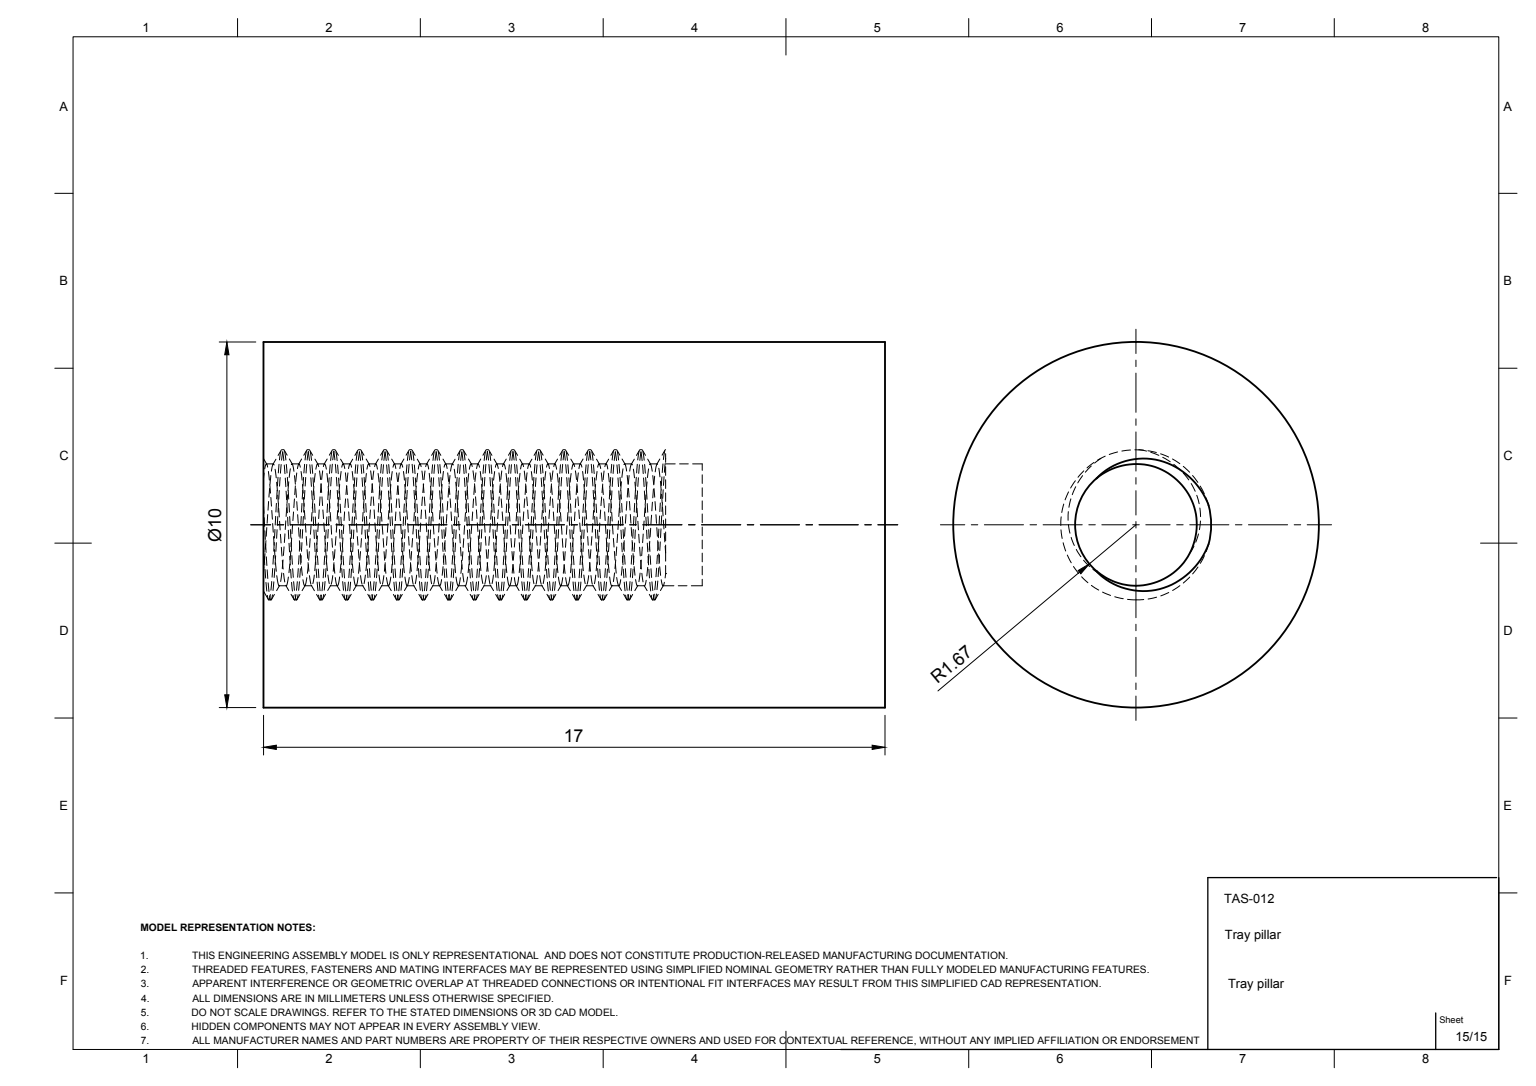
ISO-10303-21;
HEADER;
/* Generated by software containing ST-Developer
 * from STEP Tools, Inc. (www.steptools.com) 
 */

FILE_DESCRIPTION(
/* description */ (
'Independent welded steel electronics enclosure with removable sealed 
lid, internal mounting tray and two threaded cable entries. 300 x 220 
mm body. No ingress or electrical safety rating assigned.'),
/* implementation_level */ '2;1');

FILE_NAME(
/* name */ 'Tray pillar.step',
/* time_stamp */ '2026-11-14T09:13:27-08:00',
/* author */ (''),
/* organization */ (''),
/* preprocessor_version */ 'ST-DEVELOPER v20.2',
/* originating_system */ 'Autodesk Translation Framework v15.17.0.0',
/* authorisation */ '');

FILE_SCHEMA (('AUTOMOTIVE_DESIGN { 1 0 10303 214 3 1 1 }'));
ENDSEC;

DATA;
#10=MECHANICAL_DESIGN_GEOMETRIC_PRESENTATION_REPRESENTATION('',(#972),#94412);
#160=B_SPLINE_SURFACE_WITH_KNOTS('',3,3,((#58672,#58673,#58674,#58675,#58676,
#58677,#58678,#58679,#58680,#58681,#58682,#58683,#58684,#58685,#58686,#58687,
#58688,#58689,#58690,#58691,#58692,#58693,#58694,#58695,#58696,#58697,#58698,
#58699,#58700,#58701,#58702,#58703,#58704,#58705,#58706,#58707,#58708,#58709,
#58710,#58711,#58712,#58713,#58714,#58715,#58716,#58717,#58718,#58719,#58720,
#58721,#58722,#58723,#58724,#58725,#58726,#58727,#58728,#58729,#58730,#58731,
#58732,#58733,#58734,#58735,#58736,#58737,#58738,#58739,#58740,#58741,#58742,
#58743,#58744,#58745,#58746,#58747,#58748,#58749,#58750,#58751,#58752,#58753,
#58754,#58755,#58756,#58757,#58758,#58759,#58760,#58761,#58762,#58763,#58764,
#58765,#58766,#58767,#58768,#58769,#58770,#58771,#58772,#58773,#58774,#58775),
(#58776,#58777,#58778,#58779,#58780,#58781,#58782,#58783,#58784,#58785,
#58786,#58787,#58788,#58789,#58790,#58791,#58792,#58793,#58794,#58795,#58796,
#58797,#58798,#58799,#58800,#58801,#58802,#58803,#58804,#58805,#58806,#58807,
#58808,#58809,#58810,#58811,#58812,#58813,#58814,#58815,#58816,#58817,#58818,
#58819,#58820,#58821,#58822,#58823,#58824,#58825,#58826,#58827,#58828,#58829,
#58830,#58831,#58832,#58833,#58834,#58835,#58836,#58837,#58838,#58839,#58840,
#58841,#58842,#58843,#58844,#58845,#58846,#58847,#58848,#58849,#58850,#58851,
#58852,#58853,#58854,#58855,#58856,#58857,#58858,#58859,#58860,#58861,#58862,
#58863,#58864,#58865,#58866,#58867,#58868,#58869,#58870,#58871,#58872,#58873,
#58874,#58875,#58876,#58877,#58878,#58879),(#58880,#58881,#58882,#58883,
#58884,#58885,#58886,#58887,#58888,#58889,#58890,#58891,#58892,#58893,#58894,
#58895,#58896,#58897,#58898,#58899,#58900,#58901,#58902,#58903,#58904,#58905,
#58906,#58907,#58908,#58909,#58910,#58911,#58912,#58913,#58914,#58915,#58916,
#58917,#58918,#58919,#58920,#58921,#58922,#58923,#58924,#58925,#58926,#58927,
#58928,#58929,#58930,#58931,#58932,#58933,#58934,#58935,#58936,#58937,#58938,
#58939,#58940,#58941,#58942,#58943,#58944,#58945,#58946,#58947,#58948,#58949,
#58950,#58951,#58952,#58953,#58954,#58955,#58956,#58957,#58958,#58959,#58960,
#58961,#58962,#58963,#58964,#58965,#58966,#58967,#58968,#58969,#58970,#58971,
#58972,#58973,#58974,#58975,#58976,#58977,#58978,#58979,#58980,#58981,#58982,
#58983),(#58984,#58985,#58986,#58987,#58988,#58989,#58990,#58991,#58992,
#58993,#58994,#58995,#58996,#58997,#58998,#58999,#59000,#59001,#59002,#59003,
#59004,#59005,#59006,#59007,#59008,#59009,#59010,#59011,#59012,#59013,#59014,
#59015,#59016,#59017,#59018,#59019,#59020,#59021,#59022,#59023,#59024,#59025,
#59026,#59027,#59028,#59029,#59030,#59031,#59032,#59033,#59034,#59035,#59036,
#59037,#59038,#59039,#59040,#59041,#59042,#59043,#59044,#59045,#59046,#59047,
#59048,#59049,#59050,#59051,#59052,#59053,#59054,#59055,#59056,#59057,#59058,
#59059,#59060,#59061,#59062,#59063,#59064,#59065,#59066,#59067,#59068,#59069,
#59070,#59071,#59072,#59073,#59074,#59075,#59076,#59077,#59078,#59079,#59080,
#59081,#59082,#59083,#59084,#59085,#59086,#59087)),.UNSPECIFIED.,.F.,.F.,
 .F.,(4,4),(4,1,1,1,1,1,1,1,1,1,1,1,1,1,1,1,1,1,1,1,1,1,1,1,1,1,1,1,1,1,
1,1,1,1,1,1,1,1,1,1,1,1,1,1,1,1,1,1,1,1,1,1,1,1,1,1,1,1,1,1,1,1,1,1,1,1,
1,1,1,1,1,1,1,1,1,1,1,1,1,1,1,1,1,1,1,1,1,1,1,1,1,1,1,1,1,1,1,1,1,1,1,4),
(-0.000342905668100493,0.0451832374712266),(11.8612370985886,12.8591085386933,
13.8566370731299,14.8541656075665,15.8516941420031,16.8492226764397,17.8467512108763,
18.8442797453129,19.8418082797495,20.8393368141861,21.8368653486227,22.8343938830593,
23.8319224174959,24.8294509519325,25.8269794863691,26.8245080208057,27.8220365552423,
28.8195650896789,29.8170936241155,30.8146221585521,31.8121506929887,32.8096792274253,
33.8072077618619,34.8047362962985,35.8022648307351,36.7997933651717,37.7973218996083,
38.7948504340449,39.7923789684815,40.7899075029181,41.7874360373547,42.7849645717913,
43.7824931062279,44.7800216406645,45.7775501751011,46.7750787095377,47.7726072439743,
48.7701357784109,49.7676643128475,50.7651928472841,51.7627213817207,52.7602499161573,
53.7577784505939,54.7553069850305,55.7528355194671,56.7503640539037,57.7478925883403,
58.7454211227769,59.7429496572135,60.7404781916501,61.7380067260867,62.7355352605233,
63.7330637949599,64.7305923293965,65.7281208638331,66.7256493982697,67.7231779327063,
68.7207064671429,69.7182350015795,70.7157635360161,71.7132920704527,72.7108206048892,
73.7083491393258,74.7058776737625,75.7034062081991,76.7009347426357,77.6984632770722,
78.6959918115088,79.6935203459455,80.6910488803821,81.6885774148187,82.6861059492552,
83.6836344836918,84.6811630181284,85.678691552565,86.6762200870017,87.6737486214382,
88.6712771558748,89.6688056903114,90.666334224748,91.6638627591846,92.6613912936212,
93.6589198280578,94.6564483624944,95.653976896931,96.6515054313676,97.6490339658042,
98.6465625002408,99.6440910346774,100.641619569114,101.639148103551,102.636676637987,
103.634205172424,104.63173370686,105.629262241297,106.626790775734,107.62431931017,
108.621847844607,109.619376379043,110.61690491348,111.614433447917,112.611961982353),
 .UNSPECIFIED.);
#161=B_SPLINE_SURFACE_WITH_KNOTS('',3,3,((#59170,#59171,#59172,#59173,#59174,
#59175,#59176,#59177,#59178,#59179,#59180,#59181,#59182,#59183,#59184,#59185,
#59186,#59187,#59188,#59189,#59190,#59191,#59192,#59193,#59194,#59195,#59196,
#59197,#59198,#59199,#59200,#59201,#59202,#59203,#59204,#59205,#59206,#59207,
#59208,#59209,#59210,#59211,#59212,#59213,#59214,#59215,#59216,#59217,#59218,
#59219,#59220,#59221,#59222,#59223,#59224,#59225,#59226,#59227,#59228,#59229,
#59230,#59231,#59232,#59233,#59234,#59235,#59236,#59237,#59238,#59239,#59240,
#59241,#59242,#59243,#59244,#59245,#59246,#59247,#59248,#59249,#59250,#59251,
#59252,#59253,#59254,#59255,#59256,#59257,#59258,#59259,#59260,#59261,#59262,
#59263,#59264,#59265,#59266,#59267,#59268,#59269,#59270,#59271,#59272,#59273),
(#59274,#59275,#59276,#59277,#59278,#59279,#59280,#59281,#59282,#59283,
#59284,#59285,#59286,#59287,#59288,#59289,#59290,#59291,#59292,#59293,#59294,
#59295,#59296,#59297,#59298,#59299,#59300,#59301,#59302,#59303,#59304,#59305,
#59306,#59307,#59308,#59309,#59310,#59311,#59312,#59313,#59314,#59315,#59316,
#59317,#59318,#59319,#59320,#59321,#59322,#59323,#59324,#59325,#59326,#59327,
#59328,#59329,#59330,#59331,#59332,#59333,#59334,#59335,#59336,#59337,#59338,
#59339,#59340,#59341,#59342,#59343,#59344,#59345,#59346,#59347,#59348,#59349,
#59350,#59351,#59352,#59353,#59354,#59355,#59356,#59357,#59358,#59359,#59360,
#59361,#59362,#59363,#59364,#59365,#59366,#59367,#59368,#59369,#59370,#59371,
#59372,#59373,#59374,#59375,#59376,#59377),(#59378,#59379,#59380,#59381,
#59382,#59383,#59384,#59385,#59386,#59387,#59388,#59389,#59390,#59391,#59392,
#59393,#59394,#59395,#59396,#59397,#59398,#59399,#59400,#59401,#59402,#59403,
#59404,#59405,#59406,#59407,#59408,#59409,#59410,#59411,#59412,#59413,#59414,
#59415,#59416,#59417,#59418,#59419,#59420,#59421,#59422,#59423,#59424,#59425,
#59426,#59427,#59428,#59429,#59430,#59431,#59432,#59433,#59434,#59435,#59436,
#59437,#59438,#59439,#59440,#59441,#59442,#59443,#59444,#59445,#59446,#59447,
#59448,#59449,#59450,#59451,#59452,#59453,#59454,#59455,#59456,#59457,#59458,
#59459,#59460,#59461,#59462,#59463,#59464,#59465,#59466,#59467,#59468,#59469,
#59470,#59471,#59472,#59473,#59474,#59475,#59476,#59477,#59478,#59479,#59480,
#59481),(#59482,#59483,#59484,#59485,#59486,#59487,#59488,#59489,#59490,
#59491,#59492,#59493,#59494,#59495,#59496,#59497,#59498,#59499,#59500,#59501,
#59502,#59503,#59504,#59505,#59506,#59507,#59508,#59509,#59510,#59511,#59512,
#59513,#59514,#59515,#59516,#59517,#59518,#59519,#59520,#59521,#59522,#59523,
#59524,#59525,#59526,#59527,#59528,#59529,#59530,#59531,#59532,#59533,#59534,
#59535,#59536,#59537,#59538,#59539,#59540,#59541,#59542,#59543,#59544,#59545,
#59546,#59547,#59548,#59549,#59550,#59551,#59552,#59553,#59554,#59555,#59556,
#59557,#59558,#59559,#59560,#59561,#59562,#59563,#59564,#59565,#59566,#59567,
#59568,#59569,#59570,#59571,#59572,#59573,#59574,#59575,#59576,#59577,#59578,
#59579,#59580,#59581,#59582,#59583,#59584,#59585)),.UNSPECIFIED.,.F.,.F.,
 .F.,(4,4),(4,1,1,1,1,1,1,1,1,1,1,1,1,1,1,1,1,1,1,1,1,1,1,1,1,1,1,1,1,1,
1,1,1,1,1,1,1,1,1,1,1,1,1,1,1,1,1,1,1,1,1,1,1,1,1,1,1,1,1,1,1,1,1,1,1,1,
1,1,1,1,1,1,1,1,1,1,1,1,1,1,1,1,1,1,1,1,1,1,1,1,1,1,1,1,1,1,1,1,1,1,1,4),
(-0.000291827121531397,0.0452318691957662),(14.3981410127769,15.3956695472135,
16.3931980816501,17.3907266160867,18.3882551505233,19.3857836849599,20.3833122193965,
21.3808407538331,22.3783692882697,23.3758978227063,24.3734263571429,25.3709548915795,
26.3684834260161,27.3660119604527,28.3635404948893,29.3610690293259,30.3585975637625,
31.3561260981991,32.3536546326357,33.3511831670723,34.3487117015089,35.3462402359455,
36.3437687703821,37.3412973048187,38.3388258392553,39.3363543736919,40.3338829081285,
41.3314114425651,42.3289399770017,43.3264685114383,44.3239970458749,45.3215255803115,
46.3190541147481,47.3165826491847,48.3141111836213,49.3116397180579,50.3091682524945,
51.3066967869311,52.3042253213677,53.3017538558043,54.2992823902409,55.2968109246775,
56.2943394591141,57.2918679935507,58.2893965279873,59.2869250624239,60.2844535968605,
61.2819821312971,62.2795106657337,63.2770392001703,64.2745677346069,65.2720962690435,
66.2696248034801,67.2671533379167,68.2646818723533,69.2622104067899,70.2597389412265,
71.2572674756631,72.2547960100997,73.2523245445363,74.2498530789729,75.2473816134095,
76.2449101478461,77.2424386822827,78.2399672167193,79.2374957511559,80.2350242855925,
81.2325528200291,82.2300813544657,83.2276098889023,84.2251384233389,85.2226669577755,
86.2201954922121,87.2177240266487,88.2152525610853,89.2127810955219,90.2103096299585,
91.2078381643951,92.2053666988317,93.2028952332683,94.2004237677049,95.1979523021415,
96.1954808365781,97.1930093710147,98.1905379054513,99.1880664398879,100.185594974324,
101.183123508761,102.180652043198,103.178180577634,104.175709112071,105.173237646507,
106.170766180944,107.168294715381,108.165823249817,109.163351784254,110.16088031869,
111.158408853127,112.155937387564,113.153465922,114.150994456437,115.148865876639),
 .UNSPECIFIED.);
#538=B_SPLINE_CURVE_WITH_KNOTS('',3,(#48404,#48405,#48406,#48407),
 .UNSPECIFIED.,.F.,.F.,(4,4),(112.182457130247,112.611961982353),
 .UNSPECIFIED.);
#539=B_SPLINE_CURVE_WITH_KNOTS('',3,(#48410,#48411,#48412,#48413,#48414,
#48415,#48416,#48417,#48418,#48419,#48420,#48421,#48422,#48423,#48424,#48425,
#48426,#48427,#48428,#48429,#48430,#48431,#48432,#48433,#48434,#48435,#48436,
#48437,#48438,#48439,#48440),.UNSPECIFIED.,.F.,.F.,(4,3,3,3,3,3,3,3,3,3,
4),(112.181990371131,112.285911257127,112.391911114027,112.495583234741,
112.599202596607,112.702804270412,112.81058073089,112.914317775615,113.018127482769,
113.122103490096,113.133910112327),.UNSPECIFIED.);
#540=B_SPLINE_CURVE_WITH_KNOTS('',3,(#48446,#48447,#48448,#48449,#48450,
#48451,#48452,#48453,#48454,#48455,#48456,#48457,#48458,#48459,#48460,#48461,
#48462,#48463,#48464,#48465,#48466,#48467,#48468,#48469,#48470,#48471,#48472,
#48473,#48474,#48475,#48476,#48477,#48478,#48479,#48480,#48481,#48482,#48483,
#48484,#48485,#48486,#48487,#48488,#48489,#48490,#48491,#48492,#48493,#48494,
#48495,#48496,#48497,#48498,#48499,#48500,#48501,#48502,#48503,#48504,#48505,
#48506,#48507,#48508,#48509,#48510,#48511,#48512,#48513,#48514,#48515,#48516,
#48517,#48518,#48519,#48520,#48521,#48522,#48523,#48524,#48525,#48526,#48527,
#48528,#48529,#48530,#48531,#48532,#48533,#48534,#48535,#48536,#48537,#48538,
#48539,#48540,#48541,#48542,#48543,#48544,#48545,#48546,#48547,#48548,#48549,
#48550,#48551,#48552,#48553,#48554,#48555,#48556,#48557,#48558,#48559,#48560,
#48561,#48562,#48563,#48564,#48565,#48566),.UNSPECIFIED.,.F.,.F.,(4,3,3,
3,3,3,3,3,3,3,3,3,3,3,3,3,3,3,3,3,3,3,3,3,3,3,3,3,3,3,3,3,3,3,3,3,3,3,3,
3,4),(105.899155442176,106.00304508501,106.1068896956,106.210723989893,
106.314740686353,106.41871988312,106.522893881941,106.626790775734,106.731006157979,
106.835066684879,106.939005596441,107.042879290909,107.146722500751,107.250569915224,
107.354526007897,107.45854099524,107.562737655316,107.62431931017,107.728358547242,
107.832242196635,107.936003986749,108.03970049976,108.143366723004,108.247037600669,
108.350819047469,108.454660186161,108.558686145832,108.621847844607,108.726235019868,
108.830466334637,108.934573735116,109.038614403188,109.14262283246,109.246633471616,
109.350748646957,109.45492061008,109.559269251373,109.619376379043,109.74022388422,
109.860008885434,109.955742675385),.UNSPECIFIED.);
#541=B_SPLINE_CURVE_WITH_KNOTS('',3,(#48567,#48568,#48569,#48570,#48571,
#48572),.UNSPECIFIED.,.F.,.F.,(4,1,1,4),(109.955742875643,110.61690491348,
111.614433447917,112.182457130247),.UNSPECIFIED.);
#542=B_SPLINE_CURVE_WITH_KNOTS('',3,(#48574,#48575,#48576,#48577,#48578,
#48579,#48580,#48581,#48582,#48583,#48584,#48585,#48586,#48587,#48588,#48589,
#48590,#48591,#48592,#48593,#48594,#48595,#48596,#48597,#48598,#48599,#48600,
#48601,#48602,#48603,#48604,#48605,#48606,#48607,#48608,#48609,#48610,#48611,
#48612,#48613,#48614,#48615,#48616,#48617,#48618,#48619,#48620,#48621,#48622,
#48623,#48624,#48625,#48626,#48627,#48628,#48629,#48630,#48631,#48632,#48633,
#48634,#48635,#48636,#48637,#48638,#48639,#48640,#48641,#48642,#48643),
 .UNSPECIFIED.,.F.,.F.,(4,3,3,3,3,3,3,3,3,3,3,3,3,3,3,3,3,3,3,3,3,3,3,4),
(109.955742875643,110.103561930893,110.16088031869,110.264919435449,110.368802964289,
110.472564634045,110.576261026872,110.679927130268,110.783597888585,110.887379217594,
110.991220239184,111.095246084109,111.158408853127,111.262796080625,111.367027447102,
111.471134898278,111.575175616393,111.679184094987,111.783194782677,111.887310005039,
111.991482014394,112.0958307002,112.155937387564,112.181990371131),
 .UNSPECIFIED.);
#543=B_SPLINE_CURVE_WITH_KNOTS('',3,(#48644,#48645,#48646,#48647,#48648,
#48649,#48650,#48651),.UNSPECIFIED.,.F.,.F.,(4,1,1,1,1,4),(105.897706904075,
106.170766180944,107.168294715381,108.165823249817,109.163351784254,109.955739920457),
 .UNSPECIFIED.);
#544=B_SPLINE_CURVE_WITH_KNOTS('',3,(#48657,#48658,#48659,#48660,#48661,
#48662,#48663,#48664,#48665,#48666,#48667,#48668,#48669,#48670,#48671,#48672,
#48673,#48674,#48675,#48676,#48677,#48678,#48679,#48680,#48681,#48682,#48683,
#48684,#48685,#48686,#48687,#48688,#48689,#48690,#48691,#48692,#48693,#48694,
#48695,#48696,#48697,#48698,#48699,#48700,#48701,#48702,#48703,#48704,#48705,
#48706,#48707,#48708,#48709,#48710,#48711,#48712,#48713,#48714,#48715,#48716,
#48717,#48718,#48719,#48720,#48721,#48722,#48723,#48724,#48725,#48726,#48727,
#48728,#48729,#48730,#48731,#48732,#48733,#48734,#48735,#48736,#48737,#48738,
#48739,#48740,#48741,#48742,#48743,#48744,#48745,#48746,#48747,#48748,#48749,
#48750,#48751,#48752,#48753,#48754,#48755,#48756,#48757,#48758,#48759,#48760,
#48761,#48762,#48763,#48764,#48765,#48766,#48767,#48768,#48769,#48770,#48771,
#48772,#48773,#48774,#48775,#48776,#48777,#48778,#48779,#48780,#48781,#48782,
#48783),.UNSPECIFIED.,.F.,.F.,(4,3,3,3,3,3,3,3,3,3,3,3,3,3,3,3,3,3,3,3,
3,3,3,3,3,3,3,3,3,3,3,3,3,3,3,3,3,3,3,3,3,3,4),(99.6152477845043,99.6440910346774,
99.7482777229514,99.8523091754732,99.9562185935285,100.060062552649,100.163875831174,
100.267693164011,100.371619156583,100.475603988335,100.57977073543,100.641619569114,
100.745806998585,100.849839202802,100.95374938437,101.057594113864,101.161408168437,
101.265226281812,101.369153056302,101.473138671925,101.577306197386,101.639148103551,
101.743331447498,101.847359555346,101.951265644064,102.055106285069,102.158916261446,
102.262730312857,102.366653077886,102.470634707604,102.574798327491,102.636676637987,
102.740865744067,102.844899598207,102.94881138278,103.052657685547,103.156473281631,
103.260292902696,103.364221123497,103.468208153012,103.572377026272,103.634205172424,
103.672557568463),.UNSPECIFIED.);
#545=B_SPLINE_CURVE_WITH_KNOTS('',3,(#48784,#48785,#48786,#48787,#48788,
#48789,#48790,#48791,#48792,#48793,#48794,#48795,#48796,#48797,#48798,#48799,
#48800,#48801,#48802,#48803,#48804,#48805,#48806,#48807,#48808,#48809,#48810,
#48811,#48812,#48813,#48814,#48815,#48816,#48817,#48818,#48819,#48820,#48821,
#48822,#48823,#48824,#48825,#48826,#48827,#48828,#48829,#48830,#48831,#48832,
#48833,#48834,#48835,#48836,#48837,#48838,#48839,#48840,#48841,#48842,#48843,
#48844,#48845,#48846,#48847,#48848,#48849,#48850,#48851,#48852,#48853),
 .UNSPECIFIED.,.F.,.F.,(4,3,3,3,3,3,3,3,3,3,3,3,3,3,3,3,3,3,3,3,3,3,3,4),
(103.672557568731,103.776102954499,103.883056798544,103.98633119127,104.089546016561,
104.192736914806,104.295939489046,104.399253774652,104.502635390832,104.606186629628,
104.63173370686,104.735898602296,104.839908226138,104.943795866233,105.047618090183,
105.151409707593,105.255205484688,105.359110229006,105.463073953701,105.567220044936,
105.629262241297,105.733467137487,105.837506123452,105.899155442176),
 .UNSPECIFIED.);
#546=B_SPLINE_CURVE_WITH_KNOTS('',3,(#48855,#48856,#48857,#48858,#48859,
#48860),.UNSPECIFIED.,.F.,.F.,(4,1,1,4),(103.672557568463,104.175709112071,
105.173237646507,105.897706904075),.UNSPECIFIED.);
#547=B_SPLINE_CURVE_WITH_KNOTS('',3,(#48861,#48862,#48863,#48864,#48865,
#48866,#48867,#48868),.UNSPECIFIED.,.F.,.F.,(4,1,1,1,1,4),(99.6157845049343,
100.185594974324,101.183123508761,102.180652043198,103.178180577634,103.672557568463),
 .UNSPECIFIED.);
#548=B_SPLINE_CURVE_WITH_KNOTS('',3,(#48874,#48875,#48876,#48877,#48878,
#48879,#48880,#48881,#48882,#48883,#48884,#48885,#48886,#48887,#48888,#48889,
#48890,#48891,#48892,#48893,#48894,#48895,#48896,#48897,#48898,#48899,#48900,
#48901,#48902,#48903,#48904,#48905,#48906,#48907,#48908,#48909,#48910,#48911,
#48912,#48913,#48914,#48915,#48916,#48917,#48918,#48919,#48920,#48921,#48922,
#48923,#48924,#48925,#48926,#48927,#48928,#48929,#48930,#48931,#48932,#48933,
#48934,#48935,#48936,#48937,#48938,#48939,#48940,#48941,#48942,#48943,#48944,
#48945,#48946,#48947,#48948,#48949,#48950,#48951,#48952,#48953,#48954,#48955,
#48956,#48957,#48958,#48959,#48960,#48961,#48962,#48963,#48964,#48965,#48966,
#48967,#48968,#48969,#48970,#48971,#48972,#48973,#48974,#48975,#48976,#48977,
#48978,#48979,#48980,#48981,#48982,#48983,#48984,#48985,#48986,#48987,#48988,
#48989,#48990,#48991,#48992,#48993,#48994,#48995,#48996,#48997,#48998,#48999,
#49000),.UNSPECIFIED.,.F.,.F.,(4,3,3,3,3,3,3,3,3,3,3,3,3,3,3,3,3,3,3,3,
3,3,3,3,3,3,3,3,3,3,3,3,3,3,3,3,3,3,3,3,3,3,4),(93.3317577724807,93.4357061372678,
93.5397274007927,93.6439169172147,93.6589198280578,93.7631062477657,93.8671374348272,
93.9710465932312,94.0748902964138,94.178703323056,94.2825204084065,94.3864461618292,
94.4904307587697,94.5945972803976,94.6564483624944,94.7606348092475,94.8646660235604,
94.9685752093887,95.0724189400873,95.1762319942962,95.2800491072232,95.3839748880465,
95.4879595123299,95.5921260609117,95.653976896931,95.7581632576346,95.862194385787,
95.9661034856999,96.0699471306798,96.1737600994903,96.2775771274626,96.3815028245876,
96.4854873657548,96.5896538330368,96.6515054313676,96.7545601552911,96.8574737962598,
96.9602827783287,97.0675551490674,97.1702895580433,97.2730250439425,97.3758312784415,
97.3893722612836),.UNSPECIFIED.);
#549=B_SPLINE_CURVE_WITH_KNOTS('',3,(#49001,#49002,#49003,#49004,#49005,
#49006,#49007,#49008,#49009,#49010,#49011,#49012,#49013,#49014,#49015,#49016,
#49017,#49018,#49019,#49020,#49021,#49022,#49023,#49024,#49025,#49026,#49027,
#49028,#49029,#49030,#49031,#49032,#49033,#49034,#49035,#49036,#49037,#49038,
#49039,#49040,#49041,#49042,#49043,#49044,#49045,#49046,#49047,#49048,#49049,
#49050,#49051,#49052,#49053,#49054,#49055,#49056,#49057,#49058,#49059,#49060,
#49061,#49062,#49063,#49064,#49065,#49066,#49067),.UNSPECIFIED.,.F.,.F.,
(4,3,3,3,3,3,3,3,3,3,3,3,3,3,3,3,3,3,3,3,3,3,4),(97.3893722615972,97.522113023048,
97.6490339658042,97.753220555222,97.8572519130545,97.9611612429749,98.0650051180403,
98.1688183166771,98.2726355738801,98.3765614977545,98.4805462646138,98.5847129534722,
98.6465625002408,98.7507505133837,98.8588126722738,98.9627174078728,99.0665572074508,
99.1703668484503,99.274181065115,99.3780952818548,99.482069213541,99.5862024944616,
99.6152477845043),.UNSPECIFIED.);
#550=B_SPLINE_CURVE_WITH_KNOTS('',3,(#49069,#49070,#49071,#49072,#49073,
#49074),.UNSPECIFIED.,.F.,.F.,(4,1,1,4),(97.3893756995033,98.1905379054513,
99.1880664398879,99.6157845049343),.UNSPECIFIED.);
#551=B_SPLINE_CURVE_WITH_KNOTS('',3,(#49075,#49076,#49077,#49078,#49079,
#49080,#49081,#49082,#49083,#49084,#49085,#49086,#49087,#49088,#49089,#49090,
#49091,#49092,#49093,#49094,#49095,#49096,#49097,#49098,#49099,#49100,#49101,
#49102,#49103,#49104,#49105,#49106,#49107,#49108,#49109,#49110,#49111,#49112,
#49113,#49114,#49115,#49116,#49117,#49118,#49119,#49120,#49121,#49122,#49123,
#49124,#49125,#49126,#49127,#49128,#49129,#49130,#49131,#49132,#49133,#49134,
#49135,#49136,#49137,#49138,#49139,#49140,#49141,#49142,#49143,#49144,#49145,
#49146,#49147,#49148,#49149,#49150,#49151,#49152,#49153,#49154,#49155,#49156,
#49157,#49158,#49159,#49160,#49161,#49162,#49163,#49164,#49165,#49166,#49167,
#49168,#49169,#49170,#49171,#49172,#49173,#49174,#49175,#49176,#49177,#49178,
#49179,#49180,#49181,#49182,#49183,#49184,#49185,#49186,#49187,#49188,#49189,
#49190,#49191,#49192,#49193,#49194,#49195,#49196,#49197,#49198),
 .UNSPECIFIED.,.F.,.F.,(4,3,3,3,3,3,3,3,3,3,3,3,3,3,3,3,3,3,3,3,3,3,3,3,
3,3,3,3,3,3,3,3,3,3,3,3,3,3,3,3,3,4),(93.3327430891432,93.4412031739634,
93.5450898018628,93.6489210495062,93.7527316794015,93.856556420739,93.9604959875624,
94.0645034316264,94.1686838441858,94.2004237677049,94.304610191284,94.4086413823106,
94.5125505447987,94.6163942521362,94.7202072829974,94.8240243726246,94.9279501303813,
95.0319347316947,95.1361012577082,95.1979523021415,95.3021387136097,95.4061698925181,
95.5100790429346,95.6139227382356,95.7177357571129,95.8215528348257,95.9254785808556,
96.02946317053,96.1336296851692,96.1954808365781,96.2996672562813,96.403698443338,
96.507607601737,96.6114513049142,96.7152643315507,96.8190814168954,96.9230071703122,
97.0269917672468,97.1311582888685,97.1930093710147,97.3433995313053,97.3893722612836),
 .UNSPECIFIED.);
#552=B_SPLINE_CURVE_WITH_KNOTS('',3,(#49204,#49205,#49206,#49207,#49208,
#49209,#49210,#49211),.UNSPECIFIED.,.F.,.F.,(4,1,1,1,1,4),(87.0496595016183,
87.6737486214382,88.6712771558748,89.6688056903114,90.666334224748,91.1061824133145),
 .UNSPECIFIED.);
#553=B_SPLINE_CURVE_WITH_KNOTS('',3,(#49212,#49213,#49214,#49215,#49216,
#49217,#49218,#49219,#49220,#49221,#49222,#49223,#49224,#49225,#49226,#49227,
#49228,#49229,#49230,#49231,#49232,#49233,#49234,#49235,#49236,#49237,#49238,
#49239,#49240,#49241,#49242,#49243,#49244,#49245,#49246,#49247,#49248,#49249,
#49250,#49251,#49252,#49253,#49254,#49255,#49256,#49257,#49258,#49259,#49260,
#49261,#49262,#49263,#49264,#49265,#49266,#49267,#49268,#49269,#49270,#49271,
#49272,#49273,#49274,#49275,#49276,#49277,#49278,#49279,#49280,#49281),
 .UNSPECIFIED.,.F.,.F.,(4,3,3,3,3,3,3,3,3,3,3,3,3,3,3,3,3,3,3,3,3,3,3,4),
(91.106186954104,91.2126211244869,91.3191385189971,91.4258526613343,91.5326811144277,
91.6397297919096,91.6638627591846,91.7680491827495,91.872080373762,91.9759895362358,
92.0798332435591,92.1836462744062,92.2874633640191,92.3913891217618,92.4953737230612,
92.5995402490611,92.6613912936212,92.7655571697299,92.8695782280914,92.9734894823971,
93.0773351303294,93.1811423577143,93.2849756902826,93.3317577724807),
 .UNSPECIFIED.);
#554=B_SPLINE_CURVE_WITH_KNOTS('',3,(#49283,#49284,#49285,#49286,#49287,
#49288,#49289,#49290,#49291,#49292,#49293,#49294,#49295,#49296,#49297,#49298,
#49299,#49300,#49301,#49302,#49303,#49304,#49305,#49306,#49307,#49308,#49309,
#49310,#49311,#49312,#49313,#49314,#49315,#49316,#49317,#49318,#49319,#49320,
#49321,#49322,#49323,#49324,#49325,#49326,#49327,#49328,#49329,#49330,#49331,
#49332,#49333,#49334,#49335,#49336,#49337,#49338,#49339,#49340,#49341,#49342,
#49343,#49344,#49345,#49346,#49347,#49348,#49349,#49350,#49351,#49352),
 .UNSPECIFIED.,.F.,.F.,(4,3,3,3,3,3,3,3,3,3,3,3,3,3,3,3,3,3,3,3,3,3,3,4),
(91.106186954104,91.2078381643951,91.3120245843195,91.4160557716771,91.5199649304926,
91.6238086341573,91.7276216613509,91.8314387473207,91.9353645014613,92.0393490991763,
92.1435156216584,92.2053666988317,92.3095531170952,92.4135843027923,92.5174934599552,
92.6213371619734,92.7251501875286,92.8289672718709,92.9328930244111,93.0368776205386,
93.1410441414708,93.2028952332683,93.3070788384004,93.3327430891432),
 .UNSPECIFIED.);
#555=B_SPLINE_CURVE_WITH_KNOTS('',3,(#49353,#49354,#49355,#49356,#49357,
#49358,#49359,#49360,#49361,#49362,#49363,#49364,#49365,#49366,#49367,#49368,
#49369,#49370,#49371,#49372,#49373,#49374,#49375,#49376,#49377,#49378,#49379,
#49380,#49381,#49382,#49383,#49384,#49385,#49386,#49387,#49388,#49389,#49390,
#49391,#49392,#49393,#49394,#49395,#49396,#49397,#49398,#49399,#49400,#49401,
#49402,#49403,#49404,#49405,#49406,#49407,#49408,#49409,#49410,#49411,#49412,
#49413,#49414,#49415,#49416,#49417,#49418,#49419,#49420,#49421,#49422,#49423,
#49424,#49425,#49426,#49427,#49428,#49429,#49430,#49431,#49432,#49433,#49434,
#49435,#49436,#49437,#49438,#49439,#49440,#49441,#49442,#49443,#49444,#49445,
#49446,#49447,#49448,#49449,#49450,#49451,#49452,#49453,#49454,#49455,#49456,
#49457,#49458,#49459,#49460,#49461,#49462,#49463,#49464,#49465,#49466,#49467,
#49468,#49469,#49470,#49471,#49472,#49473,#49474,#49475,#49476),
 .UNSPECIFIED.,.F.,.F.,(4,3,3,3,3,3,3,3,3,3,3,3,3,3,3,3,3,3,3,3,3,3,3,3,
3,3,3,3,3,3,3,3,3,3,3,3,3,3,3,3,3,4),(87.0484659949012,87.1526312129392,
87.2177240266487,87.3219104458962,87.4259416325748,87.5298507907112,87.6336944936971,
87.7375075202133,87.8413246055082,87.9452503589819,88.0492349560335,88.1534014778652,
88.2152525610853,88.3194389804513,88.4234701672489,88.5273793255043,88.6312230286093,
88.7350360552444,88.8388531406578,88.9427788942487,89.0467634914171,89.1509300133632,
89.2127810955219,89.3169675146659,89.4209987012417,89.5249078592767,89.6287515621622,
89.7325645885791,89.8363816737758,89.940307427154,90.0442920241114,90.1484585458519,
90.2103096299585,90.3131827202774,90.4158805806228,90.5184806859093,90.6210195308692,
90.7235335246182,90.8261208446082,90.9287446851267,91.0315305432363,91.1061869536522),
 .UNSPECIFIED.);
#556=B_SPLINE_CURVE_WITH_KNOTS('',3,(#49482,#49483,#49484,#49485,#49486,
#49487,#49488,#49489,#49490,#49491,#49492,#49493,#49494,#49495,#49496,#49497,
#49498,#49499,#49500,#49501,#49502,#49503,#49504,#49505,#49506,#49507,#49508,
#49509,#49510,#49511,#49512,#49513,#49514,#49515,#49516,#49517,#49518,#49519,
#49520,#49521,#49522,#49523,#49524,#49525,#49526,#49527,#49528,#49529,#49530,
#49531,#49532,#49533,#49534,#49535,#49536,#49537,#49538,#49539,#49540,#49541,
#49542,#49543,#49544,#49545,#49546,#49547,#49548,#49549,#49550,#49551,#49552,
#49553,#49554,#49555,#49556,#49557,#49558,#49559,#49560,#49561,#49562,#49563,
#49564,#49565,#49566,#49567,#49568,#49569,#49570,#49571,#49572,#49573,#49574,
#49575,#49576,#49577,#49578,#49579,#49580,#49581,#49582,#49583,#49584,#49585,
#49586,#49587,#49588,#49589,#49590,#49591,#49592,#49593,#49594,#49595,#49596,
#49597,#49598,#49599,#49600,#49601,#49602),.UNSPECIFIED.,.F.,.F.,(4,3,3,
3,3,3,3,3,3,3,3,3,3,3,3,3,3,3,3,3,3,3,3,3,3,3,3,3,3,3,3,3,3,3,3,3,3,3,3,
3,4),(80.7662207640143,80.8702913123123,80.9742249190925,81.0780833656369,
81.1819014489876,81.2857139129852,81.3896288357873,81.4935939089057,81.5977500997127,
81.6885774148187,81.7927638340834,81.8967950207793,82.0007041789332,82.1045478819369,
82.2083609084708,82.3121779937836,82.4161037472752,82.5200883443447,82.6242548661941,
82.6861059492552,82.7902923685379,82.8943235552519,82.9982327134239,83.1020764164457,
83.2058894429977,83.3097065283284,83.4136322818377,83.517616878925,83.6217834007917,
83.6836344836918,83.7878209029459,83.8918520896312,83.9957612477749,84.0996049507683,
84.2034179772922,84.3072350625951,84.4111608160771,84.5151454131373,84.6193119349777,
84.6811630181284,84.8230016469244),.UNSPECIFIED.);
#557=B_SPLINE_CURVE_WITH_KNOTS('',3,(#49603,#49604,#49605,#49606,#49607,
#49608),.UNSPECIFIED.,.F.,.F.,(4,1,1,4),(84.8230094328245,85.678691552565,
86.6762200870017,87.0496595016183),.UNSPECIFIED.);
#558=B_SPLINE_CURVE_WITH_KNOTS('',3,(#49610,#49611,#49612,#49613,#49614,
#49615,#49616,#49617,#49618,#49619,#49620,#49621,#49622,#49623,#49624,#49625,
#49626,#49627,#49628,#49629,#49630,#49631,#49632,#49633,#49634,#49635,#49636,
#49637,#49638,#49639,#49640,#49641,#49642,#49643,#49644,#49645,#49646,#49647,
#49648,#49649,#49650,#49651,#49652,#49653,#49654,#49655,#49656,#49657,#49658,
#49659,#49660,#49661,#49662,#49663,#49664,#49665,#49666,#49667,#49668,#49669,
#49670,#49671,#49672,#49673,#49674,#49675,#49676),.UNSPECIFIED.,.F.,.F.,
(4,3,3,3,3,3,3,3,3,3,3,3,3,3,3,3,3,3,3,3,3,3,4),(84.8230020854923,84.9377584637952,
85.0529305011137,85.1686597771981,85.2226669577755,85.3268533770583,85.4308845637724,
85.5347937219446,85.6386374249663,85.7424504515183,85.8462675368491,85.9501932903585,
86.0541778874458,86.1583444093125,86.2201954922121,86.3243482544069,86.4283607931299,
86.5322681004129,86.6361050454483,86.7399459750719,86.843781441697,86.947723926167,
87.0484659949012),.UNSPECIFIED.);
#559=B_SPLINE_CURVE_WITH_KNOTS('',3,(#49677,#49678,#49679,#49680,#49681,
#49682,#49683,#49684),.UNSPECIFIED.,.F.,.F.,(4,1,1,1,1,4),(80.7656839778309,
81.2325528200291,82.2300813544657,83.2276098889023,84.2251384233389,84.8230016469244),
 .UNSPECIFIED.);
#560=B_SPLINE_CURVE_WITH_KNOTS('',3,(#49690,#49691,#49692,#49693,#49694,
#49695,#49696,#49697,#49698,#49699,#49700,#49701,#49702,#49703,#49704,#49705,
#49706,#49707,#49708,#49709,#49710,#49711,#49712,#49713,#49714,#49715,#49716,
#49717,#49718,#49719,#49720,#49721,#49722,#49723,#49724,#49725,#49726,#49727,
#49728,#49729,#49730,#49731,#49732,#49733,#49734,#49735,#49736,#49737,#49738,
#49739,#49740,#49741,#49742,#49743,#49744,#49745,#49746,#49747,#49748,#49749,
#49750,#49751,#49752,#49753,#49754,#49755,#49756,#49757,#49758,#49759,#49760,
#49761,#49762,#49763,#49764,#49765,#49766,#49767,#49768,#49769,#49770,#49771,
#49772,#49773,#49774,#49775,#49776,#49777,#49778,#49779,#49780,#49781,#49782,
#49783,#49784,#49785,#49786,#49787,#49788,#49789,#49790,#49791,#49792,#49793,
#49794,#49795,#49796,#49797,#49798,#49799,#49800,#49801,#49802,#49803,#49804,
#49805,#49806,#49807,#49808,#49809,#49810,#49811,#49812,#49813,#49814,#49815,
#49816),.UNSPECIFIED.,.F.,.F.,(4,3,3,3,3,3,3,3,3,3,3,3,3,3,3,3,3,3,3,3,
3,3,3,3,3,3,3,3,3,3,3,3,3,3,3,3,3,3,3,3,3,3,4),(74.4820777272201,74.5860984994285,
74.6902876866266,74.7058776737625,74.8100640930311,74.9140952797311,75.0180044378891,
75.1218481408968,75.2256611674348,75.3294782527517,75.4334040062473,75.5373886033209,
75.6415551251743,75.7034062081991,75.8075926274676,75.9116238141675,76.0155329723254,
76.1193766753329,76.2231897018708,76.3270067871875,76.430932540683,76.5349171377565,
76.6390836596097,76.7009347426357,76.8051211619046,76.9091523486048,77.0130615067631,
77.1169052097711,77.2207182363094,77.3245353216266,77.4284610751225,77.5324456721964,
77.63661219405,77.6984632770722,77.8036324098624,77.9060965907556,78.0084634414074,
78.1107696824831,78.2180313467107,78.3203753326952,78.4227592903825,78.5252692707006,
78.5398163393936),.UNSPECIFIED.);
#561=B_SPLINE_CURVE_WITH_KNOTS('',3,(#49817,#49818,#49819,#49820,#49821,
#49822,#49823,#49824,#49825,#49826,#49827,#49828,#49829,#49830,#49831,#49832,
#49833,#49834,#49835,#49836,#49837,#49838,#49839,#49840,#49841,#49842,#49843,
#49844,#49845,#49846,#49847,#49848,#49849,#49850,#49851,#49852,#49853,#49854,
#49855,#49856,#49857,#49858,#49859,#49860,#49861,#49862,#49863,#49864,#49865,
#49866,#49867,#49868,#49869,#49870,#49871,#49872,#49873,#49874,#49875,#49876,
#49877,#49878,#49879,#49880,#49881,#49882,#49883),.UNSPECIFIED.,.F.,.F.,
(4,3,3,3,3,3,3,3,3,3,3,3,3,3,3,3,3,3,3,3,3,3,4),(78.5398163397448,78.6959918115088,
78.8001782307767,78.904209417476,79.0081185756333,79.1119622786403,79.2157753051776,
79.3195923904937,79.4235181439887,79.5275027410616,79.6316692629143,79.6935203459455,
79.7977067652162,79.9017379519181,80.0056471100781,80.1094908130878,80.2133038396278,
80.3171209249467,80.4210466784442,80.5250312755198,80.629197797375,80.6910488803821,
80.7662207640143),.UNSPECIFIED.);
#562=B_SPLINE_CURVE_WITH_KNOTS('',3,(#49885,#49886,#49887,#49888,#49889,
#49890),.UNSPECIFIED.,.F.,.F.,(4,1,1,4),(78.5398163397448,79.2374957511559,
80.2350242855925,80.7656839778309),.UNSPECIFIED.);
#563=B_SPLINE_CURVE_WITH_KNOTS('',3,(#49891,#49892,#49893,#49894,#49895,
#49896,#49897,#49898,#49899,#49900,#49901,#49902,#49903,#49904,#49905,#49906,
#49907,#49908,#49909,#49910,#49911,#49912,#49913,#49914,#49915,#49916,#49917,
#49918,#49919,#49920,#49921,#49922,#49923,#49924,#49925,#49926,#49927,#49928,
#49929,#49930,#49931,#49932,#49933,#49934,#49935,#49936,#49937,#49938,#49939,
#49940,#49941,#49942,#49943,#49944,#49945,#49946,#49947,#49948,#49949,#49950,
#49951,#49952,#49953,#49954,#49955,#49956,#49957,#49958,#49959,#49960,#49961,
#49962,#49963,#49964,#49965,#49966,#49967,#49968,#49969,#49970,#49971,#49972,
#49973,#49974,#49975,#49976,#49977,#49978,#49979,#49980,#49981,#49982,#49983,
#49984,#49985,#49986,#49987,#49988,#49989,#49990,#49991,#49992,#49993,#49994,
#49995,#49996,#49997,#49998,#49999,#50000,#50001,#50002,#50003,#50004,#50005,
#50006,#50007,#50008,#50009,#50010,#50011,#50012,#50013,#50014),
 .UNSPECIFIED.,.F.,.F.,(4,3,3,3,3,3,3,3,3,3,3,3,3,3,3,3,3,3,3,3,3,3,3,3,
3,3,3,3,3,3,3,3,3,3,3,3,3,3,3,3,3,4),(74.483258856194,74.58714895619,74.6909820348205,
74.7947928570274,74.8986161527883,75.0025532911364,75.1065568345892,75.2107347646363,
75.2473816134095,75.3515680326781,75.4555992193779,75.5595083775358,75.6633520805436,
75.7671651070816,75.8709821923984,75.974907945894,76.0788925429675,76.1830590648209,
76.2449101478461,76.3490965671147,76.4531277538146,76.5570369119727,76.6608806149803,
76.7646936415184,76.8685107268353,76.9724364803309,77.0764210774048,77.1805875992581,
77.2424386822827,77.3466251015512,77.4506562882509,77.5545654464089,77.6584091494165,
77.7622221759546,77.8660392612716,77.9699650147671,78.0739496118409,78.1781161336942,
78.2399672167193,78.3667743019381,78.4918646593798,78.5398161595682),
 .UNSPECIFIED.);
#564=B_SPLINE_CURVE_WITH_KNOTS('',3,(#50020,#50021,#50022,#50023,#50024,
#50025,#50026,#50027),.UNSPECIFIED.,.F.,.F.,(4,1,1,1,1,4),(68.1996051490179,
68.7207064671429,69.7182350015795,70.7157635360161,71.7132920704527,72.2566310325652),
 .UNSPECIFIED.);
#565=B_SPLINE_CURVE_WITH_KNOTS('',3,(#50028,#50029,#50030,#50031,#50032,
#50033,#50034,#50035,#50036,#50037,#50038,#50039,#50040,#50041,#50042,#50043,
#50044,#50045,#50046,#50047,#50048,#50049,#50050,#50051,#50052,#50053,#50054,
#50055,#50056,#50057,#50058,#50059,#50060,#50061,#50062,#50063,#50064,#50065,
#50066,#50067,#50068,#50069,#50070,#50071,#50072,#50073,#50074,#50075,#50076,
#50077,#50078,#50079,#50080,#50081,#50082,#50083,#50084,#50085,#50086,#50087,
#50088,#50089,#50090,#50091,#50092,#50093,#50094),.UNSPECIFIED.,.F.,.F.,
(4,3,3,3,3,3,3,3,3,3,3,3,3,3,3,3,3,3,3,3,3,3,4),(72.2566312677228,72.3701786020144,
72.4815875706104,72.5962040877498,72.7108206048892,72.8150070241578,72.9190382108577,
73.0229473690157,73.1267910720234,73.2306040985615,73.3344211838783,73.438346937374,
73.5423315344476,73.646498056301,73.7083491393258,73.8125058078903,73.9165206668431,
74.0204287152825,74.1242648270253,74.228091613986,74.3319123109939,74.4358068237418,
74.4820777272201),.UNSPECIFIED.);
#566=B_SPLINE_CURVE_WITH_KNOTS('',3,(#50096,#50097,#50098,#50099,#50100,
#50101,#50102,#50103,#50104,#50105,#50106,#50107,#50108,#50109,#50110,#50111,
#50112,#50113,#50114,#50115,#50116,#50117,#50118,#50119,#50120,#50121,#50122,
#50123,#50124,#50125,#50126,#50127,#50128,#50129,#50130,#50131,#50132,#50133,
#50134,#50135,#50136,#50137,#50138,#50139,#50140,#50141,#50142,#50143,#50144,
#50145,#50146,#50147,#50148,#50149,#50150,#50151,#50152,#50153,#50154,#50155,
#50156,#50157,#50158,#50159,#50160,#50161,#50162,#50163,#50164,#50165),
 .UNSPECIFIED.,.F.,.F.,(4,3,3,3,3,3,3,3,3,3,3,3,3,3,3,3,3,3,3,3,3,3,3,4),
(72.2566310325652,72.3607828828408,72.4647795326403,72.5686542861374,72.6724637223968,
72.7762426721719,72.8800259229371,72.983917905017,73.0878690474533,73.1920015684938,
73.2523245445363,73.356510963805,73.4605421505049,73.564451308663,73.6682950116707,
73.7721080382088,73.8759251235256,73.9798508770212,74.0838354740948,74.1880019959481,
74.2498530789729,74.3540440432939,74.4580688811934,74.483258856194),
 .UNSPECIFIED.);
#567=B_SPLINE_CURVE_WITH_KNOTS('',3,(#50166,#50167,#50168,#50169,#50170,
#50171,#50172,#50173,#50174,#50175,#50176,#50177,#50178,#50179,#50180,#50181,
#50182,#50183,#50184,#50185,#50186,#50187,#50188,#50189,#50190,#50191,#50192,
#50193,#50194,#50195,#50196,#50197,#50198,#50199,#50200,#50201,#50202,#50203,
#50204,#50205,#50206,#50207,#50208,#50209,#50210,#50211,#50212,#50213,#50214,
#50215,#50216,#50217,#50218,#50219,#50220,#50221,#50222,#50223,#50224,#50225,
#50226,#50227,#50228,#50229,#50230,#50231,#50232,#50233,#50234,#50235,#50236,
#50237,#50238,#50239,#50240,#50241,#50242,#50243,#50244,#50245,#50246,#50247,
#50248,#50249,#50250,#50251,#50252,#50253,#50254,#50255,#50256,#50257,#50258,
#50259,#50260,#50261,#50262,#50263,#50264,#50265,#50266,#50267,#50268,#50269,
#50270,#50271,#50272,#50273,#50274,#50275,#50276,#50277,#50278,#50279,#50280,
#50281,#50282,#50283,#50284,#50285,#50286,#50287,#50288,#50289,#50290,#50291,
#50292),.UNSPECIFIED.,.F.,.F.,(4,3,3,3,3,3,3,3,3,3,3,3,3,3,3,3,3,3,3,3,
3,3,3,3,3,3,3,3,3,3,3,3,3,3,3,3,3,3,3,3,3,3,4),(68.1991556033306,68.2646818723533,
68.3688682916219,68.4728994783219,68.5768086364799,68.6806523394876,68.7844653660256,
68.8882824513425,68.9922082048381,69.0961928019117,69.2003593237651,69.2622104067899,
69.3663968260585,69.4704280127585,69.5743371709165,69.6781808739242,69.7819939004622,
69.885810985779,69.9897367392747,70.0937213363483,70.1978878582017,70.2597389412265,
70.3639253604952,70.4679565471951,70.5718657053531,70.6757094083608,70.7795224348989,
70.8833395202158,70.9872652737114,71.091249870785,71.1954163926384,71.2572674756631,
71.3614538949318,71.4654850816318,71.5693942397898,71.6732379427974,71.7770509693354,
71.8808680546522,71.9847938081478,72.0887784052214,72.1929449270748,72.2547960100997,
72.2566310321323),.UNSPECIFIED.);
#568=B_SPLINE_CURVE_WITH_KNOTS('',3,(#50298,#50299,#50300,#50301,#50302,
#50303,#50304,#50305,#50306,#50307,#50308,#50309,#50310,#50311,#50312,#50313,
#50314,#50315,#50316,#50317,#50318,#50319,#50320,#50321,#50322,#50323,#50324,
#50325,#50326,#50327,#50328,#50329,#50330,#50331,#50332,#50333,#50334,#50335,
#50336,#50337,#50338,#50339,#50340,#50341,#50342,#50343,#50344,#50345,#50346,
#50347,#50348,#50349,#50350,#50351,#50352,#50353,#50354,#50355,#50356,#50357,
#50358,#50359,#50360,#50361,#50362,#50363,#50364,#50365,#50366,#50367,#50368,
#50369,#50370,#50371,#50372,#50373,#50374,#50375,#50376,#50377,#50378,#50379,
#50380,#50381,#50382,#50383,#50384,#50385,#50386,#50387,#50388,#50389,#50390,
#50391,#50392,#50393,#50394,#50395,#50396,#50397,#50398,#50399,#50400,#50401,
#50402,#50403,#50404,#50405,#50406,#50407,#50408,#50409,#50410,#50411,#50412,
#50413,#50414,#50415,#50416,#50417,#50418),.UNSPECIFIED.,.F.,.F.,(4,3,3,
3,3,3,3,3,3,3,3,3,3,3,3,3,3,3,3,3,3,3,3,3,3,3,3,3,3,3,3,3,3,3,3,3,3,3,3,
3,4),(61.9168822289229,62.0208161626315,62.1246748131786,62.2284929778564,
62.3323054006316,62.4362202018145,62.5401850432597,62.6443411223858,62.7355352605233,
62.8397216797919,62.9437528664919,63.0476620246499,63.1515057276576,63.2553187541956,
63.3591358395125,63.4630615930081,63.5670461900817,63.6712127119351,63.7330637949599,
63.8372502142285,63.9412814009285,64.0451905590865,64.1490342620942,64.2528472886323,
64.356664373949,64.4605901274447,64.5645747245183,64.6687412463717,64.7305923293965,
64.8347787486652,64.9388099353651,65.0427190935231,65.1465627965308,65.2503758230688,
65.3541929083857,65.4581186618813,65.5621032589549,65.6662697808083,65.7281208638331,
65.8639211032556,65.9734456460794),.UNSPECIFIED.);
#569=B_SPLINE_CURVE_WITH_KNOTS('',3,(#50419,#50420,#50421,#50422,#50423,
#50424),.UNSPECIFIED.,.F.,.F.,(4,1,1,4),(65.9734457253856,66.7256493982697,
67.7231779327063,68.1996051490179),.UNSPECIFIED.);
#570=B_SPLINE_CURVE_WITH_KNOTS('',3,(#50426,#50427,#50428,#50429,#50430,
#50431,#50432,#50433,#50434,#50435,#50436,#50437,#50438,#50439,#50440,#50441,
#50442,#50443,#50444,#50445,#50446,#50447,#50448,#50449,#50450,#50451,#50452,
#50453,#50454,#50455,#50456,#50457,#50458,#50459,#50460,#50461,#50462,#50463,
#50464,#50465,#50466,#50467,#50468,#50469,#50470,#50471,#50472,#50473,#50474,
#50475,#50476,#50477,#50478,#50479,#50480,#50481,#50482,#50483,#50484,#50485,
#50486,#50487,#50488,#50489,#50490,#50491,#50492),.UNSPECIFIED.,.F.,.F.,
(4,3,3,3,3,3,3,3,3,3,3,3,3,3,3,3,3,3,3,3,3,3,4),(65.973445898234,66.098877789982,
66.2261301221736,66.2696248034801,66.3738112227488,66.4778424094487,66.5817515676067,
66.6855952706144,66.7894082971524,66.8932253824693,66.9971511359649,67.1011357330385,
67.2053022548919,67.2671533379167,67.371344420459,67.4753543177416,67.5792620003784,
67.6831023298771,67.7869100863057,67.8907809338262,67.9946786755476,68.0987368797689,
68.1991556033306),.UNSPECIFIED.);
#571=B_SPLINE_CURVE_WITH_KNOTS('',3,(#50493,#50494,#50495,#50496,#50497,
#50498,#50499,#50500),.UNSPECIFIED.,.F.,.F.,(4,1,1,1,1,4),(61.91564316731,
62.2795106657337,63.2770392001703,64.2745677346069,65.2720962690435,65.9734457253856),
 .UNSPECIFIED.);
#572=B_SPLINE_CURVE_WITH_KNOTS('',3,(#50506,#50507,#50508,#50509,#50510,
#50511,#50512,#50513,#50514,#50515,#50516,#50517,#50518,#50519,#50520,#50521,
#50522,#50523,#50524,#50525,#50526,#50527,#50528,#50529,#50530,#50531,#50532,
#50533,#50534,#50535,#50536,#50537,#50538,#50539,#50540,#50541,#50542,#50543,
#50544,#50545,#50546,#50547,#50548,#50549,#50550,#50551,#50552,#50553,#50554,
#50555,#50556,#50557,#50558,#50559,#50560,#50561,#50562,#50563,#50564,#50565,
#50566,#50567,#50568,#50569,#50570,#50571,#50572,#50573,#50574,#50575,#50576,
#50577,#50578,#50579,#50580,#50581,#50582,#50583,#50584,#50585,#50586,#50587,
#50588,#50589,#50590,#50591,#50592,#50593,#50594,#50595,#50596,#50597,#50598,
#50599,#50600,#50601,#50602,#50603,#50604,#50605,#50606,#50607,#50608,#50609,
#50610,#50611,#50612,#50613,#50614,#50615,#50616,#50617,#50618,#50619,#50620,
#50621,#50622,#50623,#50624,#50625,#50626,#50627,#50628,#50629,#50630,#50631,
#50632),.UNSPECIFIED.,.F.,.F.,(4,3,3,3,3,3,3,3,3,3,3,3,3,3,3,3,3,3,3,3,
3,3,3,3,3,3,3,3,3,3,3,3,3,3,3,3,3,3,3,3,3,3,4),(55.6326174533268,55.73680638972,
55.7528355194671,55.8570219387357,55.9610531254357,56.0649622835937,56.1688059866014,
56.2726190131394,56.3764360984563,56.4803618519519,56.5843464490255,56.6885129708789,
56.7503640539037,56.8545504731723,56.9585816598723,57.0624908180303,57.166334521038,
57.270147547576,57.3739646328929,57.4778903863885,57.5818749834621,57.6860415053155,
57.7478925883403,57.8520790076089,57.9561101943089,58.0600193524669,58.1638630554746,
58.2676760820126,58.3714931673294,58.475418920825,58.5794035178986,58.683570039752,
58.7454211227769,58.8487780338705,58.9539633318708,59.0570447634811,59.1600643665938,
59.2630580262842,59.3698586241814,59.4729706208906,59.5761501528133,59.6794897442538,
59.690260417873),.UNSPECIFIED.);
#573=B_SPLINE_CURVE_WITH_KNOTS('',3,(#50633,#50634,#50635,#50636,#50637,
#50638,#50639,#50640,#50641,#50642,#50643,#50644,#50645,#50646,#50647,#50648,
#50649,#50650,#50651,#50652,#50653,#50654,#50655,#50656,#50657,#50658,#50659,
#50660,#50661,#50662,#50663,#50664,#50665,#50666,#50667,#50668,#50669,#50670,
#50671,#50672,#50673,#50674,#50675,#50676,#50677,#50678,#50679,#50680,#50681,
#50682,#50683,#50684,#50685,#50686,#50687,#50688,#50689,#50690,#50691,#50692,
#50693,#50694,#50695,#50696,#50697,#50698,#50699,#50700,#50701,#50702),
 .UNSPECIFIED.,.F.,.F.,(4,3,3,3,3,3,3,3,3,3,3,3,3,3,3,3,3,3,3,3,3,3,3,4),
(59.690260418206,59.7429496572135,59.8471360764821,59.9511672631822,60.0550764213402,
60.1589201243479,60.2627331508859,60.3665502362027,60.4704759896983,60.574460586772,
60.6786271086253,60.7404781916501,60.8446646109187,60.9486957976187,61.0526049557767,
61.1564486587844,61.2602616853224,61.3640787706392,61.4680045241349,61.5719891212085,
61.6761556430618,61.7380067260867,61.842168294112,61.9168822289229),
 .UNSPECIFIED.);
#574=B_SPLINE_CURVE_WITH_KNOTS('',3,(#50704,#50705,#50706,#50707,#50708,
#50709),.UNSPECIFIED.,.F.,.F.,(4,1,1,4),(59.690260418206,60.2844535968605,
61.2819821312971,61.91564316731),.UNSPECIFIED.);
#575=B_SPLINE_CURVE_WITH_KNOTS('',3,(#50710,#50711,#50712,#50713,#50714,
#50715,#50716,#50717,#50718,#50719,#50720,#50721,#50722,#50723,#50724,#50725,
#50726,#50727,#50728,#50729,#50730,#50731,#50732,#50733,#50734,#50735,#50736,
#50737,#50738,#50739,#50740,#50741,#50742,#50743,#50744,#50745,#50746,#50747,
#50748,#50749,#50750,#50751,#50752,#50753,#50754,#50755,#50756,#50757,#50758,
#50759,#50760,#50761,#50762,#50763,#50764,#50765,#50766,#50767,#50768,#50769,
#50770,#50771,#50772,#50773,#50774,#50775,#50776,#50777,#50778,#50779,#50780,
#50781,#50782,#50783,#50784,#50785,#50786,#50787,#50788,#50789,#50790,#50791,
#50792,#50793,#50794,#50795,#50796,#50797,#50798,#50799,#50800,#50801,#50802,
#50803,#50804,#50805,#50806,#50807,#50808,#50809,#50810,#50811,#50812,#50813,
#50814,#50815,#50816,#50817,#50818,#50819,#50820,#50821,#50822,#50823,#50824,
#50825,#50826,#50827,#50828,#50829,#50830,#50831,#50832,#50833),
 .UNSPECIFIED.,.F.,.F.,(4,3,3,3,3,3,3,3,3,3,3,3,3,3,3,3,3,3,3,3,3,3,3,3,
3,3,3,3,3,3,3,3,3,3,3,3,3,3,3,3,3,4),(55.6335626494765,55.7373959362262,
55.8412067845232,55.9450299244374,56.0489667972699,56.1529699116885,56.2571475712116,
56.2943394591141,56.3985258783827,56.5025570650826,56.6064662232406,56.7103099262482,
56.8141229527862,56.9179400381028,57.0218657915985,57.1258503886722,57.2300169105256,
57.2918679935507,57.3960544128194,57.5000855995192,57.6039947576773,57.7078384606848,
57.8116514872228,57.9154685725394,58.019394326035,58.1233789231088,58.2275454449622,
58.2893965279873,58.3935829472557,58.4976141339561,58.6015232921141,58.7053669951219,
58.8091800216598,58.9129971069768,59.0169228604724,59.120907457546,59.2250739793994,
59.2869250624239,59.4023023751458,59.5173142795046,59.631721429585,59.6902599887701),
 .UNSPECIFIED.);
#576=B_SPLINE_CURVE_WITH_KNOTS('',3,(#50839,#50840,#50841,#50842,#50843,
#50844,#50845,#50846),.UNSPECIFIED.,.F.,.F.,(4,1,1,1,1,4),(49.3495089121257,
49.7676643128475,50.7651928472841,51.7627213817207,52.7602499161573,53.4070751110264),
 .UNSPECIFIED.);
#577=B_SPLINE_CURVE_WITH_KNOTS('',3,(#50847,#50848,#50849,#50850,#50851,
#50852,#50853,#50854,#50855,#50856,#50857,#50858,#50859,#50860,#50861,#50862,
#50863,#50864,#50865,#50866,#50867,#50868,#50869,#50870,#50871,#50872,#50873,
#50874,#50875,#50876,#50877,#50878,#50879,#50880,#50881,#50882,#50883,#50884,
#50885,#50886,#50887,#50888,#50889,#50890,#50891,#50892,#50893,#50894,#50895,
#50896,#50897,#50898,#50899,#50900,#50901,#50902,#50903,#50904,#50905,#50906,
#50907,#50908,#50909,#50910,#50911,#50912,#50913),.UNSPECIFIED.,.F.,.F.,
(4,3,3,3,3,3,3,3,3,3,3,3,3,3,3,3,3,3,3,3,3,3,4),(53.4070753517635,53.5260748736241,
53.6461598280863,53.7577784505939,53.8619648698625,53.9659960565623,54.0699052147203,
54.173748917728,54.277561944266,54.3813790295829,54.4853047830786,54.5892893801522,
54.6934559020056,54.7553069850305,54.8649707935675,54.9689754329642,55.0728781103241,
55.1767136856929,55.2805169373318,55.3843685433793,55.4882480448386,55.5922481426596,
55.6326174533268),.UNSPECIFIED.);
#578=B_SPLINE_CURVE_WITH_KNOTS('',3,(#50915,#50916,#50917,#50918,#50919,
#50920,#50921,#50922,#50923,#50924,#50925,#50926,#50927,#50928,#50929,#50930,
#50931,#50932,#50933,#50934,#50935,#50936,#50937,#50938,#50939,#50940,#50941,
#50942,#50943,#50944,#50945,#50946,#50947,#50948,#50949,#50950,#50951,#50952,
#50953,#50954,#50955,#50956,#50957,#50958,#50959,#50960,#50961,#50962,#50963,
#50964,#50965,#50966,#50967,#50968,#50969,#50970,#50971,#50972,#50973,#50974,
#50975,#50976,#50977,#50978,#50979,#50980,#50981,#50982,#50983,#50984),
 .UNSPECIFIED.,.F.,.F.,(4,3,3,3,3,3,3,3,3,3,3,3,3,3,3,3,3,3,3,3,3,3,3,4),
(53.4070751114733,53.5098558320602,53.612486311178,53.7150344153122,53.8175366234368,
53.920029348614,54.0226180274639,54.1252565130453,54.2280753277646,54.2992823902409,
54.4034688095096,54.5074999962095,54.6114091543675,54.7152528573752,54.8190658839133,
54.9228829692301,55.0268087227257,55.1307933197992,55.2349598416526,55.2968109246775,
55.4009764939796,55.505005930678,55.6089152639628,55.6335626494765),
 .UNSPECIFIED.);
#579=B_SPLINE_CURVE_WITH_KNOTS('',3,(#50985,#50986,#50987,#50988,#50989,
#50990,#50991,#50992,#50993,#50994,#50995,#50996,#50997,#50998,#50999,#51000,
#51001,#51002,#51003,#51004,#51005,#51006,#51007,#51008,#51009,#51010,#51011,
#51012,#51013,#51014,#51015,#51016,#51017,#51018,#51019,#51020,#51021,#51022,
#51023,#51024,#51025,#51026,#51027,#51028,#51029,#51030,#51031,#51032,#51033,
#51034,#51035,#51036,#51037,#51038,#51039,#51040,#51041,#51042,#51043,#51044,
#51045,#51046,#51047,#51048,#51049,#51050,#51051,#51052,#51053,#51054,#51055,
#51056,#51057,#51058,#51059,#51060,#51061,#51062,#51063,#51064,#51065,#51066,
#51067,#51068,#51069,#51070,#51071,#51072,#51073,#51074,#51075,#51076,#51077,
#51078,#51079,#51080,#51081,#51082,#51083,#51084,#51085,#51086,#51087,#51088,
#51089,#51090,#51091,#51092,#51093,#51094,#51095,#51096,#51097,#51098,#51099,
#51100,#51101,#51102,#51103,#51104,#51105,#51106,#51107,#51108),
 .UNSPECIFIED.,.F.,.F.,(4,3,3,3,3,3,3,3,3,3,3,3,3,3,3,3,3,3,3,3,3,3,3,3,
3,3,3,3,3,3,3,3,3,3,3,3,3,3,3,3,3,4),(49.3501402663156,49.4542648365893,
49.5611277635774,49.6650067633435,49.7688341253606,49.8726446068756,49.9817755182803,
50.0857237633826,50.1897448377912,50.2939342287898,50.3091682524945,50.413354671763,
50.5173858584629,50.6212950166208,50.7251387196283,50.8289517461662,50.932768831483,
51.0366945849785,51.140679182052,51.2448457039053,51.3066967869311,51.4108832061997,
51.5149143928997,51.6188235510577,51.7226672540654,51.8264802806034,51.9302973659203,
52.0342231194159,52.1382077164896,52.2423742383429,52.3042253213677,52.4084117406364,
52.5124429273364,52.6163520854945,52.7201957885022,52.8240088150403,52.9278259003571,
53.0317516538528,53.1357362509265,53.2399027727799,53.3017538558043,53.4070751110264),
 .UNSPECIFIED.);
#580=B_SPLINE_CURVE_WITH_KNOTS('',3,(#51114,#51115,#51116,#51117,#51118,
#51119,#51120,#51121,#51122,#51123,#51124,#51125,#51126,#51127,#51128,#51129,
#51130,#51131,#51132,#51133,#51134,#51135,#51136,#51137,#51138,#51139,#51140,
#51141,#51142,#51143,#51144,#51145,#51146,#51147,#51148,#51149,#51150,#51151,
#51152,#51153,#51154,#51155,#51156,#51157,#51158,#51159,#51160,#51161,#51162,
#51163,#51164,#51165,#51166,#51167,#51168,#51169,#51170,#51171,#51172,#51173,
#51174,#51175,#51176,#51177,#51178,#51179,#51180,#51181,#51182,#51183,#51184,
#51185,#51186,#51187,#51188,#51189,#51190,#51191,#51192,#51193,#51194,#51195,
#51196,#51197,#51198,#51199,#51200,#51201,#51202,#51203,#51204,#51205,#51206,
#51207,#51208,#51209,#51210,#51211,#51212,#51213,#51214,#51215,#51216,#51217,
#51218,#51219,#51220,#51221,#51222,#51223,#51224,#51225,#51226,#51227,#51228,
#51229,#51230,#51231,#51232,#51233,#51234),.UNSPECIFIED.,.F.,.F.,(4,3,3,
3,3,3,3,3,3,3,3,3,3,3,3,3,3,3,3,3,3,3,3,3,3,3,3,3,3,3,3,3,3,3,3,3,3,3,3,
3,4),(43.0672872443465,43.1711461664278,43.274964439754,43.3787768084601,
43.4826914487572,43.5866559831908,43.690811914766,43.7824931062279,43.8866795254984,
43.9907107122005,44.0946198703604,44.1984635733701,44.3022765999102,44.4060936852289,
44.5100194387266,44.6140040358023,44.7181705576576,44.7800216406645,44.8842080599324,
44.9882392466315,45.0921484047887,45.1959921077957,45.2998051343331,45.4036222196496,
45.5075479731445,45.6115325702172,45.7156990920699,45.7775501751011,45.8817365943696,
45.9857677810689,46.0896769392268,46.1935206422343,46.2973336687722,46.4011507540888,
46.5050765075843,46.6090611046576,46.7132276265108,46.7750787095377,46.8955468169138,
47.0149579018511,47.1238895638475),.UNSPECIFIED.);
#581=B_SPLINE_CURVE_WITH_KNOTS('',3,(#51235,#51236,#51237,#51238,#51239,
#51240),.UNSPECIFIED.,.F.,.F.,(4,1,1,4),(47.1238898038468,47.7726072439743,
48.7701357784109,49.3495089121257),.UNSPECIFIED.);
#582=B_SPLINE_CURVE_WITH_KNOTS('',3,(#51242,#51243,#51244,#51245,#51246,
#51247,#51248,#51249,#51250,#51251,#51252,#51253,#51254,#51255,#51256,#51257,
#51258,#51259,#51260,#51261,#51262,#51263,#51264,#51265,#51266,#51267,#51268,
#51269,#51270,#51271,#51272,#51273,#51274,#51275,#51276,#51277,#51278,#51279,
#51280,#51281,#51282,#51283,#51284,#51285,#51286,#51287,#51288,#51289,#51290,
#51291,#51292,#51293,#51294,#51295,#51296,#51297,#51298,#51299,#51300,#51301,
#51302,#51303,#51304,#51305,#51306,#51307,#51308,#51309,#51310,#51311),
 .UNSPECIFIED.,.F.,.F.,(4,3,3,3,3,3,3,3,3,3,3,3,3,3,3,3,3,3,3,3,3,3,3,4),
(47.1238898038468,47.2757519674286,47.3165826491847,47.4207690684526,47.524800255152,
47.6287094133093,47.7325531163163,47.8363661428537,47.9401832281699,48.0441089816649,
48.1480935787378,48.2522601005905,48.3141111836213,48.4182976028898,48.5223287895896,
48.6262379477475,48.7300816507551,48.8338946772929,48.9377117626097,49.0416375161052,
49.1456221131786,49.2497886350318,49.3116397180579,49.3501402663156),
 .UNSPECIFIED.);
#583=B_SPLINE_CURVE_WITH_KNOTS('',3,(#51312,#51313,#51314,#51315,#51316,
#51317,#51318,#51319),.UNSPECIFIED.,.F.,.F.,(4,1,1,1,1,4),(43.0658398005562,
43.3264685114383,44.3239970458749,45.3215255803115,46.3190541147481,47.1238860295235),
 .UNSPECIFIED.);
#584=B_SPLINE_CURVE_WITH_KNOTS('',3,(#51325,#51326,#51327,#51328,#51329,
#51330,#51331,#51332,#51333,#51334,#51335,#51336,#51337,#51338,#51339,#51340,
#51341,#51342,#51343,#51344,#51345,#51346,#51347,#51348,#51349,#51350,#51351,
#51352,#51353,#51354,#51355,#51356,#51357,#51358,#51359,#51360,#51361,#51362,
#51363,#51364,#51365,#51366,#51367,#51368,#51369,#51370,#51371,#51372,#51373,
#51374,#51375,#51376,#51377,#51378,#51379,#51380,#51381,#51382,#51383,#51384,
#51385,#51386,#51387,#51388,#51389,#51390,#51391,#51392,#51393,#51394,#51395,
#51396,#51397,#51398,#51399,#51400,#51401,#51402,#51403,#51404,#51405,#51406,
#51407,#51408,#51409,#51410,#51411,#51412,#51413,#51414,#51415,#51416,#51417,
#51418,#51419,#51420,#51421,#51422,#51423,#51424,#51425,#51426,#51427,#51428,
#51429,#51430,#51431,#51432,#51433,#51434,#51435,#51436,#51437,#51438,#51439,
#51440,#51441,#51442,#51443,#51444,#51445,#51446,#51447,#51448,#51449,#51450,
#51451),.UNSPECIFIED.,.F.,.F.,(4,3,3,3,3,3,3,3,3,3,3,3,3,3,3,3,3,3,3,3,
3,3,3,3,3,3,3,3,3,3,3,3,3,3,3,3,3,3,3,3,3,3,4),(36.7834620528982,36.7997933651717,
36.9039797843287,37.0080109709146,37.1119201289555,37.2157638318444,37.3195768582619,
37.4233939434569,37.5273196968292,37.6313042937785,37.7354708155074,37.7973218996083,
37.9015083189688,38.0055395057619,38.1094486640147,38.2132923671181,38.3171053937527,
38.4209224791667,38.5248482327598,38.6288328299312,38.7329993518819,38.7948504340449,
38.899036853292,39.0030680399703,39.1069771981065,39.2108209010924,39.3146339276087,
39.4184510129037,39.5223767663778,39.6263613634299,39.7305278852622,39.7923789684815,
39.8965653877372,40.0005965744239,40.1045057325683,40.2083494355621,40.3121624620861,
40.4159795473886,40.5199053008698,40.6238898979288,40.7280564197675,40.7899075029181,
40.8407044966672),.UNSPECIFIED.);
#585=B_SPLINE_CURVE_WITH_KNOTS('',3,(#51452,#51453,#51454,#51455,#51456,
#51457,#51458,#51459,#51460,#51461,#51462,#51463,#51464,#51465,#51466,#51467,
#51468,#51469,#51470,#51471,#51472,#51473,#51474,#51475,#51476,#51477,#51478,
#51479,#51480,#51481,#51482,#51483,#51484,#51485,#51486,#51487,#51488,#51489,
#51490,#51491,#51492,#51493,#51494,#51495,#51496,#51497,#51498,#51499,#51500,
#51501,#51502,#51503,#51504,#51505,#51506,#51507,#51508,#51509,#51510,#51511,
#51512,#51513,#51514,#51515,#51516,#51517,#51518,#51519,#51520,#51521),
 .UNSPECIFIED.,.F.,.F.,(4,3,3,3,3,3,3,3,3,3,3,3,3,3,3,3,3,3,3,3,3,3,3,4),
(40.8407044969988,40.9440672893101,41.0494883828156,41.1525861150597,41.2556259852456,
41.3586438439961,41.4658418923358,41.5689883265775,41.6722057013573,41.7755885097806,
41.7874360373547,41.8916224566194,41.9956536433155,42.0995628014695,42.2034065044732,
42.3072195310072,42.4110366163199,42.5149623698115,42.6189469668809,42.7231134887303,
42.7849645717913,42.8891423345831,42.9931552794839,43.0672872443465),
 .UNSPECIFIED.);
#586=B_SPLINE_CURVE_WITH_KNOTS('',3,(#51523,#51524,#51525,#51526,#51527,
#51528),.UNSPECIFIED.,.F.,.F.,(4,1,1,4),(40.8407051184979,41.3314114425651,
42.3289399770017,43.0658398005562),.UNSPECIFIED.);
#587=B_SPLINE_CURVE_WITH_KNOTS('',3,(#51529,#51530,#51531,#51532,#51533,
#51534,#51535,#51536,#51537,#51538,#51539,#51540,#51541,#51542,#51543,#51544,
#51545,#51546,#51547,#51548,#51549,#51550,#51551,#51552,#51553,#51554,#51555,
#51556,#51557,#51558,#51559,#51560,#51561,#51562,#51563,#51564,#51565,#51566,
#51567,#51568,#51569,#51570,#51571,#51572,#51573,#51574,#51575,#51576,#51577,
#51578,#51579,#51580,#51581,#51582,#51583,#51584,#51585,#51586,#51587,#51588,
#51589,#51590,#51591,#51592,#51593,#51594,#51595,#51596,#51597,#51598,#51599,
#51600,#51601,#51602,#51603,#51604,#51605,#51606,#51607,#51608,#51609,#51610,
#51611,#51612,#51613,#51614,#51615,#51616,#51617,#51618,#51619,#51620,#51621,
#51622,#51623,#51624,#51625,#51626,#51627,#51628,#51629,#51630,#51631,#51632,
#51633,#51634,#51635,#51636,#51637,#51638,#51639,#51640,#51641,#51642,#51643,
#51644,#51645,#51646,#51647,#51648,#51649,#51650,#51651,#51652),
 .UNSPECIFIED.,.F.,.F.,(4,3,3,3,3,3,3,3,3,3,3,3,3,3,3,3,3,3,3,3,3,3,3,3,
3,3,3,3,3,3,3,3,3,3,3,3,3,3,3,3,3,4),(36.7837376627694,36.887548540786,
36.9913715043335,37.0953080764532,37.1993107049402,37.303488058312,37.3412973048187,
37.4454837247122,37.5495149120458,37.6534240708478,37.7572677745056,37.8610808016985,
37.9648978876741,38.0688236418301,38.172808239566,38.2769747620775,38.3388258392553,
38.4430122584196,38.547043445015,38.6509526030691,38.7547963059732,38.8586093324081,
38.9624264176225,39.0663521710174,39.1703367679912,39.2745032897469,39.3363543736919,
39.4405407928485,39.544571979434,39.6484811374745,39.7523248403629,39.85613786678,
39.9599549519746,40.0638807053465,40.1678653022953,40.2720318240237,40.3338829081285,
40.4430298278223,40.5518710897036,40.6605292202185,40.7689635853024,40.8407044966672),
 .UNSPECIFIED.);
#588=B_SPLINE_CURVE_WITH_KNOTS('',3,(#51658,#51659,#51660,#51661,#51662,
#51663,#51664,#51665),.UNSPECIFIED.,.F.,.F.,(4,1,1,1,1,4),(30.4995607225879,
30.8146221585521,31.8121506929887,32.8096792274253,33.8072077618619,34.5575191894876),
 .UNSPECIFIED.);
#589=B_SPLINE_CURVE_WITH_KNOTS('',3,(#51666,#51667,#51668,#51669,#51670,
#51671,#51672,#51673,#51674,#51675,#51676,#51677,#51678,#51679,#51680,#51681,
#51682,#51683,#51684,#51685,#51686,#51687,#51688,#51689,#51690,#51691,#51692,
#51693,#51694,#51695,#51696,#51697,#51698,#51699,#51700,#51701,#51702,#51703,
#51704,#51705,#51706,#51707,#51708,#51709,#51710,#51711,#51712,#51713,#51714,
#51715,#51716,#51717,#51718,#51719,#51720,#51721,#51722,#51723,#51724,#51725,
#51726,#51727,#51728,#51729,#51730,#51731,#51732),.UNSPECIFIED.,.F.,.F.,
(4,3,3,3,3,3,3,3,3,3,3,3,3,3,3,3,3,3,3,3,3,3,4),(34.5575192801504,34.6928923433788,
34.8047362962985,34.9089227161898,35.0129539035213,35.116863062321,35.2207067659762,
35.3245197931666,35.4283368791399,35.5322626332934,35.6362472310269,35.7404137535359,
35.8022648307351,35.9064523898748,36.0104843838919,36.1143930799466,36.2182358499137,
36.3220474727609,36.4258626833867,36.5297810949895,36.6337581570599,36.7379046758095,
36.7834620528982),.UNSPECIFIED.);
#590=B_SPLINE_CURVE_WITH_KNOTS('',3,(#51734,#51735,#51736,#51737,#51738,
#51739,#51740,#51741,#51742,#51743,#51744,#51745,#51746,#51747,#51748,#51749,
#51750,#51751,#51752,#51753,#51754,#51755,#51756,#51757,#51758,#51759,#51760,
#51761,#51762,#51763,#51764,#51765,#51766,#51767,#51768,#51769,#51770,#51771,
#51772,#51773,#51774,#51775,#51776,#51777,#51778,#51779,#51780,#51781,#51782,
#51783,#51784,#51785,#51786,#51787,#51788,#51789,#51790,#51791,#51792,#51793,
#51794,#51795,#51796,#51797,#51798,#51799,#51800,#51801,#51802,#51803),
 .UNSPECIFIED.,.F.,.F.,(4,3,3,3,3,3,3,3,3,3,3,3,3,3,3,3,3,3,3,3,3,3,3,4),
(34.5575191899647,34.6600276259523,34.7624524502431,34.8648302680991,34.9671976162021,
35.0696598730461,35.1721712758146,35.2748625475711,35.3462402359455,35.4504266548286,
35.5544578411485,35.658366998936,35.7622107015796,35.8660237277603,35.9698408127272,
36.0737665658867,36.1777511626315,36.2819176841713,36.3437687703821,36.4479637269223,
36.5519784416308,36.6558896246249,36.75972644537,36.7837376627694),
 .UNSPECIFIED.);
#591=B_SPLINE_CURVE_WITH_KNOTS('',3,(#51804,#51805,#51806,#51807,#51808,
#51809,#51810,#51811,#51812,#51813,#51814,#51815,#51816,#51817,#51818,#51819,
#51820,#51821,#51822,#51823,#51824,#51825,#51826,#51827,#51828,#51829,#51830,
#51831,#51832,#51833,#51834,#51835,#51836,#51837,#51838,#51839,#51840,#51841,
#51842,#51843,#51844,#51845,#51846,#51847,#51848,#51849,#51850,#51851,#51852,
#51853,#51854,#51855,#51856,#51857,#51858,#51859,#51860,#51861,#51862,#51863,
#51864,#51865,#51866,#51867,#51868,#51869,#51870,#51871,#51872,#51873,#51874,
#51875,#51876,#51877,#51878,#51879,#51880,#51881,#51882,#51883,#51884,#51885,
#51886,#51887,#51888,#51889,#51890,#51891,#51892,#51893,#51894,#51895,#51896,
#51897,#51898,#51899,#51900,#51901,#51902,#51903,#51904,#51905,#51906,#51907,
#51908,#51909,#51910,#51911,#51912,#51913,#51914,#51915,#51916,#51917,#51918,
#51919,#51920,#51921,#51922,#51923,#51924,#51925,#51926,#51927),
 .UNSPECIFIED.,.F.,.F.,(4,3,3,3,3,3,3,3,3,3,3,3,3,3,3,3,3,3,3,3,3,3,3,3,
3,3,3,3,3,3,3,3,3,3,3,3,3,3,3,3,3,4),(30.5009126726331,30.6078143508288,
30.7116934740814,30.815520868173,30.9193312905574,31.0285299924679,31.1324780670269,
31.2364989095826,31.3406881250854,31.3561260981991,31.4603125441236,31.5643437578127,
31.6682529433233,31.7720966738931,31.8759097281617,31.9797268413366,32.0836526226934,
32.1876372476719,32.2918037971965,32.3536546326357,32.4578410516562,32.5618722381836,
32.6657813962831,32.769625099303,32.8734381259239,32.9772552113946,33.0811809651525,
33.1851655625499,33.2893320848217,33.3511831670723,33.4553695791772,33.5594007585792,
33.6633099092749,33.7671536047227,33.8709666236145,33.9747837012098,34.0787094469216,
34.1826940361645,34.2868605501974,34.3487117015089,34.4945927786811,34.5575191894876),
 .UNSPECIFIED.);
#592=B_SPLINE_CURVE_WITH_KNOTS('',3,(#51933,#51934,#51935,#51936,#51937,
#51938,#51939,#51940),.UNSPECIFIED.,.F.,.F.,(4,1,1,1,1,4),(24.2177548267501,
24.8294509519325,25.8269794863691,26.8245080208057,27.8220365552423,28.274333882308),
 .UNSPECIFIED.);
#593=B_SPLINE_CURVE_WITH_KNOTS('',3,(#51941,#51942,#51943,#51944,#51945,
#51946),.UNSPECIFIED.,.F.,.F.,(4,1,1,4),(28.274333882308,28.8195650896789,
29.8170936241155,30.4995607225879),.UNSPECIFIED.);
#594=B_SPLINE_CURVE_WITH_KNOTS('',3,(#51948,#51949,#51950,#51951,#51952,
#51953,#51954,#51955,#51956,#51957,#51958,#51959,#51960,#51961,#51962,#51963,
#51964,#51965,#51966,#51967,#51968,#51969,#51970,#51971,#51972,#51973,#51974,
#51975,#51976,#51977,#51978,#51979,#51980,#51981,#51982,#51983,#51984,#51985,
#51986,#51987,#51988,#51989,#51990,#51991,#51992,#51993,#51994,#51995,#51996,
#51997,#51998,#51999,#52000,#52001,#52002,#52003,#52004,#52005,#52006,#52007,
#52008,#52009,#52010,#52011,#52012,#52013,#52014,#52015,#52016,#52017),
 .UNSPECIFIED.,.F.,.F.,(4,3,3,3,3,3,3,3,3,3,3,3,3,3,3,3,3,3,3,3,3,3,3,4),
(28.2743338823081,28.3635404948893,28.4677270806907,28.5717584358195,28.6756677644013,
28.779511638971,28.883324837953,28.9871420963408,29.0910680226713,29.1950527927073,
29.2992194858461,29.3610690293259,29.4652554639064,29.569286666705,29.6731958420586,
29.777039562931,29.8808526079774,29.984669712422,30.0885954858662,30.1925801033819,
30.2967466462425,30.3585975637625,30.4627747018241,30.5009126726331),
 .UNSPECIFIED.);
#595=B_SPLINE_CURVE_WITH_KNOTS('',3,(#52018,#52019,#52020,#52021,#52022,
#52023,#52024,#52025),.UNSPECIFIED.,.F.,.F.,(4,1,1,1,1,4),(24.2163931842857,
24.3734263571429,25.3709548915795,26.3684834260161,27.3660119604527,28.2743252313376),
 .UNSPECIFIED.);
#596=B_SPLINE_CURVE_WITH_KNOTS('',3,(#52031,#52032,#52033,#52034,#52035,
#52036),.UNSPECIFIED.,.F.,.F.,(4,1,1,4),(15.7079632679489,16.3931980816501,
17.3907266160867,17.9337012577548),.UNSPECIFIED.);
#597=B_SPLINE_CURVE_WITH_KNOTS('',3,(#52038,#52039,#52040,#52041,#52042),
 .UNSPECIFIED.,.F.,.F.,(4,1,4),(14.3981410127769,15.3956695472135,15.7079632679489),
 .UNSPECIFIED.);
#598=B_SPLINE_CURVE_WITH_KNOTS('',3,(#52046,#52047,#52048,#52049,#52050,
#52051,#52052,#52053,#52054,#52055,#52056,#52057,#52058,#52059,#52060,#52061,
#52062,#52063,#52064,#52065,#52066,#52067,#52068,#52069,#52070,#52071,#52072,
#52073,#52074,#52075,#52076,#52077,#52078,#52079,#52080,#52081,#52082,#52083,
#52084,#52085,#52086,#52087,#52088,#52089,#52090,#52091,#52092,#52093,#52094,
#52095,#52096,#52097,#52098,#52099,#52100,#52101,#52102,#52103),
 .UNSPECIFIED.,.F.,.F.,(4,3,3,3,3,3,3,3,3,3,3,3,3,3,3,3,3,3,3,4),(13.8761928828999,
13.9801649720632,14.0894150515011,14.1931072386484,14.296736927948,14.4003392051333,
14.5039491154842,14.6076671378982,14.7114479052023,14.8153999666522,14.8541656075665,
14.9608903151143,15.0635176111712,15.1660512775799,15.2685278719585,15.3709838699761,
15.4735074808561,15.5760720021476,15.6787728795733,15.7079632679489),
 .UNSPECIFIED.);
#599=B_SPLINE_CURVE_WITH_KNOTS('',3,(#52104,#52105,#52106,#52107,#52108,
#52109,#52110),.UNSPECIFIED.,.F.,.F.,(4,1,1,1,4),(15.7079632679489,15.8516941420031,
16.8492226764397,17.8467512108763,17.9345079337947),.UNSPECIFIED.);
#600=B_SPLINE_CURVE_WITH_KNOTS('',3,(#52116,#52117,#52118,#52119,#52120,
#52121,#52122,#52123,#52124,#52125,#52126,#52127,#52128,#52129,#52130,#52131,
#52132,#52133,#52134,#52135,#52136,#52137,#52138,#52139,#52140,#52141,#52142,
#52143,#52144,#52145,#52146,#52147,#52148,#52149,#52150,#52151,#52152,#52153,
#52154,#52155,#52156,#52157,#52158,#52159,#52160,#52161,#52162,#52163,#52164,
#52165,#52166,#52167,#52168,#52169,#52170,#52171,#52172,#52173,#52174,#52175,
#52176,#52177,#52178,#52179,#52180,#52181,#52182,#52183,#52184,#52185,#52186,
#52187,#52188,#52189,#52190,#52191,#52192,#52193,#52194,#52195,#52196,#52197,
#52198,#52199,#52200,#52201,#52202,#52203,#52204,#52205,#52206,#52207,#52208,
#52209,#52210,#52211,#52212,#52213,#52214,#52215,#52216,#52217,#52218,#52219,
#52220,#52221,#52222,#52223,#52224,#52225,#52226,#52227,#52228,#52229,#52230,
#52231,#52232,#52233,#52234,#52235,#52236,#52237,#52238,#52239,#52240,#52241,
#52242,#52243,#52244,#52245,#52246,#52247,#52248,#52249,#52250,#52251),
 .UNSPECIFIED.,.F.,.F.,(4,3,3,3,3,3,3,3,3,3,3,3,3,3,3,3,3,3,3,3,3,3,3,3,
3,3,3,3,3,3,3,3,3,3,3,3,3,3,3,3,3,3,3,3,3,4),(95.9108836822778,96.0202873100601,
96.1295970836597,96.2388539961436,96.3480989644021,96.4574524049631,96.5668605200234,
96.6764760888946,96.7602678403501,96.870274343827,96.981214597697,97.0909160403511,
97.2005489408146,97.3101536583972,97.4220643374946,97.5318017309419,97.6447990528643,
97.7577963747867,97.8677427759327,97.978690542594,98.088340801476,98.1979259593122,
98.3074864207066,98.4194460428358,98.529148157587,98.6422365334051,98.7553249092233,
98.863931659696,98.9750468826915,99.0833537633358,99.1915974508863,99.2998202680834,
99.4130785619775,99.5214671674737,99.6299441469002,99.7386243094718,99.7528534436599,
99.8657192639262,99.9783447484258,100.090828298591,100.203203130945,100.315502311895,
100.42779296924,100.54006917202,100.652430269464,100.750381978097),
 .UNSPECIFIED.);
#601=B_SPLINE_CURVE_WITH_KNOTS('',3,(#52255,#52256,#52257,#52258,#52259,
#52260,#52261,#52262,#52263,#52264),.UNSPECIFIED.,.F.,.F.,(4,3,3,4),(-98.7357640758916,
-98.6263458761001,-98.5171144442792,-98.4464074264151),.UNSPECIFIED.);
#602=B_SPLINE_CURVE_WITH_KNOTS('',3,(#52269,#52270,#52271,#52272,#52273,
#52274,#52275,#52276,#52277,#52278,#52279,#52280,#52281),.UNSPECIFIED.,
 .F.,.F.,(4,3,3,3,4),(-98.4464074264151,-98.3373449196508,-98.228335758133,
-98.1193172715618,-98.094162871386),.UNSPECIFIED.);
#603=B_SPLINE_CURVE_WITH_KNOTS('',3,(#52282,#52283,#52284,#52285,#52286,
#52287,#52288,#52289,#52290,#52291,#52292,#52293,#52294,#52295,#52296,#52297,
#52298,#52299,#52300,#52301,#52302,#52303,#52304,#52305,#52306,#52307,#52308,
#52309,#52310,#52311,#52312,#52313,#52314,#52315,#52316,#52317,#52318,#52319,
#52320,#52321,#52322,#52323,#52324,#52325,#52326,#52327,#52328,#52329,#52330,
#52331,#52332,#52333,#52334,#52335,#52336,#52337,#52338,#52339,#52340,#52341,
#52342,#52343,#52344,#52345,#52346,#52347,#52348,#52349,#52350,#52351,#52352,
#52353,#52354,#52355,#52356,#52357,#52358,#52359,#52360,#52361,#52362,#52363,
#52364,#52365,#52366,#52367,#52368,#52369,#52370,#52371,#52372,#52373,#52374,
#52375,#52376,#52377,#52378,#52379,#52380,#52381,#52382,#52383,#52384,#52385,
#52386,#52387,#52388,#52389,#52390,#52391,#52392,#52393,#52394,#52395,#52396,
#52397,#52398,#52399,#52400,#52401,#52402,#52403,#52404,#52405,#52406,#52407,
#52408,#52409,#52410,#52411,#52412,#52413,#52414,#52415,#52416,#52417,#52418,
#52419,#52420,#52421,#52422,#52423,#52424,#52425,#52426,#52427,#52428,#52429,
#52430,#52431,#52432,#52433,#52434,#52435,#52436,#52437,#52438,#52439,#52440,
#52441,#52442,#52443,#52444),.UNSPECIFIED.,.F.,.F.,(4,3,3,3,3,3,3,3,3,3,
3,3,3,3,3,3,3,3,3,3,3,3,3,3,3,3,3,3,3,3,3,3,3,3,3,3,3,3,3,3,3,3,3,3,3,3,
3,3,3,3,3,3,3,3,4),(-98.0941628710682,-97.96814081787,-97.8409325597495,
-97.7577963747867,-97.6478110000828,-97.5368681051162,-97.4271754338014,
-97.3175466708406,-97.2079414641239,-97.0960230581805,-96.9862737960981,
-96.8732708182241,-96.7602678403501,-96.6506201762776,-96.5396350674821,
-96.4302948044108,-96.3210229586511,-96.2117785902267,-96.0995187691484,
-95.9901358924464,-95.8764375991799,-95.7627393059135,-95.6529127814426,
-95.5419500301969,-95.4324257238689,-95.3229684069732,-95.2135374400353,
-95.1014557728957,-94.991885638747,-94.8785482051119,-94.7652107714769,
-94.6553934240873,-94.5444295257064,-94.4349133954284,-94.3254638552065,
-94.2160402511401,-94.1039507476152,-93.9943868569596,-93.881034547,-93.7676822370403,
-93.6579087468788,-93.5469393663444,-93.4374690990798,-93.3280660442032,
-93.2186894719818,-93.1065555296373,-92.9970394857318,-92.8835965941678,
-92.7701537026037,-92.6610396721199,-92.5520859975439,-92.4432521481903,
-92.3344888111749,-92.2257252315868,-92.1641970933112),.UNSPECIFIED.);
#604=B_SPLINE_CURVE_WITH_KNOTS('',3,(#52450,#52451,#52452,#52453,#52454,
#52455,#52456,#52457,#52458,#52459,#52460,#52461,#52462,#52463,#52464,#52465,
#52466,#52467,#52468,#52469,#52470,#52471,#52472,#52473,#52474,#52475,#52476,
#52477,#52478,#52479,#52480,#52481,#52482,#52483,#52484,#52485,#52486,#52487,
#52488,#52489,#52490,#52491,#52492,#52493,#52494,#52495,#52496,#52497,#52498,
#52499,#52500,#52501,#52502,#52503,#52504,#52505,#52506,#52507,#52508,#52509,
#52510,#52511,#52512,#52513,#52514,#52515,#52516,#52517,#52518,#52519,#52520,
#52521,#52522,#52523,#52524,#52525,#52526,#52527,#52528,#52529,#52530,#52531,
#52532,#52533,#52534,#52535,#52536,#52537,#52538,#52539,#52540,#52541,#52542,
#52543,#52544,#52545,#52546,#52547,#52548,#52549,#52550,#52551,#52552,#52553,
#52554,#52555,#52556,#52557,#52558,#52559,#52560,#52561,#52562,#52563,#52564,
#52565,#52566,#52567,#52568,#52569,#52570,#52571,#52572,#52573,#52574,#52575,
#52576,#52577,#52578,#52579,#52580,#52581,#52582,#52583,#52584,#52585,#52586,
#52587,#52588,#52589,#52590,#52591,#52592,#52593,#52594,#52595,#52596,#52597,
#52598,#52599,#52600,#52601,#52602,#52603,#52604,#52605,#52606,#52607,#52608,
#52609,#52610,#52611,#52612,#52613,#52614,#52615),.UNSPECIFIED.,.F.,.F.,
(4,3,3,3,3,3,3,3,3,3,3,3,3,3,3,3,3,3,3,3,3,3,3,3,3,3,3,3,3,3,3,3,3,3,3,
3,3,3,3,3,3,3,3,3,3,3,3,3,3,3,3,3,3,3,3,4),(89.6265168405702,89.7416999786078,
89.7775680992939,89.8873597387442,89.9983268506175,90.1078160365984,90.2172382449346,
90.326634173892,90.4387497888516,90.5482854700897,90.6616910519101,90.7750966337305,
90.8848943530555,90.9958607049444,91.1053559024537,91.2147840805338,91.3241859281211,
91.4362957381326,91.5458371451358,91.6592311566515,91.7726251681671,91.8824260289159,
91.9933919881269,92.1028905104742,92.2123220720462,92.3217273557269,92.4338339424461,
92.5433788739247,92.6567662882642,92.7701537026037,92.8799258782005,92.9908954230555,
93.1003651299235,93.2097679068537,93.3191444831736,93.4312789216403,93.5407956652934,
93.6542389511669,93.7676822370403,93.8775024156856,93.9884659601595,94.0979832706209,
94.2074333726056,94.3168569209728,94.4289453835988,94.538507696895,94.651859234186,
94.7652107714769,94.8734085310505,94.9814556744687,95.089395275171,95.1972702333879,
95.305166435024,95.4130758431646,95.5210990899593,95.5576018624958),
 .UNSPECIFIED.);
#605=B_SPLINE_CURVE_WITH_KNOTS('',3,(#52616,#52617,#52618,#52619,#52620,
#52621,#52622,#52623,#52624,#52625,#52626,#52627,#52628),.UNSPECIFIED.,
 .F.,.F.,(4,3,3,3,4),(95.5576018628657,95.7133781757262,95.7627393059135,
95.8723662565049,95.9108836822778),.UNSPECIFIED.);
#606=B_SPLINE_CURVE_WITH_KNOTS('',3,(#52630,#52631,#52632,#52633,#52634,
#52635,#52636,#52637,#52638,#52639,#52640,#52641,#52642),.UNSPECIFIED.,
 .F.,.F.,(4,3,3,3,4),(-92.1641970933112,-92.0553357947036,-91.9464069945238,
-91.8372961626777,-91.8109778956704),.UNSPECIFIED.);
#607=B_SPLINE_CURVE_WITH_KNOTS('',3,(#52643,#52644,#52645,#52646,#52647,
#52648,#52649,#52650,#52651,#52652),.UNSPECIFIED.,.F.,.F.,(4,1,1,1,1,1,
1,4),(-91.8109775642065,-91.7726251681671,-90.7750966337305,-89.7775680992939,
-88.7800395648573,-87.7825110304207,-86.7849824959841,-85.8810642303289),
 .UNSPECIFIED.);
#608=B_SPLINE_CURVE_WITH_KNOTS('',3,(#52658,#52659,#52660,#52661,#52662,
#52663,#52664,#52665,#52666,#52667,#52668,#52669,#52670,#52671,#52672,#52673,
#52674,#52675,#52676,#52677,#52678,#52679,#52680,#52681,#52682,#52683,#52684,
#52685,#52686,#52687,#52688,#52689,#52690,#52691,#52692,#52693,#52694,#52695,
#52696,#52697,#52698,#52699,#52700,#52701,#52702,#52703,#52704,#52705,#52706,
#52707,#52708,#52709,#52710,#52711,#52712,#52713,#52714,#52715,#52716,#52717,
#52718,#52719,#52720,#52721,#52722,#52723,#52724,#52725,#52726,#52727,#52728,
#52729,#52730,#52731,#52732,#52733,#52734,#52735,#52736,#52737,#52738,#52739,
#52740,#52741,#52742,#52743,#52744,#52745,#52746,#52747,#52748,#52749,#52750,
#52751,#52752,#52753,#52754,#52755,#52756,#52757,#52758,#52759,#52760,#52761,
#52762,#52763,#52764,#52765,#52766,#52767,#52768,#52769,#52770,#52771,#52772,
#52773,#52774,#52775,#52776,#52777,#52778,#52779,#52780,#52781,#52782,#52783,
#52784,#52785,#52786,#52787,#52788,#52789,#52790,#52791,#52792,#52793,#52794,
#52795,#52796,#52797,#52798,#52799,#52800,#52801,#52802,#52803,#52804,#52805,
#52806,#52807,#52808,#52809,#52810,#52811,#52812,#52813,#52814,#52815,#52816,
#52817,#52818,#52819,#52820,#52821,#52822,#52823,#52824,#52825,#52826,#52827,
#52828,#52829,#52830,#52831,#52832,#52833,#52834,#52835,#52836,#52837,#52838,
#52839,#52840,#52841,#52842,#52843,#52844,#52845,#52846,#52847,#52848,#52849,
#52850,#52851,#52852,#52853),.UNSPECIFIED.,.F.,.F.,(4,2,2,2,2,2,2,2,2,2,
2,2,2,2,2,2,2,2,2,2,2,2,2,2,2,2,2,2,2,2,2,2,2,2,2,2,2,2,2,2,2,2,2,2,2,2,
2,2,2,2,2,2,2,2,2,2,2,2,2,2,2,2,2,2,2,2,2,2,2,2,2,2,2,2,2,2,2,2,2,2,2,2,
2,2,2,2,2,2,2,2,2,2,2,2,2,2,2,4),(-0.991236153398999,-0.990017865976998,
-0.964607879434727,-0.943939536477733,-0.922340595067815,-0.91885741669439,
-0.916924820957,-0.915292113581256,-0.913130929280484,-0.908382445715242,
-0.886866887530864,-0.847302037237583,-0.838963004043493,-0.835172705929818,
-0.83222782939185,-0.829008582358732,-0.823744300259359,-0.802366888533965,
-0.781707146913141,-0.775200231778021,-0.755609484870657,-0.752164588709421,
-0.750240610566901,-0.748606734880102,-0.746432954453861,-0.741614150301461,
-0.734848095536509,-0.714847540287023,-0.678606366608066,-0.672285034585661,
-0.668505018026553,-0.665561651923485,-0.662337497142246,-0.657050020559074,
-0.635291539871278,-0.604902387260126,-0.588774647522847,-0.585428344628336,
-0.583526493905173,-0.582038967196741,-0.579918876560076,-0.575393286400109,
-0.556033025010661,-0.522722974749949,-0.508051222584194,-0.503202641130385,
-0.500072158908907,-0.497092601997238,-0.493012007878406,-0.483182245670826,
-0.468851008500812,-0.448369897731706,-0.442067401786093,-0.42232462769962,
-0.418875902185947,-0.41695111693077,-0.41531747189453,-0.413145182831603,
-0.408334228069118,-0.401582738643682,-0.381657016717515,-0.345307233686974,
-0.338992396615969,-0.335214346322189,-0.332271413861628,-0.329046622193269,
-0.323755526239595,-0.301932589169151,-0.271249539362225,-0.255458224900243,
-0.252129948707979,-0.25023224562982,-0.248744110519532,-0.246618113211251,
-0.242060270886421,-0.222397340509815,-0.188245937030999,-0.174547669159655,
-0.169803535366404,-0.166695138592338,-0.163918924956194,-0.160999925688576,
-0.153812070139955,-0.144424563473928,-0.119742431598706,-0.0909134879582886,
-0.0862462850030538,-0.0841228543318537,-0.0824756176659709,-0.0805358393016943,
-0.0769189482045256,-0.0722721498534541,-0.0613630431171712,-0.0268129717864068,
-0.00882475856751817,-0.00411511755648563,-0.00192617516552268,-0.000492596523146994),
 .UNSPECIFIED.);
#609=B_SPLINE_CURVE_WITH_KNOTS('',3,(#52854,#52855,#52856,#52857,#52858,
#52859,#52860,#52861,#52862,#52863),.UNSPECIFIED.,.F.,.F.,(4,3,3,4),(89.2744165556861,
89.3888571977691,89.5076870191697,89.6265168405702),.UNSPECIFIED.);
#610=B_SPLINE_CURVE_WITH_KNOTS('',3,(#52865,#52866,#52867,#52868,#52869),
 .UNSPECIFIED.,.F.,.F.,(4,1,4),(-85.8810642303289,-85.7874539615475,-85.5277947543664),
 .UNSPECIFIED.);
#611=B_SPLINE_CURVE_WITH_KNOTS('',3,(#52870,#52871,#52872,#52873,#52874,
#52875,#52876,#52877,#52878,#52879,#52880,#52881,#52882,#52883,#52884,#52885,
#52886,#52887,#52888,#52889,#52890,#52891,#52892,#52893,#52894,#52895,#52896,
#52897,#52898,#52899,#52900,#52901,#52902,#52903,#52904,#52905,#52906,#52907,
#52908,#52909,#52910,#52911,#52912,#52913,#52914,#52915,#52916,#52917,#52918,
#52919,#52920,#52921,#52922,#52923,#52924,#52925,#52926,#52927,#52928,#52929,
#52930,#52931,#52932,#52933,#52934,#52935,#52936,#52937,#52938,#52939,#52940,
#52941,#52942,#52943,#52944,#52945,#52946,#52947,#52948,#52949,#52950,#52951,
#52952,#52953,#52954,#52955,#52956,#52957,#52958,#52959,#52960,#52961,#52962,
#52963,#52964,#52965,#52966,#52967,#52968,#52969,#52970,#52971,#52972,#52973,
#52974,#52975,#52976,#52977,#52978,#52979,#52980,#52981,#52982,#52983,#52984,
#52985,#52986,#52987,#52988,#52989,#52990,#52991,#52992,#52993,#52994,#52995,
#52996,#52997,#52998,#52999,#53000,#53001,#53002,#53003,#53004,#53005,#53006,
#53007,#53008,#53009,#53010,#53011,#53012,#53013,#53014,#53015,#53016,#53017,
#53018,#53019,#53020,#53021,#53022,#53023,#53024,#53025,#53026,#53027,#53028,
#53029,#53030,#53031,#53032,#53033,#53034,#53035,#53036,#53037,#53038,#53039,
#53040,#53041,#53042,#53043,#53044,#53045,#53046,#53047,#53048,#53049,#53050,
#53051,#53052,#53053,#53054,#53055,#53056,#53057,#53058,#53059,#53060,#53061,
#53062,#53063,#53064,#53065,#53066,#53067),.UNSPECIFIED.,.F.,.F.,(4,2,2,
2,2,2,2,2,2,2,2,2,2,2,2,2,2,2,2,2,2,2,2,2,2,2,2,2,2,2,2,2,2,2,2,2,2,2,2,
2,2,2,2,2,2,2,2,2,2,2,2,2,2,2,2,2,2,2,2,2,2,2,2,2,2,2,2,2,2,2,2,2,2,2,2,
2,2,2,2,2,2,2,2,2,2,2,2,2,2,2,2,2,2,2,2,2,2,2,4),(-2.10007152061629,-2.0785364363192,
-2.06876879443929,-2.06502723271782,-2.06215732255702,-2.05921404607757,
-2.05598824670138,-2.05069402147021,-2.03118054673824,-2.00235696093729,
-1.98395474968524,-1.97974526720886,-1.97762987828826,-1.97614281246107,
-1.97423760999817,-1.97087673633506,-1.95440479701274,-1.92475158618459,
-1.91005468091917,-1.90004862616664,-1.89594033809507,-1.89295588930762,
-1.88983397620689,-1.88502666320277,-1.87074353320602,-1.83712252901638,
-1.81765266149352,-1.81311512035469,-1.81099274588001,-1.80950487068175,
-1.80760434937467,-1.80426421072928,-1.78830678225958,-1.75774075509178,
-1.73594359349288,-1.73065335347535,-1.7274285024067,-1.72448514336714,
-1.72070602457934,-1.71438825398602,-1.67812384382059,-1.65816570442503,
-1.65140813162939,-1.64659340759779,-1.64442030513839,-1.64278642186039,
-1.64086183814362,-1.63741442463673,-1.61774086211831,-1.61091935796612,
-1.58934289314332,-1.57589480595146,-1.56650337691086,-1.56249273044517,
-1.55952460204975,-1.55636969220717,-1.55140653185989,-1.53567471638681,
-1.50330150153963,-1.48428216903819,-1.47979338804293,-1.47768013943784,
-1.47619333302005,-1.47428671986486,-1.47091952137281,-1.45431269890522,
-1.42472988080548,-1.40267757024358,-1.39737216894697,-1.39414406265657,
-1.3912015888965,-1.38742894494581,-1.38113410054262,-1.34447867491172,
-1.32477939660341,-1.31807187240799,-1.3132839097142,-1.31111561939044,
-1.30946745101539,-1.30753341744949,-1.30404363491216,-1.28090286767243,
-1.26369671357128,-1.23877829312778,-1.23190785859255,-1.22835316959585,
-1.22571934640295,-1.22241412492548,-1.21674873049364,-1.18586948899327,
-1.16100699126578,-1.15264414030638,-1.14700762821841,-1.14469491349508,
-1.14302837901843,-1.14117530047933,-1.13796378017104,-1.12482076840509,
-1.10917023491673),.UNSPECIFIED.);
#612=B_SPLINE_CURVE_WITH_KNOTS('',3,(#53072,#53073,#53074,#53075,#53076,
#53077,#53078,#53079,#53080,#53081,#53082,#53083,#53084,#53085,#53086,#53087,
#53088,#53089,#53090,#53091,#53092,#53093,#53094,#53095,#53096,#53097,#53098,
#53099,#53100,#53101,#53102,#53103,#53104,#53105,#53106,#53107,#53108,#53109,
#53110,#53111,#53112,#53113,#53114,#53115,#53116,#53117,#53118,#53119,#53120,
#53121,#53122,#53123,#53124,#53125,#53126,#53127,#53128,#53129,#53130,#53131,
#53132,#53133,#53134,#53135,#53136,#53137,#53138,#53139,#53140,#53141,#53142,
#53143,#53144,#53145,#53146,#53147,#53148,#53149,#53150,#53151,#53152,#53153,
#53154,#53155,#53156,#53157,#53158,#53159,#53160,#53161,#53162,#53163,#53164,
#53165,#53166,#53167,#53168,#53169,#53170,#53171,#53172,#53173,#53174,#53175,
#53176,#53177,#53178,#53179,#53180,#53181,#53182,#53183,#53184,#53185,#53186,
#53187,#53188,#53189,#53190,#53191,#53192,#53193,#53194,#53195,#53196,#53197,
#53198,#53199,#53200,#53201,#53202,#53203,#53204,#53205,#53206,#53207,#53208,
#53209,#53210,#53211,#53212,#53213,#53214,#53215,#53216,#53217,#53218,#53219,
#53220,#53221,#53222,#53223,#53224,#53225,#53226,#53227,#53228,#53229,#53230,
#53231,#53232,#53233,#53234,#53235,#53236,#53237,#53238,#53239,#53240,#53241,
#53242,#53243,#53244,#53245,#53246,#53247,#53248,#53249,#53250,#53251,#53252,
#53253,#53254,#53255,#53256,#53257,#53258,#53259,#53260,#53261,#53262,#53263,
#53264,#53265,#53266,#53267,#53268,#53269,#53270,#53271,#53272,#53273,#53274,
#53275,#53276,#53277),.UNSPECIFIED.,.F.,.F.,(4,2,2,2,2,2,2,2,2,2,2,2,2,
2,2,2,2,2,2,2,2,2,2,2,2,2,2,2,2,2,2,2,2,2,2,2,2,2,2,2,2,2,2,2,2,2,2,2,2,
2,2,2,2,2,2,2,2,2,2,2,2,2,2,2,2,2,2,2,2,2,2,2,2,2,2,2,2,2,2,2,2,2,2,2,2,
2,2,2,2,2,2,2,2,2,2,2,2,2,2,2,2,2,4),(-2.04110855067476,-2.03076381586652,
-2.0089897584076,-2.00370085006763,-2.00047627473838,-1.99753282492654,
-1.99375311899073,-1.98743331218493,-1.95119882772989,-1.9227955618766,
-1.91903491361895,-1.91706514786033,-1.91542090533246,-1.91330183013505,
-1.9087821044297,-1.87733516721823,-1.84328564492068,-1.8374611115415,-1.83412207505555,
-1.83120008618467,-1.82755386181497,-1.82045488802992,-1.79003848636111,
-1.76583945065451,-1.75833314785634,-1.75312652038043,-1.75088491962852,
-1.74922852743731,-1.74733944422112,-1.74404971753485,-1.72886487565409,
-1.69991045873406,-1.68066422640008,-1.67235630589557,-1.66853045390329,
-1.66558949205946,-1.66235617697529,-1.65702615309848,-1.63683232564857,
-1.59348012562206,-1.58694185735254,-1.5844926639368,-1.58280268163173,
-1.5810039402212,-1.57804075298967,-1.56789594052795,-1.5614471595886,-1.53077701651864,
-1.50895423388436,-1.50366243583937,-1.50043725944239,-1.49749401035757,
-1.49371560151973,-1.48740032500443,-1.45108553155655,-1.43115839232335,
-1.42440671967328,-1.41959513566273,-1.41742260217782,-1.41578878496851,
-1.41386385492518,-1.41041487609998,-1.39068210556499,-1.3843349556325,
-1.36377373663007,-1.34226063994424,-1.33698756646965,-1.33376636446422,
-1.33082192576004,-1.32703529271342,-1.31871741782793,-1.27915109257104,
-1.25763989993403,-1.25289175908312,-1.25073061963213,-1.24909788341911,
-1.24716521061065,-1.24368172671001,-1.22210948972152,-1.21796305475088,
-1.19793272430067,-1.18314095768735,-1.1730891574056,-1.16897367766887,
-1.16598788307167,-1.16323883382283,-1.15948784036015,-1.15190960686635,
-1.1124401334353,-1.09095944765144,-1.08621421578381,-1.08405354553322,
-1.0824207897418,-1.08048764160776,-1.07700226613155,-1.05522095651838,
-1.05034361097503,-1.01159072374133,-1.00545858411251,-1.00169182335993,
-0.998757891544168,-0.99549323853491,-0.991236153398999),.UNSPECIFIED.);
#613=B_SPLINE_CURVE_WITH_KNOTS('',3,(#53278,#53279,#53280,#53281,#53282,
#53283,#53284,#53285,#53286,#53287,#53288,#53289,#53290,#53291,#53292,#53293,
#53294,#53295,#53296,#53297,#53298,#53299,#53300,#53301,#53302,#53303,#53304,
#53305,#53306,#53307,#53308,#53309,#53310,#53311,#53312,#53313,#53314,#53315,
#53316,#53317,#53318,#53319,#53320,#53321,#53322,#53323,#53324,#53325,#53326,
#53327,#53328,#53329,#53330,#53331,#53332,#53333,#53334,#53335,#53336,#53337,
#53338,#53339,#53340,#53341,#53342,#53343,#53344,#53345,#53346,#53347,#53348,
#53349,#53350,#53351,#53352,#53353,#53354,#53355,#53356,#53357,#53358,#53359,
#53360,#53361,#53362,#53363,#53364,#53365,#53366,#53367,#53368,#53369,#53370,
#53371,#53372,#53373,#53374,#53375,#53376,#53377,#53378,#53379,#53380,#53381,
#53382,#53383,#53384,#53385,#53386,#53387,#53388,#53389,#53390,#53391,#53392,
#53393,#53394,#53395,#53396,#53397,#53398,#53399,#53400,#53401,#53402,#53403,
#53404,#53405,#53406,#53407,#53408,#53409,#53410,#53411,#53412,#53413,#53414,
#53415,#53416,#53417,#53418,#53419,#53420,#53421,#53422,#53423,#53424,#53425,
#53426,#53427,#53428,#53429,#53430,#53431,#53432,#53433,#53434,#53435,#53436,
#53437,#53438,#53439,#53440,#53441,#53442,#53443,#53444,#53445,#53446,#53447,
#53448,#53449,#53450,#53451,#53452,#53453,#53454,#53455,#53456,#53457,#53458,
#53459,#53460,#53461,#53462,#53463,#53464,#53465,#53466,#53467,#53468,#53469,
#53470,#53471,#53472,#53473,#53474,#53475,#53476,#53477,#53478,#53479,#53480,
#53481,#53482,#53483,#53484,#53485),.UNSPECIFIED.,.F.,.F.,(4,2,2,2,2,2,
2,2,2,2,2,2,2,2,2,2,2,2,2,2,2,2,2,2,2,2,2,2,2,2,2,2,2,2,2,2,2,2,2,2,2,2,
2,2,2,2,2,2,2,2,2,2,2,2,2,2,2,2,2,2,2,2,2,2,2,2,2,2,2,2,2,2,2,2,2,2,2,2,
2,2,2,2,2,2,2,2,2,2,2,2,2,2,2,2,2,2,2,2,2,2,2,2,2,4),(-1.10917023491673,
-1.09780314118422,-1.07225908258597,-1.06530958502227,-1.06173924456896,
-1.05910391043913,-1.05580982384355,-1.05019632888415,-1.02079744724882,
-0.991284433603716,-0.981650882393839,-0.978739801476121,-0.976952504346429,
-0.975255931018385,-0.972771926128064,-0.965985524808992,-0.955132329620842,
-0.933346313864944,-0.903406464592416,-0.89773614042774,-0.89442984961194,
-0.891796144927973,-0.888242899319584,-0.881379711288852,-0.856519376055898,
-0.839293624574117,-0.816141745348745,-0.812652454382971,-0.810718532503337,
-0.809070373076671,-0.806901949031408,-0.80211321737921,-0.795403477182408,
-0.775694480284611,-0.739015888895629,-0.73272011790953,-0.728947250626557,
-0.726004774124995,-0.722776837720733,-0.717472097304373,-0.695425227256277,
-0.66590515143579,-0.656794159610615,-0.648140599938779,-0.645338199308374,
-0.643574731727522,-0.641861932312708,-0.63929625790687,-0.631894661130396,
-0.619577769341614,-0.582592117112216,-0.568401254974707,-0.56360377197765,
-0.560484046483025,-0.557498655147684,-0.553384158147427,-0.543336734996394,
-0.528555263686441,-0.508544994584828,-0.504278305999244,-0.482840000822797,
-0.479358804460191,-0.477426768689665,-0.475794169803756,-0.47363264486231,
-0.46888156102796,-0.447336716776784,-0.407675194317095,-0.399431332731411,
-0.395658018203836,-0.392715731836914,-0.38948855191263,-0.3841863293089,
-0.36217520988874,-0.332095131052859,-0.315950488554445,-0.312603752403881,
-0.310701885660114,-0.309214500928508,-0.307094799918483,-0.302570723735803,
-0.283222458346412,-0.249943173278937,-0.235241836313093,-0.230390355519392,
-0.227259427235587,-0.22428046285279,-0.220202299774329,-0.210386694139145,
-0.19608391261695,-0.175665101246482,-0.151511714522243,-0.146768846520951,
-0.144631870956978,-0.142983443199958,-0.141215798394648,-0.138114853869353,
-0.134124858945641,-0.12544065447551,-0.0954286080090174,-0.0700939486962987,
-0.064493435702309,-0.0612024694929878,-0.0595374781479462),
 .UNSPECIFIED.);
#614=B_SPLINE_CURVE_WITH_KNOTS('',3,(#53491,#53492,#53493,#53494,#53495,
#53496,#53497,#53498,#53499,#53500,#53501,#53502,#53503,#53504,#53505,#53506,
#53507,#53508,#53509,#53510,#53511,#53512,#53513,#53514,#53515,#53516,#53517,
#53518,#53519,#53520,#53521,#53522,#53523,#53524,#53525,#53526,#53527,#53528,
#53529,#53530,#53531,#53532,#53533,#53534,#53535,#53536,#53537,#53538,#53539,
#53540,#53541,#53542,#53543,#53544,#53545,#53546,#53547,#53548,#53549,#53550,
#53551,#53552,#53553,#53554,#53555,#53556,#53557,#53558,#53559,#53560,#53561,
#53562,#53563,#53564,#53565,#53566,#53567,#53568,#53569,#53570,#53571,#53572,
#53573,#53574,#53575,#53576,#53577,#53578,#53579,#53580,#53581,#53582,#53583,
#53584,#53585,#53586,#53587,#53588,#53589,#53590,#53591,#53592,#53593,#53594,
#53595,#53596,#53597,#53598,#53599,#53600,#53601,#53602,#53603,#53604,#53605,
#53606,#53607,#53608,#53609,#53610,#53611,#53612,#53613,#53614,#53615,#53616,
#53617,#53618,#53619,#53620,#53621,#53622,#53623,#53624,#53625,#53626,#53627,
#53628,#53629,#53630,#53631,#53632,#53633,#53634,#53635,#53636,#53637,#53638,
#53639,#53640,#53641,#53642,#53643,#53644,#53645,#53646,#53647,#53648,#53649,
#53650,#53651,#53652,#53653,#53654,#53655,#53656,#53657,#53658,#53659,#53660,
#53661,#53662,#53663,#53664,#53665,#53666,#53667,#53668,#53669,#53670,#53671,
#53672,#53673,#53674,#53675,#53676,#53677,#53678,#53679,#53680,#53681,#53682,
#53683,#53684,#53685,#53686,#53687,#53688,#53689,#53690,#53691,#53692,#53693,
#53694,#53695,#53696,#53697,#53698,#53699,#53700),.UNSPECIFIED.,.F.,.F.,
(4,2,2,2,2,2,2,2,2,2,2,2,2,2,2,2,2,2,2,2,2,2,2,2,2,2,2,2,2,2,2,2,2,2,2,
2,2,2,2,2,2,2,2,2,2,2,2,2,2,2,2,2,2,2,2,2,2,2,2,2,2,2,2,2,2,2,2,2,2,2,2,
2,2,2,2,2,2,2,2,2,2,2,2,2,2,2,2,2,2,2,2,2,2,2,2,2,2,2,2,2,2,2,2,2,4),(-0.991340061094534,
-0.98920246580239,-0.985892070943082,-0.983998417543123,-0.9823432842587,
-0.980110386246792,-0.974953970657174,-0.967544151433446,-0.943937354432828,
-0.912714269366428,-0.905623704154458,-0.90197943989973,-0.899057888336441,
-0.895718120940077,-0.889889042822999,-0.855667907249648,-0.824460926690277,
-0.819932370416947,-0.817811816006102,-0.816167668474606,-0.814199530731012,
-0.81044599135912,-0.782161991903423,-0.745755684101324,-0.739444483520501,
-0.735667531524847,-0.732724835093212,-0.729499672142621,-0.724206501792553,
-0.702346267814432,-0.671566076484301,-0.655890806045303,-0.652577464861746,
-0.650683172186911,-0.649028228394813,-0.646796586869404,-0.641647315516918,
-0.634251286145616,-0.61072709880859,-0.579397105721552,-0.572307765744901,
-0.568663805211868,-0.565742339225463,-0.562402497996578,-0.55657283896063,
-0.522141438871249,-0.491184089837036,-0.486631504524908,-0.48450650002899,
-0.482862087066209,-0.480897454163308,-0.477160737336082,-0.472314058866212,
-0.460681236454466,-0.439388367291313,-0.410256793518379,-0.404609510813054,
-0.401276691124032,-0.398382162433067,-0.394741678270005,-0.387432190858959,
-0.377835793013308,-0.352143498200701,-0.324794333482777,-0.320082217557296,
-0.31795072339367,-0.316302806272113,-0.314369013785592,-0.31078001980745,
-0.282230708124701,-0.245814300630239,-0.239504047872713,-0.23572745066662,
-0.232784908843778,-0.229559791713426,-0.224266409621652,-0.202399707202107,
-0.171610172324106,-0.155971765936306,-0.152648983812978,-0.150752608621542,
-0.149153715295316,-0.149134145752116,-0.149114703943759,-0.149095383505877,
-0.149076178237325,-0.149057082091785,-0.149038089174465,-0.149019193737152,
-0.14900039015904,-0.148981672947616,-0.148963036725475,-0.146845365989864,
-0.144331827442144,-0.139921370409683,-0.1298384769529,-0.0943091076171302,
-0.0760052498260046,-0.0708057193007756,-0.0676007636255934,-0.0646523535893921,
-0.060768233202206,-0.0521261683564409,-0.0242665367690054,-0.000492710661275274),
 .UNSPECIFIED.);
#615=B_SPLINE_CURVE_WITH_KNOTS('',3,(#53701,#53702,#53703,#53704,#53705,
#53706,#53707,#53708,#53709,#53710,#53711,#53712,#53713,#53714,#53715,#53716,
#53717,#53718,#53719,#53720),.UNSPECIFIED.,.F.,.F.,(4,2,2,2,2,2,2,2,2,4),
(-2.09993882802925,-2.08869886965324,-2.08628696029132,-2.08456699226199,
-2.083031835045,-2.08149453819177,-2.07937193789139,-2.07393091411062,-2.05926295066118,
-2.04110855067476),.UNSPECIFIED.);
#616=B_SPLINE_CURVE_WITH_KNOTS('',3,(#53722,#53723,#53724,#53725,#53726,
#53727,#53728,#53729,#53730,#53731,#53732,#53733),.UNSPECIFIED.,.F.,.F.,
(4,2,2,2,2,4),(-0.0595374781479462,-0.0582743076702352,-0.0545553048994626,
-0.0468312306777383,-0.0365100484917665,-0.000492659668756888),
 .UNSPECIFIED.);
#617=B_SPLINE_CURVE_WITH_KNOTS('',3,(#53734,#53735,#53736,#53737,#53738,
#53739,#53740,#53741,#53742,#53743,#53744,#53745,#53746,#53747,#53748,#53749,
#53750,#53751,#53752,#53753,#53754,#53755,#53756,#53757,#53758,#53759,#53760,
#53761,#53762,#53763,#53764,#53765,#53766,#53767,#53768,#53769,#53770,#53771,
#53772,#53773,#53774,#53775,#53776,#53777,#53778,#53779,#53780,#53781,#53782,
#53783,#53784,#53785,#53786,#53787,#53788,#53789,#53790,#53791,#53792,#53793,
#53794,#53795,#53796,#53797,#53798,#53799,#53800,#53801,#53802,#53803,#53804,
#53805,#53806,#53807,#53808,#53809,#53810,#53811,#53812,#53813,#53814,#53815,
#53816,#53817,#53818,#53819,#53820,#53821,#53822,#53823,#53824,#53825,#53826,
#53827,#53828,#53829,#53830,#53831,#53832,#53833,#53834,#53835,#53836,#53837,
#53838,#53839,#53840,#53841,#53842,#53843,#53844,#53845,#53846,#53847,#53848,
#53849,#53850,#53851,#53852,#53853,#53854,#53855,#53856,#53857,#53858,#53859,
#53860,#53861,#53862,#53863,#53864,#53865,#53866,#53867,#53868,#53869,#53870,
#53871,#53872,#53873,#53874,#53875,#53876,#53877,#53878,#53879,#53880,#53881,
#53882,#53883,#53884,#53885,#53886,#53887,#53888,#53889,#53890,#53891,#53892,
#53893,#53894,#53895,#53896,#53897,#53898,#53899,#53900,#53901,#53902,#53903,
#53904,#53905,#53906,#53907,#53908,#53909,#53910,#53911,#53912,#53913,#53914,
#53915,#53916,#53917,#53918,#53919,#53920,#53921,#53922,#53923,#53924,#53925,
#53926,#53927),.UNSPECIFIED.,.F.,.F.,(4,2,2,2,2,2,2,2,2,2,2,2,2,2,2,2,2,
2,2,2,2,2,2,2,2,2,2,2,2,2,2,2,2,2,2,2,2,2,2,2,2,2,2,2,2,2,2,2,2,2,2,2,2,
2,2,2,2,2,2,2,2,2,2,2,2,2,2,2,2,2,2,2,2,2,2,2,2,2,2,2,2,2,2,2,2,2,2,2,2,
2,2,2,2,2,2,2,4),(-2.10000173286267,-2.08784529945252,-2.0818241350934,
-2.07949850599191,-2.0778111684359,-2.07613401143259,-2.07430816150208,
-2.07122208891968,-2.05973632205585,-2.0406965402433,-2.02426558874489,
-2.00238112718897,-1.99708503033397,-1.99385859131561,-1.99091506206345,
-1.98713749800015,-1.98082635373945,-1.94442082373072,-1.91584332378824,
-1.91227305338482,-1.91034281151202,-1.90869375455209,-1.90655549055158,
-1.90180801965512,-1.87801516213019,-1.85810522698771,-1.84324566348585,
-1.83316100065038,-1.82904006134694,-1.82605296058888,-1.82293408717729,
-1.81814324970362,-1.8040214362917,-1.77025181881292,-1.75072729195109,
-1.74618340308607,-1.74405958903847,-1.74257129557485,-1.74067106548965,
-1.73733322421561,-1.72144948256797,-1.69101286710652,-1.66901622816419,
-1.66371331839731,-1.66048533576287,-1.65754207797673,-1.65376718790769,
-1.64746578413458,-1.61088989558763,-1.58249500163516,-1.57890531012757,
-1.57697093211146,-1.57532239559003,-1.57318990373664,-1.56847489950099,
-1.54107916896174,-1.51538017288048,-1.50578041664814,-1.49846906384927,
-1.49482743453616,-1.49193191133557,-1.48859784864288,-1.48294820288119,
-1.45382101360991,-1.43252740890118,-1.42090686924639,-1.4160628922804,
-1.41232721597242,-1.41036238500471,-1.40871736604499,-1.40659097788066,
-1.40203333348044,-1.37106994167086,-1.33659729825625,-1.33076479108221,
-1.3274236643598,-1.32450128086828,-1.32085644192214,-1.31376619512649,
-1.28248779203966,-1.25894019818624,-1.25154000611395,-1.2463877398711,
-1.2441551699199,-1.24249966160833,-1.24060489505375,-1.23729101618844,
-1.22162033473911,-1.19087605209644,-1.16892862033792,-1.16362881542626,
-1.16040159976283,-1.15745831756361,-1.15368239412195,-1.14737699328768,
-1.11087458577517,-1.10913982844865),.UNSPECIFIED.);
#618=B_SPLINE_CURVE_WITH_KNOTS('',3,(#53932,#53933,#53934,#53935,#53936,
#53937,#53938,#53939,#53940,#53941,#53942,#53943,#53944,#53945,#53946,#53947,
#53948,#53949,#53950,#53951,#53952,#53953,#53954,#53955,#53956,#53957,#53958,
#53959,#53960,#53961,#53962,#53963,#53964,#53965,#53966,#53967,#53968,#53969,
#53970,#53971,#53972,#53973,#53974,#53975,#53976,#53977,#53978,#53979,#53980,
#53981,#53982,#53983,#53984,#53985,#53986,#53987,#53988,#53989,#53990,#53991,
#53992,#53993,#53994,#53995,#53996,#53997,#53998,#53999,#54000,#54001,#54002,
#54003,#54004,#54005,#54006,#54007,#54008,#54009,#54010,#54011,#54012,#54013,
#54014,#54015,#54016,#54017,#54018,#54019,#54020,#54021,#54022,#54023,#54024,
#54025,#54026,#54027,#54028,#54029,#54030,#54031,#54032,#54033,#54034,#54035,
#54036,#54037,#54038,#54039,#54040,#54041,#54042,#54043,#54044,#54045,#54046,
#54047,#54048,#54049,#54050,#54051,#54052,#54053,#54054,#54055,#54056,#54057,
#54058,#54059,#54060,#54061,#54062,#54063,#54064,#54065,#54066,#54067,#54068,
#54069,#54070,#54071,#54072,#54073,#54074,#54075,#54076,#54077,#54078,#54079,
#54080,#54081,#54082,#54083,#54084,#54085,#54086,#54087,#54088,#54089,#54090,
#54091,#54092,#54093,#54094,#54095,#54096,#54097,#54098,#54099,#54100,#54101,
#54102,#54103,#54104,#54105,#54106,#54107,#54108,#54109,#54110,#54111,#54112,
#54113,#54114,#54115,#54116,#54117,#54118,#54119,#54120,#54121,#54122,#54123,
#54124,#54125,#54126,#54127,#54128,#54129,#54130,#54131),.UNSPECIFIED.,
 .F.,.F.,(4,2,2,2,2,2,2,2,2,2,2,2,2,2,2,2,2,2,2,2,2,2,2,2,2,2,2,2,2,2,2,
2,2,2,2,2,2,2,2,2,2,2,2,2,2,2,2,2,2,2,2,2,2,2,2,2,2,2,2,2,2,2,2,2,2,2,2,
2,2,2,2,2,2,2,2,2,2,2,2,2,2,2,2,2,2,2,2,2,2,2,2,2,2,2,2,2,2,2,2,4),(-2.04097989592064,
-2.01643454881326,-1.99867457066985,-1.98823495665113,-1.98533631711536,
-1.98355188807003,-1.98187373456921,-1.97979424848172,-1.97461318682226,
-1.93094583053922,-1.90926005730472,-1.90397737789773,-1.90075461085136,
-1.89781152551908,-1.89403050179105,-1.88574139544896,-1.84615706595855,
-1.82463996225972,-1.81989185650961,-1.81773103186237,-1.81609866344362,
-1.81416658211516,-1.81068452397676,-1.78917818454528,-1.78496385128544,
-1.76502065433151,-1.75018716651009,-1.7401160856542,-1.73599824120865,
-1.73301257318057,-1.72989447874049,-1.72510339229687,-1.71096730234241,
-1.67395778297624,-1.66164165710378,-1.65661185068838,-1.65276631331365,
-1.65077934945949,-1.64913666607856,-1.64703984197957,-1.64263691113105,
-1.60940824133699,-1.58149842274345,-1.57286227549758,-1.56897911009622,
-1.56603078727429,-1.56282530839965,-1.55762350900728,-1.53928147727738,
-1.5039076559364,-1.49377807312749,-1.48731153633058,-1.48487291656532,
-1.48318514643127,-1.48160694366644,-1.47885640457167,-1.47063158883834,
-1.46097793927844,-1.43144234155053,-1.4093908147684,-1.40408622499255,
-1.40085871152601,-1.39791684553085,-1.39414507832638,-1.38785193178936,
-1.35119126814421,-1.33150154608391,-1.32479638229279,-1.3200099074253,
-1.31784214574603,-1.31619431841227,-1.31426062354715,-1.3107713203957,
-1.28759459939239,-1.27033585626588,-1.24787614812831,-1.23948837808926,
-1.23564870486035,-1.23270630613491,-1.22948053264786,-1.22418418485653,
-1.20461265651106,-1.16085419733883,-1.1562515897723,-1.15266118188117,
-1.15072706590745,-1.14907916860977,-1.14694803739181,-1.14223810389979,
-1.11470911711937,-1.08911525072692,-1.07480794059978,-1.07013750571097,
-1.06704446230174,-1.06407714097964,-1.05989566405639,-1.05017299558284,
-1.03563134770873,-1.00482702409126,-0.991340061094534),.UNSPECIFIED.);
#619=B_SPLINE_CURVE_WITH_KNOTS('',3,(#54132,#54133,#54134,#54135,#54136,
#54137,#54138,#54139,#54140,#54141,#54142,#54143,#54144,#54145,#54146,#54147,
#54148,#54149,#54150,#54151,#54152,#54153,#54154,#54155,#54156,#54157,#54158,
#54159,#54160,#54161,#54162,#54163,#54164,#54165,#54166,#54167,#54168,#54169,
#54170,#54171,#54172,#54173,#54174,#54175,#54176,#54177,#54178,#54179,#54180,
#54181,#54182,#54183,#54184,#54185,#54186,#54187,#54188,#54189,#54190,#54191,
#54192,#54193,#54194,#54195,#54196,#54197,#54198,#54199,#54200,#54201,#54202,
#54203,#54204,#54205,#54206,#54207,#54208,#54209,#54210,#54211,#54212,#54213,
#54214,#54215,#54216,#54217,#54218,#54219,#54220,#54221,#54222,#54223,#54224,
#54225,#54226,#54227,#54228,#54229,#54230,#54231,#54232,#54233,#54234,#54235,
#54236,#54237,#54238,#54239,#54240,#54241,#54242,#54243,#54244,#54245,#54246,
#54247,#54248,#54249,#54250,#54251,#54252,#54253,#54254,#54255,#54256,#54257,
#54258,#54259,#54260,#54261,#54262,#54263,#54264,#54265,#54266,#54267,#54268,
#54269,#54270,#54271,#54272,#54273,#54274,#54275,#54276,#54277,#54278,#54279,
#54280,#54281,#54282,#54283,#54284,#54285,#54286,#54287,#54288,#54289,#54290,
#54291,#54292,#54293,#54294,#54295,#54296,#54297,#54298,#54299,#54300,#54301,
#54302,#54303,#54304,#54305,#54306,#54307,#54308,#54309,#54310,#54311,#54312,
#54313,#54314,#54315,#54316,#54317,#54318,#54319,#54320,#54321,#54322,#54323,
#54324,#54325,#54326,#54327,#54328,#54329,#54330,#54331,#54332,#54333,#54334,
#54335,#54336,#54337,#54338,#54339,#54340,#54341,#54342,#54343,#54344,#54345,
#54346,#54347,#54348,#54349,#54350,#54351,#54352,#54353,#54354,#54355,#54356,
#54357),.UNSPECIFIED.,.F.,.F.,(4,2,2,2,2,2,2,2,2,2,2,2,2,2,2,2,2,2,2,2,
2,2,2,2,2,2,2,2,2,2,2,2,2,2,2,2,2,2,2,2,2,2,2,2,2,2,2,2,2,2,2,2,2,2,2,2,
2,2,2,2,2,2,2,2,2,2,2,2,2,2,2,2,2,2,2,2,2,2,2,2,2,2,2,2,2,2,2,2,2,2,2,2,
2,2,2,2,2,2,2,2,2,2,2,2,2,2,2,2,2,2,2,2,4),(-1.10913982844865,-1.09106795055996,
-1.084339173503,-1.07953965907219,-1.0773690951644,-1.075735260039,-1.07380849983863,
-1.07035212401128,-1.05034070711872,-1.00500181410813,-0.998796004615634,
-0.995048507963371,-0.992109253737245,-0.988867863748533,-0.983501070336844,
-0.960350817368616,-0.930304611090647,-0.915259285440901,-0.911976323597886,
-0.910088670522428,-0.90843177836852,-0.906187085717017,-0.900962974022094,
-0.893421857911931,-0.869012640474297,-0.838843482889157,-0.831733018178526,
-0.828084257752818,-0.825161867104849,-0.821824138487046,-0.816006486673927,
-0.779593122733005,-0.750755265648821,-0.746087432986437,-0.743963636303344,
-0.742316129337228,-0.740376097056809,-0.736758660438702,-0.70720974270184,
-0.671929604503066,-0.665562772728414,-0.6617697733166,-0.65882439883221,
-0.655606218072681,-0.650347376521122,-0.629059517547184,-0.608319980153307,
-0.601733200781957,-0.582200106433717,-0.578756636158879,-0.576832920459043,
-0.575198902864116,-0.573024444829927,-0.568202222356984,-0.561429840172035,
-0.541396630496964,-0.50520549265272,-0.49888142881401,-0.495100549399652,
-0.492156947280929,-0.488932972074349,-0.483646795348441,-0.461912400671883,
-0.431660848866696,-0.415380230393842,-0.412027905528294,-0.41012464830468,
-0.408637300633719,-0.406519119590564,-0.40200395121782,-0.38274076947758,
-0.34969940393548,-0.334719566271866,-0.329835559107048,-0.326697510677828,
-0.323721627064164,-0.319663319304236,-0.309975102200079,-0.295932772271624,
-0.27521813333345,-0.268188939960367,-0.248899798409811,-0.245463052959539,
-0.243540896974316,-0.242056603922087,-0.239965790128632,-0.235595186403043,
-0.217633463249286,-0.185672870046334,-0.168553711526254,-0.163442706653727,
-0.160256378829578,-0.157506521636873,-0.157347050096386,-0.1571997612204,
-0.157060874279407,-0.156927548981441,-0.156797526364973,-0.156668907090355,
-0.156540004483214,-0.156409239524296,-0.153312770234407,-0.148952569479307,
-0.141429206504758,-0.124370185405663,-0.105014574945038,-0.0823638306380467,
-0.0788764371682638,-0.0769430257481847,-0.0753106291282405,-0.0731511473577938,
-0.0684113095755912,-0.0594010420905767),.UNSPECIFIED.);
#620=B_SPLINE_CURVE_WITH_KNOTS('',3,(#54363,#54364,#54365,#54366,#54367,
#54368,#54369,#54370,#54371,#54372,#54373,#54374,#54375,#54376,#54377,#54378,
#54379,#54380,#54381,#54382,#54383,#54384,#54385,#54386,#54387,#54388,#54389,
#54390,#54391,#54392,#54393,#54394,#54395,#54396,#54397,#54398,#54399,#54400,
#54401,#54402,#54403,#54404,#54405,#54406,#54407,#54408,#54409,#54410,#54411,
#54412,#54413,#54414,#54415,#54416,#54417,#54418,#54419,#54420,#54421,#54422,
#54423,#54424,#54425,#54426,#54427,#54428,#54429,#54430,#54431,#54432,#54433,
#54434,#54435,#54436,#54437,#54438,#54439,#54440,#54441,#54442,#54443,#54444,
#54445,#54446,#54447,#54448,#54449,#54450,#54451,#54452,#54453,#54454,#54455,
#54456,#54457,#54458,#54459,#54460,#54461,#54462,#54463,#54464,#54465,#54466,
#54467,#54468,#54469,#54470,#54471,#54472,#54473,#54474,#54475,#54476,#54477,
#54478,#54479,#54480,#54481,#54482,#54483,#54484,#54485,#54486,#54487,#54488,
#54489,#54490,#54491,#54492,#54493,#54494,#54495,#54496,#54497,#54498,#54499,
#54500,#54501,#54502,#54503,#54504,#54505,#54506,#54507,#54508,#54509,#54510,
#54511,#54512,#54513,#54514,#54515,#54516,#54517,#54518,#54519,#54520,#54521,
#54522,#54523,#54524,#54525,#54526,#54527,#54528,#54529,#54530,#54531,#54532,
#54533,#54534,#54535,#54536,#54537,#54538,#54539,#54540,#54541,#54542,#54543,
#54544,#54545,#54546,#54547,#54548,#54549,#54550,#54551,#54552,#54553,#54554,
#54555,#54556,#54557,#54558,#54559,#54560),.UNSPECIFIED.,.F.,.F.,(4,2,2,
2,2,2,2,2,2,2,2,2,2,2,2,2,2,2,2,2,2,2,2,2,2,2,2,2,2,2,2,2,2,2,2,2,2,2,2,
2,2,2,2,2,2,2,2,2,2,2,2,2,2,2,2,2,2,2,2,2,2,2,2,2,2,2,2,2,2,2,2,2,2,2,2,
2,2,2,2,2,2,2,2,2,2,2,2,2,2,2,2,2,2,2,2,2,2,2,4),(-0.991324874888266,-0.976739863257293,
-0.97132404534437,-0.9680718997956,-0.965134788555649,-0.961343670438805,
-0.953231687803036,-0.925996969295892,-0.892901263883769,-0.88755141755747,
-0.885443544004503,-0.883757626556907,-0.881984258502916,-0.879137521470844,
-0.869182132443042,-0.84949895295485,-0.812767132215365,-0.806473074275067,
-0.802700394931127,-0.799757587866313,-0.796528806945328,-0.791221566304062,
-0.769142814089731,-0.740242030405451,-0.723060592501381,-0.719663886134979,
-0.717750497905008,-0.716264597104834,-0.714160638432258,-0.709721983734,
-0.691159604463721,-0.645942161180393,-0.639709908564875,-0.635954908158763,
-0.633014682940957,-0.629777267565902,-0.624428950938107,-0.601620481290346,
-0.570022012622387,-0.556046124880154,-0.552779930235178,-0.55091489918402,
-0.549251997097842,-0.546963887581918,-0.541479622435086,-0.533423736025437,
-0.505566285595962,-0.477117657240083,-0.471450133161718,-0.468144343035572,
-0.465510431747339,-0.46195612249418,-0.455088109869861,-0.430191779750625,
-0.41298779477031,-0.389850134986449,-0.38636068152024,-0.384426670059028,
-0.382778438811334,-0.3806099374494,-0.375821114883758,-0.369111337072889,
-0.349403208019381,-0.312716183273986,-0.306420196159932,-0.302647173907626,
-0.299704566828113,-0.296476480729612,-0.291171488673828,-0.269124112555203,
-0.239561566097529,-0.229557653630966,-0.22164623104683,-0.21893474500181,
-0.217363954288633,-0.215669937024994,-0.213199481235841,-0.206511008517992,
-0.162846542597495,-0.143110644288626,-0.137789571447329,-0.134558234162309,
-0.131616865973127,-0.131487372485602,-0.131362803029669,-0.131242428153373,
-0.131125605603381,-0.131011764075998,-0.127489392331951,-0.118715462853635,
-0.106353615936504,-0.0804420554854634,-0.0565122364423548,-0.0530177863972708,
-0.0510828083351631,-0.0494349514420726,-0.0472685080778907,-0.0424901910055939,
-0.000492539812704547),.UNSPECIFIED.);
#621=B_SPLINE_CURVE_WITH_KNOTS('',3,(#54561,#54562,#54563,#54564,#54565,
#54566,#54567,#54568,#54569,#54570,#54571,#54572,#54573,#54574,#54575,#54576,
#54577,#54578,#54579,#54580),.UNSPECIFIED.,.F.,.F.,(4,2,2,2,2,2,2,2,2,4),
(-2.10003377121719,-2.08459930780237,-2.0760706583423,-2.07213879347443,
-2.06920340574752,-2.06622732444713,-2.0630905739407,-2.05821171241528,
-2.04326789181161,-2.04097989592064),.UNSPECIFIED.);
#622=B_SPLINE_CURVE_WITH_KNOTS('',3,(#54582,#54583,#54584,#54585,#54586,
#54587,#54588,#54589),.UNSPECIFIED.,.F.,.F.,(4,2,2,4),(-0.0594010420905767,
-0.0469797452701944,-0.00923093699204744,-0.000492411924495984),
 .UNSPECIFIED.);
#623=B_SPLINE_CURVE_WITH_KNOTS('',3,(#54590,#54591,#54592,#54593,#54594,
#54595,#54596,#54597,#54598,#54599,#54600,#54601,#54602,#54603,#54604,#54605,
#54606,#54607,#54608,#54609,#54610,#54611,#54612,#54613,#54614,#54615,#54616,
#54617,#54618,#54619,#54620,#54621,#54622,#54623,#54624,#54625,#54626,#54627,
#54628,#54629,#54630,#54631,#54632,#54633,#54634,#54635,#54636,#54637,#54638,
#54639,#54640,#54641,#54642,#54643,#54644,#54645,#54646,#54647,#54648,#54649,
#54650,#54651,#54652,#54653,#54654,#54655,#54656,#54657,#54658,#54659,#54660,
#54661,#54662,#54663,#54664,#54665,#54666,#54667,#54668,#54669,#54670,#54671,
#54672,#54673,#54674,#54675,#54676,#54677,#54678,#54679,#54680,#54681,#54682,
#54683,#54684,#54685,#54686,#54687,#54688,#54689,#54690,#54691,#54692,#54693,
#54694,#54695,#54696,#54697,#54698,#54699,#54700,#54701,#54702,#54703,#54704,
#54705,#54706,#54707,#54708,#54709,#54710,#54711,#54712,#54713,#54714,#54715,
#54716,#54717,#54718,#54719,#54720,#54721,#54722,#54723,#54724,#54725,#54726,
#54727,#54728,#54729,#54730,#54731,#54732,#54733,#54734,#54735,#54736,#54737,
#54738,#54739,#54740,#54741,#54742,#54743,#54744,#54745,#54746,#54747,#54748,
#54749,#54750,#54751,#54752,#54753,#54754,#54755,#54756,#54757,#54758,#54759,
#54760,#54761,#54762,#54763,#54764,#54765,#54766,#54767,#54768,#54769,#54770,
#54771,#54772,#54773,#54774,#54775,#54776,#54777,#54778,#54779,#54780,#54781,
#54782,#54783,#54784,#54785),.UNSPECIFIED.,.F.,.F.,(4,2,2,2,2,2,2,2,2,2,
2,2,2,2,2,2,2,2,2,2,2,2,2,2,2,2,2,2,2,2,2,2,2,2,2,2,2,2,2,2,2,2,2,2,2,2,
2,2,2,2,2,2,2,2,2,2,2,2,2,2,2,2,2,2,2,2,2,2,2,2,2,2,2,2,2,2,2,2,2,2,2,2,
2,2,2,2,2,2,2,2,2,2,2,2,2,2,2,4),(-2.09968458105429,-2.09731412985729,-2.09467903382393,
-2.0919058211916,-2.08880466245833,-2.0840951227781,-2.07059180368999,-2.02615847253882,
-2.01796616203498,-2.01241383089942,-2.0101148004495,-2.0084504287947,-2.0065910758917,
-2.00335035789764,-1.98977461733642,-1.96306696649972,-1.93767331476089,
-1.93074293448994,-1.92717651869468,-1.92454172588388,-1.92124527557621,
-1.91562011309231,-1.88635358662017,-1.8651031661546,-1.85345166798431,
-1.84632420712183,-1.84379431072544,-1.842088833935,-1.8403156444537,-1.83746834126897,
-1.82842234805155,-1.82065795448036,-1.78998778027071,-1.76816706326629,
-1.76287584474351,-1.75965101225839,-1.75670806738825,-1.75293003141391,
-1.74661532366266,-1.71031196095746,-1.69038451391682,-1.6836331638887,
-1.67882189485682,-1.67664955647517,-1.67501590571389,-1.6730911851793,
-1.6696426018293,-1.64991166355826,-1.64356689621778,-1.62300825172028,
-1.60871963610255,-1.59891174835192,-1.59483466261056,-1.59185578800477,
-1.58872432854165,-1.5838707204169,-1.56914958775325,-1.53591074285196,
-1.51657963151166,-1.51205726580885,-1.50993785558262,-1.50845045998029,
-1.50654832081517,-1.50320046929565,-1.48703645491905,-1.45694693675365,
-1.43492761107478,-1.42962457074456,-1.42639719018042,-1.42345492024717,
-1.41968190443652,-1.41338500525859,-1.37677741883421,-1.34843042423717,
-1.3448410194355,-1.34290705708564,-1.34125904080504,-1.33912743065624,
-1.3344151773375,-1.30704854662197,-1.28134086087788,-1.27174066592667,
-1.26442958450656,-1.26078867996609,-1.25789399819178,-1.25456119740361,
-1.24891440363802,-1.21980895362846,-1.19855495402512,-1.18690664084724,
-1.18205561883779,-1.17831599836515,-1.17635071084594,-1.17470628252862,
-1.1725819091216,-1.16803301826951,-1.13701033063592,-1.10891213746094),
 .UNSPECIFIED.);
#624=B_SPLINE_CURVE_WITH_KNOTS('',3,(#54790,#54791,#54792,#54793,#54794,
#54795,#54796,#54797,#54798,#54799,#54800,#54801,#54802,#54803,#54804,#54805,
#54806,#54807,#54808,#54809,#54810,#54811,#54812,#54813,#54814,#54815,#54816,
#54817,#54818,#54819,#54820,#54821,#54822,#54823,#54824,#54825,#54826,#54827,
#54828,#54829,#54830,#54831,#54832,#54833,#54834,#54835,#54836,#54837,#54838,
#54839,#54840,#54841,#54842,#54843,#54844,#54845,#54846,#54847,#54848,#54849,
#54850,#54851,#54852,#54853,#54854,#54855,#54856,#54857,#54858,#54859,#54860,
#54861,#54862,#54863,#54864,#54865,#54866,#54867,#54868,#54869,#54870,#54871,
#54872,#54873,#54874,#54875,#54876,#54877,#54878,#54879,#54880,#54881,#54882,
#54883,#54884,#54885,#54886,#54887,#54888,#54889,#54890,#54891,#54892,#54893,
#54894,#54895,#54896,#54897,#54898,#54899,#54900,#54901,#54902,#54903,#54904,
#54905,#54906,#54907,#54908,#54909,#54910,#54911,#54912,#54913,#54914,#54915,
#54916,#54917,#54918,#54919,#54920,#54921,#54922,#54923,#54924,#54925,#54926,
#54927,#54928,#54929,#54930,#54931,#54932,#54933,#54934,#54935,#54936,#54937,
#54938,#54939,#54940,#54941,#54942,#54943,#54944,#54945,#54946,#54947,#54948,
#54949,#54950,#54951,#54952,#54953,#54954,#54955,#54956,#54957,#54958,#54959,
#54960,#54961,#54962,#54963,#54964,#54965,#54966,#54967,#54968,#54969,#54970,
#54971,#54972,#54973,#54974,#54975,#54976,#54977,#54978,#54979,#54980,#54981,
#54982,#54983,#54984,#54985,#54986,#54987,#54988,#54989,#54990,#54991),
 .UNSPECIFIED.,.F.,.F.,(4,2,2,2,2,2,2,2,2,2,2,2,2,2,2,2,2,2,2,2,2,2,2,2,
2,2,2,2,2,2,2,2,2,2,2,2,2,2,2,2,2,2,2,2,2,2,2,2,2,2,2,2,2,2,2,2,2,2,2,2,
2,2,2,2,2,2,2,2,2,2,2,2,2,2,2,2,2,2,2,2,2,2,2,2,2,2,2,2,2,2,2,2,2,2,2,2,
2,2,2,2,4),(-2.04133053968484,-2.00942223267799,-1.98795143919906,-1.97509604920505,
-1.97112329979462,-1.96807677610341,-1.96512522884565,-1.96129213452401,
-1.95303791682513,-1.91351867964898,-1.89201084448789,-1.8872625944005,
-1.88510121523301,-1.88346821490706,-1.88153512918655,-1.8780506710343,
-1.85643322193555,-1.85233311422696,-1.83213734321064,-1.81743756213607,
-1.80742944091667,-1.8033202825645,-1.80033520078978,-1.79721262807208,
-1.79240431156436,-1.77811853012929,-1.74448730218503,-1.72501198332002,
-1.72047330597303,-1.71835044768818,-1.7168622551832,-1.71496137023007,
-1.71162068632634,-1.69566475339045,-1.66508540409417,-1.64328136065559,
-1.63798983732462,-1.63476427433656,-1.63182031474892,-1.62804049768809,
-1.62172174024913,-1.58543742188698,-1.56548051770844,-1.55872249340508,
-1.55390725974498,-1.55173379183105,-1.5500995775605,-1.5481745458862,-1.54472621542136,
-1.52504269730513,-1.5182229436901,-1.49663901712644,-1.48318900479111,
-1.4737960033512,-1.46978457248824,-1.46681582961828,-1.46366023857543,
-1.45869595479566,-1.44296031706477,-1.4105781386192,-1.39155354968455,
-1.3870636548549,-1.38494992787545,-1.38346280514221,-1.38155582439192,
-1.37818807047584,-1.36158153196709,-1.33198545659644,-1.30992730332048,
-1.30462067555095,-1.30139186559733,-1.29844878149714,-1.29467540227027,
-1.28837945222244,-1.25170717386403,-1.23200708220547,-1.2252987191653,
-1.22051003932177,-1.21834134355003,-1.21669283455972,-1.2147583733192,
-1.21126776474198,-1.18811478769983,-1.17089578437679,-1.14598239922988,
-1.13911178210425,-1.13555659528586,-1.13292224432861,-1.12961615727611,
-1.12394877422018,-1.09320784447763,-1.06947528105522,-1.06034051730432,
-1.05433192601215,-1.05196062056218,-1.05028432022268,-1.04845608644409,
-1.04535946854249,-1.0322681027794,-0.998255818184011,-0.991324874888266),
 .UNSPECIFIED.);
#625=B_SPLINE_CURVE_WITH_KNOTS('',3,(#54992,#54993,#54994,#54995,#54996,
#54997,#54998,#54999,#55000,#55001,#55002,#55003,#55004,#55005,#55006,#55007,
#55008,#55009,#55010,#55011,#55012,#55013,#55014,#55015,#55016,#55017,#55018,
#55019,#55020,#55021,#55022,#55023,#55024,#55025,#55026,#55027,#55028,#55029,
#55030,#55031,#55032,#55033,#55034,#55035,#55036,#55037,#55038,#55039,#55040,
#55041,#55042,#55043,#55044,#55045,#55046,#55047,#55048,#55049,#55050,#55051,
#55052,#55053,#55054,#55055,#55056,#55057,#55058,#55059,#55060,#55061,#55062,
#55063,#55064,#55065,#55066,#55067,#55068,#55069,#55070,#55071,#55072,#55073,
#55074,#55075,#55076,#55077,#55078,#55079,#55080,#55081,#55082,#55083,#55084,
#55085,#55086,#55087,#55088,#55089,#55090,#55091,#55092,#55093,#55094,#55095,
#55096,#55097,#55098,#55099,#55100,#55101,#55102,#55103,#55104,#55105,#55106,
#55107,#55108,#55109,#55110,#55111,#55112,#55113,#55114,#55115,#55116,#55117,
#55118,#55119,#55120,#55121,#55122,#55123,#55124,#55125,#55126,#55127,#55128,
#55129,#55130,#55131,#55132,#55133,#55134,#55135,#55136,#55137,#55138,#55139,
#55140,#55141,#55142,#55143,#55144,#55145,#55146,#55147,#55148,#55149,#55150,
#55151,#55152,#55153,#55154,#55155,#55156,#55157,#55158,#55159,#55160,#55161,
#55162,#55163,#55164,#55165,#55166,#55167,#55168,#55169,#55170,#55171,#55172,
#55173,#55174,#55175,#55176,#55177,#55178,#55179,#55180,#55181,#55182,#55183,
#55184,#55185,#55186,#55187,#55188,#55189,#55190,#55191,#55192,#55193,#55194,
#55195,#55196,#55197,#55198,#55199,#55200,#55201),.UNSPECIFIED.,.F.,.F.,
(4,2,2,2,2,2,2,2,2,2,2,2,2,2,2,2,2,2,2,2,2,2,2,2,2,2,2,2,2,2,2,2,2,2,2,
2,2,2,2,2,2,2,2,2,2,2,2,2,2,2,2,2,2,2,2,2,2,2,2,2,2,2,2,2,2,2,2,2,2,2,2,
2,2,2,2,2,2,2,2,2,2,2,2,2,2,2,2,2,2,2,2,2,2,2,2,2,2,2,2,2,2,2,2,2,4),(-1.10891213746094,
-1.1025633642418,-1.09675596498821,-1.09342079918388,-1.09049873079705,
-1.08684784268661,-1.07972500987875,-1.04984946772662,-1.01641280378912,
-1.01203215014507,-1.00993950979549,-1.00829694968953,-1.00630630431078,
-1.00244296863831,-0.997382484187126,-0.984949815622372,-0.947137552229913,
-0.933764272117823,-0.92905725596907,-0.925956683426332,-0.922960333752754,
-0.918782528297241,-0.908315985064879,-0.892645539132459,-0.863007997155038,
-0.848033052976157,-0.844754056027536,-0.842867547764913,-0.841210837261998,
-0.838965284184677,-0.833734379988036,-0.826179421124063,-0.801678757061201,
-0.77165171134716,-0.764535389508557,-0.76088589450098,-0.757964011777495,
-0.754628051859136,-0.748816601694433,-0.741684943745739,-0.725990412548922,
-0.696612974909208,-0.68143520548209,-0.678146421345032,-0.676257694871797,
-0.67460150521706,-0.672359971784562,-0.667152730616636,-0.659643961682607,
-0.635430963657303,-0.605008980703444,-0.597909140214804,-0.594263036266875,
-0.591341421426077,-0.588003111309202,-0.582180588827743,-0.547717074415929,
-0.516788018608673,-0.512232779815384,-0.510107292827893,-0.508462856755302,
-0.506498606252927,-0.502763688836621,-0.497920003563948,-0.486298037287833,
-0.464995829294303,-0.435862159743072,-0.430214682084528,-0.426881836216722,
-0.423987334639317,-0.420346945837214,-0.413037846239776,-0.403442054520717,
-0.377751919203769,-0.350404162156482,-0.345692216817802,-0.343560764867445,
-0.341912862038218,-0.339979054060065,-0.33638993902098,-0.307783451178721,
-0.271435876720952,-0.265122102020854,-0.261344529032147,-0.25840187089686,
-0.255177276220613,-0.249886250283688,-0.228057817584104,-0.197351102087575,
-0.181589326238876,-0.178268193931256,-0.176372201113465,-0.174717731899929,
-0.172489337486825,-0.167358551905306,-0.159998141976578,-0.136685618662079,
-0.105083823888635,-0.0979982857234888,-0.0943552260900261,-0.0914339671919788,
-0.0880937989132507,-0.0822620718678626,-0.0750984618859152,-0.0593641111093442),
 .UNSPECIFIED.);
#626=B_SPLINE_CURVE_WITH_KNOTS('',3,(#55207,#55208,#55209,#55210,#55211,
#55212,#55213,#55214,#55215,#55216,#55217,#55218,#55219,#55220,#55221,#55222,
#55223,#55224,#55225,#55226,#55227,#55228,#55229,#55230,#55231,#55232,#55233,
#55234,#55235,#55236,#55237,#55238,#55239,#55240,#55241,#55242,#55243,#55244,
#55245,#55246,#55247,#55248,#55249,#55250,#55251,#55252,#55253,#55254,#55255,
#55256,#55257,#55258,#55259,#55260,#55261,#55262,#55263,#55264,#55265,#55266,
#55267,#55268,#55269,#55270,#55271,#55272,#55273,#55274,#55275,#55276,#55277,
#55278,#55279,#55280,#55281,#55282,#55283,#55284,#55285,#55286,#55287,#55288,
#55289,#55290,#55291,#55292,#55293,#55294,#55295,#55296,#55297,#55298,#55299,
#55300,#55301,#55302,#55303,#55304,#55305,#55306,#55307,#55308,#55309,#55310,
#55311,#55312,#55313,#55314,#55315,#55316,#55317,#55318,#55319,#55320,#55321,
#55322,#55323,#55324,#55325,#55326,#55327,#55328,#55329,#55330,#55331,#55332,
#55333,#55334,#55335,#55336,#55337,#55338,#55339,#55340,#55341,#55342,#55343,
#55344,#55345,#55346,#55347,#55348,#55349,#55350,#55351,#55352,#55353,#55354,
#55355,#55356,#55357,#55358,#55359,#55360,#55361,#55362,#55363,#55364,#55365,
#55366,#55367,#55368,#55369,#55370,#55371,#55372),.UNSPECIFIED.,.F.,.F.,
(4,3,3,3,3,3,3,3,3,3,3,3,3,3,3,3,3,3,3,3,3,3,3,3,3,3,3,3,3,3,3,3,3,3,3,
3,3,3,3,3,3,3,3,3,3,3,3,3,3,3,3,3,3,3,3,4),(45.6442294067315,45.755562043948,
45.8671127049469,45.8863125840836,45.9961074696102,46.107074175724,46.2165666038188,
46.3259920438982,46.4353911890671,46.5475036714304,46.6570424939021,46.7704418062112,
46.8838411185202,46.9936360040466,47.1046027101604,47.2140951382552,47.3235205783346,
47.4329197235036,47.5450322058669,47.6545710283387,47.7679703406478,47.8813696529568,
47.9911645384834,48.1021312445971,48.211623672692,48.3210491127715,48.4304482579405,
48.5425607403037,48.6520995627755,48.7654988750845,48.8788981873934,48.9886930729199,
49.0996597790337,49.2091522071285,49.3185776472081,49.4279767923771,49.5400892747403,
49.649628097212,49.763027409521,49.87642672183,49.9862216073565,50.0971883134703,
50.2066807415652,50.3161061816448,50.4255053268137,50.5376178091769,50.6471566316488,
50.7605559439577,50.8739552562666,50.9830326905725,51.0919496345074,51.2007480886016,
51.3094873290939,51.418191872754,51.5269441665217,51.5753047126086),
 .UNSPECIFIED.);
#627=B_SPLINE_CURVE_WITH_KNOTS('',3,(#55373,#55374,#55375,#55376,#55377,
#55378,#55379,#55380,#55381,#55382,#55383,#55384,#55385,#55386,#55387,#55388,
#55389,#55390),.UNSPECIFIED.,.F.,.F.,(4,2,2,2,2,2,2,2,4),(-2.10014213462196,
-2.06257558601288,-2.05743286849352,-2.05352065982169,-2.05151969222044,
-2.04987707829303,-2.04779506593583,-2.04347211109637,-2.04133053968484),
 .UNSPECIFIED.);
#628=B_SPLINE_CURVE_WITH_KNOTS('',3,(#55392,#55393,#55394,#55395,#55396,
#55397,#55398,#55399,#55400,#55401,#55402,#55403,#55404,#55405,#55406,#55407,
#55408,#55409,#55410,#55411),.UNSPECIFIED.,.F.,.F.,(4,2,2,2,2,2,2,2,2,4),
(-0.0593641111093442,-0.0592945763534438,-0.0244898707930381,-0.014250358420362,
-0.0112791011793178,-0.00947879736946485,-0.00791757388433898,-0.00623963099242318,
-0.00362518939908151,-0.000491822792723786),.UNSPECIFIED.);
#629=B_SPLINE_CURVE_WITH_KNOTS('',3,(#55412,#55413,#55414,#55415,#55416,
#55417,#55418,#55419,#55420,#55421,#55422,#55423,#55424,#55425,#55426,#55427,
#55428,#55429,#55430,#55431,#55432,#55433,#55434,#55435,#55436,#55437,#55438,
#55439,#55440,#55441,#55442,#55443,#55444,#55445,#55446,#55447,#55448,#55449,
#55450,#55451,#55452,#55453,#55454,#55455,#55456,#55457,#55458,#55459,#55460,
#55461,#55462,#55463,#55464,#55465,#55466,#55467,#55468,#55469,#55470,#55471,
#55472,#55473,#55474,#55475,#55476,#55477,#55478,#55479,#55480,#55481,#55482,
#55483,#55484,#55485,#55486,#55487,#55488,#55489,#55490,#55491,#55492,#55493,
#55494,#55495,#55496,#55497,#55498,#55499,#55500,#55501,#55502,#55503,#55504,
#55505,#55506,#55507,#55508,#55509,#55510,#55511,#55512,#55513,#55514,#55515,
#55516,#55517,#55518,#55519,#55520,#55521,#55522,#55523,#55524,#55525,#55526,
#55527,#55528,#55529,#55530,#55531,#55532,#55533,#55534,#55535,#55536,#55537,
#55538,#55539,#55540,#55541,#55542,#55543,#55544,#55545,#55546,#55547,#55548,
#55549,#55550,#55551,#55552,#55553,#55554,#55555,#55556,#55557,#55558,#55559,
#55560,#55561,#55562,#55563,#55564,#55565,#55566,#55567,#55568,#55569,#55570,
#55571,#55572,#55573,#55574,#55575,#55576,#55577,#55578,#55579,#55580,#55581,
#55582,#55583,#55584,#55585,#55586,#55587,#55588,#55589,#55590,#55591,#55592,
#55593,#55594,#55595,#55596,#55597,#55598,#55599,#55600,#55601,#55602,#55603,
#55604,#55605,#55606,#55607,#55608,#55609,#55610,#55611,#55612,#55613,#55614,
#55615,#55616,#55617,#55618,#55619,#55620,#55621,#55622,#55623,#55624,#55625,
#55626,#55627,#55628,#55629,#55630,#55631,#55632,#55633,#55634,#55635,#55636,
#55637,#55638,#55639,#55640,#55641,#55642,#55643,#55644,#55645,#55646,#55647,
#55648,#55649,#55650,#55651,#55652,#55653,#55654,#55655,#55656,#55657,#55658,
#55659,#55660,#55661,#55662,#55663,#55664,#55665,#55666,#55667,#55668,#55669,
#55670,#55671),.UNSPECIFIED.,.F.,.F.,(4,2,2,2,2,2,2,2,2,2,2,2,2,2,2,2,2,
2,2,2,2,2,2,2,2,2,2,2,2,2,2,2,2,2,2,2,2,2,2,2,2,2,2,2,2,2,2,2,2,2,2,2,2,
2,2,2,2,2,2,2,2,2,2,2,2,2,2,2,2,2,2,2,2,2,2,2,2,2,2,2,2,2,2,2,2,2,2,2,2,
2,2,2,2,2,2,2,2,2,2,2,2,2,2,2,2,2,2,2,2,2,2,2,2,2,2,2,2,2,2,2,2,2,2,2,2,
2,2,2,2,4),(-2.10006909147699,-2.06042698248811,-2.03980647629323,-2.03146648594754,
-2.02763510315893,-2.02469359950251,-2.02146337858658,-2.01614706804224,
-1.9962000499577,-1.95269366760667,-1.94816988454401,-1.9456127155445,-1.94345601991161,
-1.94343583567694,-1.94341562285936,-1.94339537552586,-1.94337508765153,
-1.94335475310606,-1.94333436565094,-1.94332346393289,-1.94331229026595,
-1.94330083104297,-1.94328907174349,-1.94327699684956,-1.94326458976273,
-1.94325183269404,-1.94323870656951,-1.94322519089653,-1.94321126362617,
-1.94319690099945,-1.94318207737893,-1.94316676504375,-1.94315093398021,
-1.94313455162251,-1.94311758257521,-1.94309998828557,-1.94308172667756,
-1.94306275172435,-1.94304301296563,-1.94302245494273,-1.94300101655145,
-1.94297863027483,-1.94295522130587,-1.94293070650797,-1.9429049931827,
-1.94287797761661,-1.94284954334717,-1.94281955908304,-1.94278787619298,
-1.94275432565812,-1.94271871433806,-1.94268082036658,-1.9426509704841,
-1.94106261086972,-1.93892177710552,-1.93415824915268,-1.90981690568386,
-1.88889157001418,-1.86796294276235,-1.86272692591118,-1.85951375564633,
-1.85656712836847,-1.85276434150927,-1.8443535857145,-1.80489322408999,
-1.7834167699023,-1.7786722163301,-1.77651177960524,-1.77487916580743,-1.77294613552,
-1.76946084057255,-1.74764142224433,-1.72666562914355,-1.70171666859176,
-1.69626138724263,-1.69300111494656,-1.69006638979896,-1.68629198979989,
-1.68013322697073,-1.64170984436539,-1.61505485131496,-1.61138390437407,
-1.60943272697357,-1.60778665110324,-1.6056782471193,-1.60109476798526,
-1.57036777474382,-1.53571154464025,-1.52987941141069,-1.52653873141973,
-1.52361687344045,-1.5199728666579,-1.51288480756635,-1.48151926610307,
-1.45804627885887,-1.45065909735514,-1.44551377912789,-1.4432826365378,
-1.44162754666876,-1.4397325201904,-1.43641660695055,-1.42071035358183,
-1.38992362895068,-1.36806146041605,-1.36276742635263,-1.35954181364691,
-1.35659876059069,-1.35282142280912,-1.34650978290014,-1.31013975697264,
-1.2815396563814,-1.27797123007123,-1.27604159322631,-1.27439280202657,
-1.27225456611438,-1.26750592928128,-1.24199245658235,-1.21960968147045,
-1.20721341351749,-1.19836180926394,-1.19444110580818,-1.19148686272814,
-1.18829666656338,-1.18316827059753,-1.16617833419779,-1.13421088682827,
-1.11620325570252,-1.11182720358427,-1.10973528143656,-1.10915292416611),
 .UNSPECIFIED.);
#630=B_SPLINE_CURVE_WITH_KNOTS('',3,(#55677,#55678,#55679,#55680,#55681,
#55682,#55683,#55684,#55685,#55686,#55687,#55688,#55689,#55690,#55691,#55692,
#55693,#55694,#55695,#55696,#55697,#55698,#55699,#55700,#55701,#55702,#55703,
#55704,#55705,#55706,#55707,#55708,#55709,#55710,#55711,#55712,#55713,#55714,
#55715,#55716,#55717,#55718,#55719,#55720,#55721,#55722,#55723,#55724,#55725,
#55726,#55727,#55728,#55729,#55730,#55731,#55732,#55733,#55734,#55735,#55736,
#55737,#55738,#55739,#55740,#55741,#55742,#55743,#55744,#55745,#55746,#55747,
#55748,#55749,#55750,#55751,#55752,#55753,#55754,#55755,#55756,#55757,#55758,
#55759,#55760,#55761,#55762,#55763,#55764,#55765,#55766,#55767,#55768,#55769,
#55770,#55771,#55772,#55773,#55774,#55775,#55776,#55777,#55778,#55779,#55780,
#55781,#55782,#55783,#55784,#55785,#55786,#55787,#55788,#55789,#55790,#55791,
#55792,#55793,#55794,#55795,#55796,#55797,#55798,#55799,#55800,#55801,#55802,
#55803,#55804,#55805,#55806,#55807,#55808,#55809,#55810,#55811,#55812,#55813,
#55814,#55815,#55816,#55817,#55818,#55819,#55820,#55821,#55822,#55823,#55824,
#55825,#55826,#55827,#55828,#55829,#55830,#55831,#55832,#55833,#55834,#55835,
#55836,#55837,#55838,#55839,#55840,#55841,#55842,#55843,#55844,#55845,#55846,
#55847,#55848,#55849,#55850,#55851,#55852,#55853,#55854,#55855,#55856,#55857,
#55858,#55859,#55860,#55861,#55862,#55863,#55864,#55865,#55866,#55867,#55868,
#55869,#55870,#55871,#55872,#55873,#55874),.UNSPECIFIED.,.F.,.F.,(4,2,2,
2,2,2,2,2,2,2,2,2,2,2,2,2,2,2,2,2,2,2,2,2,2,2,2,2,2,2,2,2,2,2,2,2,2,2,2,
2,2,2,2,2,2,2,2,2,2,2,2,2,2,2,2,2,2,2,2,2,2,2,2,2,2,2,2,2,2,2,2,2,2,2,2,
2,2,2,2,2,2,2,2,2,2,2,2,2,2,2,2,2,2,2,2,2,2,2,4),(-0.991222341842758,-0.988736115830365,
-0.985429716872542,-0.982795938841155,-0.979242614379858,-0.97237936274641,
-0.947519773672175,-0.930290479672997,-0.907134999625649,-0.903645530734768,
-0.901711534824292,-0.900063332870706,-0.897894891023519,-0.893106279894226,
-0.886396860354405,-0.866690331178903,-0.830001964819376,-0.823706201888839,
-0.819933275710456,-0.816990721566128,-0.813762671172812,-0.808457685745978,
-0.786409302719088,-0.756874383810196,-0.747473952614986,-0.739061707527578,
-0.736287968513925,-0.734704989278039,-0.733019983597198,-0.730597830420924,
-0.724247191690939,-0.714373236978621,-0.692675034975813,-0.661142621969833,
-0.655506115389764,-0.652175401548015,-0.649280127069679,-0.645635326646925,
-0.638305155457721,-0.62867351816379,-0.602809969022405,-0.57570419916963,
-0.570981310248147,-0.568847690715342,-0.567199351129337,-0.565266535647471,
-0.561683013099233,-0.55709150769755,-0.513350292512699,-0.493703961778137,
-0.488402931426541,-0.485175984463718,-0.482233604856421,-0.478395525181586,
-0.47001767855272,-0.447878611317424,-0.40878714859733,-0.404208972333476,
-0.402079171605349,-0.400434372151114,-0.398473261013458,-0.394753734461102,
-0.389935915374499,-0.378409162882555,-0.357003699504285,-0.327747189498164,
-0.322071754712161,-0.318764586794498,-0.316131316457517,-0.31258013407555,
-0.305726186973548,-0.280935442020369,-0.263662120324144,-0.240476898439039,
-0.236987752763299,-0.235053980647722,-0.233405999141088,-0.231237886185148,
-0.226450149586381,-0.219742070273756,-0.200040491879911,-0.163350076492882,
-0.15705717722147,-0.153285322170092,-0.150426831357105,-0.147370968562231,
-0.143046309003511,-0.137612748193346,-0.127188487944933,-0.10056308469208,
-0.0980535496024327,-0.0738493315394838,-0.0703514591928269,-0.0684157770337268,
-0.0667681107699831,-0.0646029501361435,-0.0598313828507849,-0.0380777263262519,
-0.000492602108507802),.UNSPECIFIED.);
#631=B_SPLINE_CURVE_WITH_KNOTS('',3,(#55875,#55876,#55877,#55878,#55879,
#55880,#55881,#55882,#55883,#55884,#55885,#55886,#55887),.UNSPECIFIED.,
 .F.,.F.,(4,3,3,3,4),(45.292119405429,45.4031325580051,45.5141760165917,
45.6253344673629,45.6442294067315),.UNSPECIFIED.);
#632=B_SPLINE_CURVE_WITH_KNOTS('',3,(#55888,#55889,#55890,#55891,#55892,
#55893,#55894,#55895,#55896,#55897,#55898,#55899,#55900,#55901,#55902,#55903,
#55904,#55905,#55906,#55907,#55908,#55909,#55910,#55911,#55912,#55913,#55914,
#55915,#55916,#55917,#55918,#55919,#55920,#55921,#55922,#55923,#55924,#55925,
#55926,#55927,#55928,#55929,#55930,#55931,#55932,#55933,#55934,#55935,#55936,
#55937,#55938,#55939,#55940,#55941,#55942,#55943,#55944,#55945,#55946,#55947,
#55948,#55949,#55950,#55951,#55952,#55953,#55954,#55955,#55956,#55957,#55958,
#55959,#55960,#55961,#55962,#55963,#55964,#55965,#55966,#55967,#55968,#55969,
#55970,#55971,#55972,#55973,#55974,#55975,#55976,#55977,#55978,#55979,#55980,
#55981,#55982,#55983,#55984,#55985,#55986,#55987,#55988,#55989,#55990,#55991,
#55992,#55993,#55994,#55995,#55996,#55997,#55998,#55999,#56000,#56001,#56002,
#56003,#56004,#56005,#56006,#56007,#56008,#56009,#56010,#56011,#56012,#56013,
#56014,#56015,#56016,#56017,#56018,#56019,#56020,#56021,#56022,#56023,#56024,
#56025,#56026,#56027,#56028,#56029,#56030,#56031,#56032,#56033,#56034,#56035,
#56036,#56037,#56038,#56039,#56040,#56041,#56042,#56043,#56044,#56045,#56046,
#56047,#56048,#56049,#56050,#56051,#56052,#56053,#56054,#56055,#56056,#56057,
#56058,#56059,#56060,#56061,#56062,#56063,#56064,#56065,#56066,#56067,#56068,
#56069,#56070,#56071,#56072,#56073,#56074,#56075,#56076,#56077,#56078,#56079,
#56080,#56081,#56082,#56083,#56084,#56085,#56086,#56087,#56088,#56089,#56090,
#56091,#56092,#56093),.UNSPECIFIED.,.F.,.F.,(4,2,2,2,2,2,2,2,2,2,2,2,2,
2,2,2,2,2,2,2,2,2,2,2,2,2,2,2,2,2,2,2,2,2,2,2,2,2,2,2,2,2,2,2,2,2,2,2,2,
2,2,2,2,2,2,2,2,2,2,2,2,2,2,2,2,2,2,2,2,2,2,2,2,2,2,2,2,2,2,2,2,2,2,2,2,
2,2,2,2,2,2,2,2,2,2,2,2,2,2,2,2,2,4),(-1.10915292416611,-1.10825079081598,
-1.1063292457688,-1.10289549192893,-1.08373122537149,-1.05032496968337,
-1.034182926507,-1.02917413652272,-1.02600957642963,-1.02304572664456,-1.0190614413913,
-1.00983003115074,-0.996699510755589,-0.974812585359114,-0.969892933399924,
-0.948188552366218,-0.944704778830646,-0.942772132535236,-0.941139560443809,
-0.938978777311095,-0.934232014918134,-0.912731628609526,-0.873210557968264,
-0.86494358154075,-0.861108709719495,-0.85815753172259,-0.854959575707928,
-0.849793919947537,-0.8299010179121,-0.808108115825579,-0.80243886498364,
-0.781526984439174,-0.778053098808981,-0.776122729579546,-0.77448995192073,
-0.772326122139348,-0.767562066886004,-0.745884970981147,-0.705803009331144,
-0.697938340202351,-0.694193146788012,-0.691262126798466,-0.687986381573837,
-0.682457315225892,-0.655683597708827,-0.616535719565333,-0.611970389837679,
-0.609843019397428,-0.608198443177589,-0.606235604667619,-0.602507540321231,
-0.597675354062329,-0.586095646882868,-0.564748692695435,-0.53552226810327,
-0.529847010859261,-0.526539953097078,-0.523906770614772,-0.52035570345531,
-0.513501949899647,-0.488711339626953,-0.471441110104947,-0.448259215918448,
-0.444770263564931,-0.442836574476547,-0.441188643516863,-0.43902055935761,
-0.434232728108947,-0.427524365655815,-0.407820441283542,-0.371143199941577,
-0.364848511758308,-0.361076221795289,-0.358134154423512,-0.354906625022364,
-0.34960245615806,-0.327556027713085,-0.29809201700578,-0.290151711519928,
-0.280500342728967,-0.277587680632365,-0.275800206820813,-0.274104153945243,
-0.27162191162735,-0.264846607656808,-0.254018215977439,-0.232211835145648,
-0.204762088487403,-0.197717886763157,-0.194083215877829,-0.191162420136257,
-0.187815947342846,-0.181955129649531,-0.148651351729641,-0.116513062467537,
-0.112089796990142,-0.109981402893426,-0.108335548915263,-0.106384922637174,
-0.102715710338574,-0.0979818938659247,-0.086760354592038,-0.0595119917279155),
 .UNSPECIFIED.);
#633=B_SPLINE_CURVE_WITH_KNOTS('',3,(#56098,#56099,#56100,#56101,#56102,
#56103,#56104,#56105,#56106,#56107,#56108,#56109,#56110,#56111,#56112,#56113,
#56114,#56115,#56116,#56117,#56118,#56119,#56120,#56121,#56122,#56123,#56124,
#56125,#56126,#56127,#56128,#56129,#56130,#56131,#56132,#56133,#56134,#56135,
#56136,#56137,#56138,#56139,#56140,#56141,#56142,#56143,#56144,#56145,#56146,
#56147,#56148,#56149,#56150,#56151,#56152,#56153,#56154,#56155,#56156,#56157,
#56158,#56159,#56160,#56161,#56162,#56163,#56164,#56165,#56166,#56167,#56168,
#56169,#56170,#56171,#56172,#56173,#56174,#56175,#56176,#56177,#56178,#56179,
#56180,#56181,#56182,#56183,#56184,#56185,#56186,#56187,#56188,#56189,#56190,
#56191,#56192,#56193,#56194,#56195,#56196,#56197,#56198,#56199,#56200,#56201,
#56202,#56203,#56204,#56205,#56206,#56207,#56208,#56209,#56210,#56211,#56212,
#56213,#56214,#56215,#56216,#56217,#56218,#56219,#56220,#56221,#56222,#56223,
#56224,#56225,#56226,#56227,#56228,#56229,#56230,#56231,#56232,#56233,#56234,
#56235,#56236,#56237,#56238,#56239,#56240,#56241,#56242,#56243,#56244,#56245,
#56246,#56247,#56248,#56249,#56250,#56251,#56252,#56253,#56254,#56255,#56256,
#56257,#56258,#56259,#56260,#56261,#56262,#56263,#56264,#56265,#56266,#56267,
#56268,#56269,#56270,#56271,#56272,#56273,#56274,#56275,#56276,#56277,#56278,
#56279,#56280,#56281,#56282,#56283,#56284,#56285,#56286,#56287,#56288,#56289,
#56290,#56291,#56292,#56293,#56294,#56295),.UNSPECIFIED.,.F.,.F.,(4,2,2,
2,2,2,2,2,2,2,2,2,2,2,2,2,2,2,2,2,2,2,2,2,2,2,2,2,2,2,2,2,2,2,2,2,2,2,2,
2,2,2,2,2,2,2,2,2,2,2,2,2,2,2,2,2,2,2,2,2,2,2,2,2,2,2,2,2,2,2,2,2,2,2,2,
2,2,2,2,2,2,2,2,2,2,2,2,2,2,2,2,2,2,2,2,2,2,2,4),(-2.04125292518874,-2.03894385906771,
-2.0086167602156,-1.9987512842822,-1.99063901794145,-1.98680858232649,-1.98386672724615,
-1.98063505013605,-1.97531385257718,-1.95529170396841,-1.91182131686073,
-1.90522195471023,-1.90276389947667,-1.90107210296551,-1.89949808281679,
-1.89677059908336,-1.88873496970261,-1.87884691711931,-1.84929135617849,
-1.82723320617522,-1.82192692860413,-1.81869837618869,-1.8157555554526,
-1.81198255346591,-1.805687322463,-1.76901551993487,-1.74931893601361,-1.7426115061407,
-1.73782343040583,-1.735654957439,-1.73400659546301,-1.73207228034356,-1.72858187445159,
-1.70540462604948,-1.68815013902088,-1.66329142738332,-1.65642812632849,
-1.65287458858188,-1.6502405978268,-1.64693384168821,-1.64126246351765,
-1.61146634867061,-1.58996633424274,-1.57885772947006,-1.57415475056505,
-1.57050358363136,-1.56855643539007,-1.56690974422363,-1.56479554535921,
-1.56018091462033,-1.5212275442612,-1.49428882348829,-1.48875217555391,
-1.48547435892506,-1.48254298373868,-1.47879940539059,-1.47094602709401,
-1.43086114350963,-1.40918592963673,-1.40442145407425,-1.40225729315876,
-1.4006241911428,-1.39869339030437,-1.39521856928128,-1.37431388654119,
-1.3693983096508,-1.35200433253846,-1.32741732477023,-1.32197815909426,
-1.31872113395761,-1.3157853426765,-1.31200397973758,-1.30582179682574,
-1.2603921976727,-1.24195914797297,-1.23753472188651,-1.23543340192903,
-1.23394771856894,-1.23203233495851,-1.22862692917518,-1.2105229577108,
-1.16505843700595,-1.15697142647289,-1.15318503265454,-1.15024872501543,
-1.14699457244317,-1.14156845026328,-1.11988391122826,-1.08606896867069,
-1.07728730461913,-1.07144720620063,-1.0691021411999,-1.0674303954053,-1.06559159566497,
-1.06244592629941,-1.05027315976444,-1.0243561927847,-0.994406655279623,
-0.991222341842758),.UNSPECIFIED.);
#634=B_SPLINE_CURVE_WITH_KNOTS('',3,(#56297,#56298,#56299,#56300,#56301,
#56302,#56303,#56304,#56305,#56306,#56307,#56308,#56309,#56310,#56311,#56312,
#56313,#56314,#56315,#56316),.UNSPECIFIED.,.F.,.F.,(4,2,2,2,2,2,2,2,2,4),
(-0.0595119917279155,-0.0586930344537183,-0.0373482121527803,-0.0313487865350335,
-0.0276208962624948,-0.0246916304183028,-0.0219520084146087,-0.0187213524838508,
-0.0116698606299128,-0.000491772399311334),.UNSPECIFIED.);
#635=B_SPLINE_CURVE_WITH_KNOTS('',3,(#56317,#56318,#56319,#56320,#56321,
#56322,#56323,#56324,#56325,#56326,#56327,#56328,#56329,#56330,#56331,#56332,
#56333,#56334,#56335,#56336,#56337,#56338,#56339,#56340,#56341,#56342,#56343,
#56344,#56345,#56346,#56347,#56348,#56349,#56350,#56351,#56352,#56353,#56354,
#56355,#56356,#56357,#56358,#56359,#56360,#56361,#56362,#56363,#56364,#56365,
#56366,#56367,#56368,#56369,#56370,#56371,#56372,#56373,#56374,#56375,#56376,
#56377,#56378,#56379,#56380,#56381,#56382,#56383,#56384,#56385,#56386,#56387,
#56388,#56389,#56390,#56391,#56392,#56393,#56394,#56395,#56396,#56397,#56398,
#56399,#56400,#56401,#56402,#56403,#56404,#56405,#56406,#56407,#56408,#56409,
#56410,#56411,#56412,#56413,#56414,#56415,#56416,#56417,#56418,#56419,#56420,
#56421,#56422,#56423,#56424,#56425,#56426,#56427,#56428,#56429,#56430,#56431,
#56432,#56433,#56434,#56435,#56436,#56437,#56438,#56439,#56440,#56441,#56442,
#56443,#56444,#56445,#56446,#56447,#56448,#56449,#56450,#56451,#56452,#56453,
#56454,#56455,#56456,#56457,#56458,#56459,#56460,#56461,#56462,#56463,#56464,
#56465,#56466,#56467,#56468,#56469,#56470,#56471,#56472,#56473,#56474,#56475,
#56476,#56477,#56478,#56479,#56480,#56481,#56482,#56483,#56484,#56485,#56486,
#56487,#56488,#56489,#56490,#56491,#56492,#56493,#56494,#56495,#56496,#56497,
#56498,#56499,#56500,#56501,#56502,#56503,#56504,#56505,#56506,#56507,#56508),
 .UNSPECIFIED.,.F.,.F.,(4,2,2,2,2,2,2,2,2,2,2,2,2,2,2,2,2,2,2,2,2,2,2,2,
2,2,2,2,2,2,2,2,2,2,2,2,2,2,2,2,2,2,2,2,2,2,2,2,2,2,2,2,2,2,2,2,2,2,2,2,
2,2,2,2,2,2,2,2,2,2,2,2,2,2,2,2,2,2,2,2,2,2,2,2,2,2,2,2,2,2,2,2,2,2,2,4),
(-2.09985264300038,-2.07634126040968,-2.0477689920784,-2.04419976479163,
-2.04226962137628,-2.04062035027246,-2.03848143268273,-2.03390404652844,
-2.00367752407994,-1.97990014181989,-1.97070510626822,-1.96369652470103,
-1.96018700760897,-1.95731214266405,-1.95400536132066,-1.94833536546717,
-1.91899508832036,-1.89188103455156,-1.88393026275446,-1.87849779140609,
-1.87621791806677,-1.87455590342492,-1.87268611498573,-1.86939907698012,
-1.8550482065297,-1.82377445548619,-1.80100035802833,-1.79565283567918,
-1.79241516797978,-1.78947425041419,-1.78571772784181,-1.77948155930131,
-1.7419519284354,-1.71468113426106,-1.71091699538094,-1.70894621044565,
-1.70730159572318,-1.70518264378745,-1.70066528096452,-1.66924956737454,
-1.63516145693111,-1.62932990872132,-1.62598885726903,-1.62306626476174,
-1.61942080460461,-1.61232818849689,-1.58125977909918,-1.55754893325383,
-1.55012152043423,-1.54495513727622,-1.54272006680958,-1.54106416116889,
-1.53917061969497,-1.53586246591984,-1.52030333385083,-1.491369123967,-1.47561549844014,
-1.46846572503323,-1.46264273169486,-1.45930353940011,-1.45638080715795,
-1.45273285379155,-1.44562790888823,-1.41536663362571,-1.39104426208925,
-1.38351736472024,-1.37829988427577,-1.37605612779594,-1.37439914198933,
-1.37251052066494,-1.36922399137595,-1.35411744860148,-1.32460582471591,
-1.30890549408723,-1.30177142889655,-1.29595846626567,-1.29262145640245,
-1.2896985584405,-1.28604766821214,-1.27892817879026,-1.24896296684978,
-1.22442902039424,-1.21318670327752,-1.21022695482445,-1.20842874223766,
-1.20675744247451,-1.20470659342738,-1.20067066639486,-1.16834932325329,
-1.13513191413727,-1.12928549372802,-1.12594145994443,-1.12301946258418,
-1.11937894018971,-1.11230940815688,-1.10892217029559),.UNSPECIFIED.);
#636=B_SPLINE_CURVE_WITH_KNOTS('',3,(#56514,#56515,#56516,#56517,#56518,
#56519,#56520,#56521,#56522,#56523,#56524,#56525,#56526,#56527,#56528,#56529,
#56530,#56531,#56532,#56533,#56534,#56535,#56536,#56537,#56538,#56539,#56540,
#56541,#56542,#56543,#56544,#56545,#56546,#56547,#56548,#56549,#56550,#56551,
#56552,#56553,#56554,#56555,#56556,#56557,#56558,#56559,#56560,#56561,#56562,
#56563,#56564,#56565,#56566,#56567,#56568,#56569,#56570,#56571,#56572,#56573,
#56574,#56575,#56576,#56577,#56578,#56579,#56580,#56581,#56582,#56583,#56584,
#56585,#56586,#56587,#56588,#56589,#56590,#56591,#56592,#56593,#56594,#56595,
#56596,#56597,#56598,#56599,#56600,#56601,#56602,#56603,#56604,#56605,#56606,
#56607,#56608,#56609,#56610,#56611,#56612,#56613,#56614,#56615,#56616,#56617,
#56618,#56619,#56620,#56621,#56622,#56623,#56624,#56625,#56626,#56627,#56628,
#56629,#56630,#56631,#56632,#56633,#56634,#56635,#56636,#56637,#56638,#56639,
#56640,#56641,#56642,#56643,#56644,#56645,#56646,#56647,#56648,#56649,#56650,
#56651,#56652,#56653,#56654,#56655,#56656,#56657,#56658,#56659,#56660,#56661,
#56662,#56663,#56664,#56665,#56666,#56667,#56668,#56669,#56670,#56671,#56672,
#56673,#56674,#56675,#56676,#56677,#56678,#56679,#56680,#56681,#56682,#56683,
#56684,#56685,#56686,#56687,#56688,#56689,#56690,#56691,#56692,#56693,#56694,
#56695,#56696,#56697,#56698,#56699,#56700,#56701,#56702,#56703,#56704,#56705,
#56706,#56707,#56708,#56709,#56710,#56711),.UNSPECIFIED.,.F.,.F.,(4,2,2,
2,2,2,2,2,2,2,2,2,2,2,2,2,2,2,2,2,2,2,2,2,2,2,2,2,2,2,2,2,2,2,2,2,2,2,2,
2,2,2,2,2,2,2,2,2,2,2,2,2,2,2,2,2,2,2,2,2,2,2,2,2,2,2,2,2,2,2,2,2,2,2,2,
2,2,2,2,2,2,2,2,2,2,2,2,2,2,2,2,2,2,2,2,2,2,2,4),(-0.991342359623623,-0.975835741061672,
-0.971794971303946,-0.969743212814923,-0.968072009170711,-0.966275028603975,
-0.963319374625724,-0.952121241183367,-0.927768063492579,-0.897528344122859,
-0.890422007491915,-0.88677445412746,-0.883852594659744,-0.880515003648459,
-0.874696371383313,-0.841004067262,-0.809194504970679,-0.80475635347989,
-0.802644998649867,-0.800998853951234,-0.799050350652882,-0.795391476131473,
-0.790674925746254,-0.779515916321856,-0.758056026301051,-0.728274550313147,
-0.722603026298116,-0.71929668125776,-0.716663283719795,-0.713110911863436,
-0.706251058904969,-0.681414394153353,-0.664173309890699,-0.641010840331872,
-0.637521770485119,-0.635588009058922,-0.633940015803678,-0.631771860119216,
-0.626983925141381,-0.620275487243704,-0.600572143853975,-0.563887321355189,
-0.557592417685907,-0.553819985285405,-0.550877804085015,-0.547650150454212,
-0.542345788290194,-0.52029942361843,-0.490783397563295,-0.481730749060472,
-0.473028532839146,-0.470220605273364,-0.468456040720251,-0.466744374073428,
-0.464183686712158,-0.456819858487764,-0.444595292746979,-0.408196906789883,
-0.393413768926188,-0.388553455325311,-0.385420683702292,-0.382442721578806,
-0.378370326822386,-0.368591201930815,-0.354363130366284,-0.333746464794258,
-0.327283429937007,-0.307663483050674,-0.304218190638545,-0.302294269442552,
-0.300660627497915,-0.298487399945628,-0.293670763739243,-0.286908483169456,
-0.266925607332375,-0.230666924039089,-0.224347649236332,-0.22056846853901,
-0.217625527026843,-0.214401607785031,-0.209113985222482,-0.187344644158807,
-0.167058649673325,-0.143036928693502,-0.138294097017229,-0.136157184391538,
-0.134508828517522,-0.132953913036267,-0.130112873812364,-0.118903817561915,
-0.0944770245339817,-0.0643468468871919,-0.057236613713599,-0.0535885291722072,
-0.0506669537412706,-0.0473304568577627,-0.0415157530421755,-0.0343788544218471,
-0.00049243862796517),.UNSPECIFIED.);
#637=B_SPLINE_CURVE_WITH_KNOTS('',3,(#56712,#56713,#56714,#56715,#56716,
#56717,#56718,#56719,#56720,#56721,#56722,#56723,#56724,#56725,#56726,#56727,
#56728,#56729),.UNSPECIFIED.,.F.,.F.,(4,2,2,2,2,2,2,2,4),(-2.10003863830129,
-2.07623146422239,-2.07278785006591,-2.07065464050834,-2.0690363565175,
-2.0674037107728,-2.06546955883118,-2.06197975505772,-2.04125292518874),
 .UNSPECIFIED.);
#638=B_SPLINE_CURVE_WITH_KNOTS('',3,(#56730,#56731,#56732,#56733,#56734,
#56735,#56736,#56737,#56738,#56739,#56740,#56741,#56742,#56743,#56744,#56745,
#56746,#56747,#56748,#56749,#56750,#56751,#56752,#56753,#56754,#56755,#56756,
#56757,#56758,#56759,#56760,#56761,#56762,#56763,#56764,#56765,#56766,#56767,
#56768,#56769,#56770,#56771,#56772,#56773,#56774,#56775,#56776,#56777,#56778,
#56779,#56780,#56781,#56782,#56783,#56784,#56785,#56786,#56787,#56788,#56789,
#56790,#56791,#56792,#56793,#56794,#56795,#56796,#56797,#56798,#56799,#56800,
#56801,#56802,#56803,#56804,#56805,#56806,#56807,#56808,#56809,#56810,#56811,
#56812,#56813,#56814,#56815,#56816,#56817,#56818,#56819,#56820,#56821,#56822,
#56823,#56824,#56825,#56826,#56827,#56828,#56829,#56830,#56831,#56832,#56833,
#56834,#56835,#56836,#56837,#56838,#56839,#56840,#56841,#56842,#56843,#56844,
#56845,#56846,#56847,#56848,#56849,#56850,#56851,#56852,#56853,#56854,#56855,
#56856,#56857,#56858,#56859,#56860,#56861,#56862,#56863,#56864,#56865,#56866,
#56867,#56868,#56869,#56870,#56871,#56872,#56873,#56874,#56875,#56876,#56877,
#56878,#56879,#56880,#56881,#56882,#56883,#56884,#56885,#56886,#56887,#56888,
#56889,#56890,#56891,#56892,#56893,#56894,#56895,#56896,#56897,#56898,#56899,
#56900,#56901,#56902,#56903,#56904,#56905,#56906,#56907,#56908,#56909,#56910,
#56911,#56912,#56913,#56914,#56915,#56916,#56917,#56918,#56919,#56920,#56921,
#56922,#56923,#56924,#56925,#56926,#56927,#56928,#56929,#56930,#56931),
 .UNSPECIFIED.,.F.,.F.,(4,2,2,2,2,2,2,2,2,2,2,2,2,2,2,2,2,2,2,2,2,2,2,2,
2,2,2,2,2,2,2,2,2,2,2,2,2,2,2,2,2,2,2,2,2,2,2,2,2,2,2,2,2,2,2,2,2,2,2,2,
2,2,2,2,2,2,2,2,2,2,2,2,2,2,2,2,2,2,2,2,2,2,2,2,2,2,2,2,2,2,2,2,2,2,2,2,
2,2,2,2,4),(-1.10892217029559,-1.07977061052498,-1.05716920039812,-1.04992924047292,
-1.04486002851235,-1.04266549991244,-1.04100992873101,-1.03911560203961,
-1.03571400353351,-1.01627636280745,-0.984411849646787,-0.967153296080242,
-0.961999934824887,-0.958804169550778,-0.955851415031561,-0.951942584082718,
-0.943161785897095,-0.930902592489248,-0.909029488294242,-0.882809097489435,
-0.878053163624821,-0.875913518789525,-0.87426444993826,-0.87233549498649,
-0.868770758403794,-0.864210344046972,-0.820568312949517,-0.800799331652675,
-0.795476441022647,-0.792244627651719,-0.789303225026949,-0.785474199084657,
-0.777148459163312,-0.757063927222483,-0.736613062583773,-0.714189528100988,
-0.710702658399633,-0.70876932791681,-0.70713686119596,-0.704977106573372,
-0.700235985337598,-0.678792316347286,-0.63944817301007,-0.630911625566706,
-0.627087149890059,-0.624137522882779,-0.620934841114427,-0.61574710587523,
-0.595536204111023,-0.573963587623792,-0.567249067055552,-0.547481566526644,
-0.544032326559917,-0.542107459018176,-0.540473853577796,-0.538301761381941,
-0.533491848869111,-0.526742255744353,-0.50682574584309,-0.470468009964309,
-0.464154122883258,-0.460376354461172,-0.457433470609105,-0.454208554046077,
-0.448916827016657,-0.427082142033797,-0.396359823121102,-0.380611628413457,
-0.377291981024385,-0.375396229468092,-0.373741538414354,-0.371512267349576,
-0.366377026296749,-0.35900820694939,-0.335647175203267,-0.304104335968121,
-0.297017436280988,-0.293373916451746,-0.290452404761072,-0.287112073825418,
-0.281280395793052,-0.274117027901466,-0.258314683090749,-0.229447591516495,
-0.213959816265293,-0.210656215495483,-0.20876409421353,-0.207108606424764,
-0.204872950091473,-0.199700445513516,-0.19225937055201,-0.16846260644167,
-0.137546108323334,-0.130419868389251,-0.126768253711598,-0.123846104205907,
-0.12051138894092,-0.114927369485567,-0.0925606574938055,-0.0692245969056221,
-0.0592684060220813),.UNSPECIFIED.);
#639=B_SPLINE_CURVE_WITH_KNOTS('',3,(#56936,#56937,#56938,#56939,#56940,
#56941,#56942,#56943,#56944,#56945,#56946,#56947,#56948,#56949,#56950,#56951,
#56952,#56953,#56954,#56955,#56956,#56957,#56958,#56959,#56960,#56961,#56962,
#56963,#56964,#56965,#56966,#56967,#56968,#56969,#56970,#56971,#56972,#56973,
#56974,#56975,#56976,#56977,#56978,#56979,#56980,#56981,#56982,#56983,#56984,
#56985,#56986,#56987,#56988,#56989,#56990,#56991,#56992,#56993,#56994,#56995,
#56996,#56997,#56998,#56999,#57000,#57001,#57002,#57003,#57004,#57005,#57006,
#57007,#57008,#57009,#57010,#57011,#57012,#57013,#57014,#57015,#57016,#57017,
#57018,#57019,#57020,#57021,#57022,#57023,#57024,#57025,#57026,#57027,#57028,
#57029,#57030,#57031,#57032,#57033,#57034,#57035,#57036,#57037,#57038,#57039,
#57040,#57041,#57042,#57043,#57044,#57045,#57046,#57047,#57048,#57049,#57050,
#57051,#57052,#57053,#57054,#57055,#57056,#57057,#57058,#57059,#57060,#57061,
#57062,#57063,#57064,#57065,#57066,#57067,#57068,#57069,#57070,#57071,#57072,
#57073,#57074,#57075,#57076,#57077,#57078,#57079,#57080,#57081,#57082,#57083,
#57084,#57085,#57086,#57087,#57088,#57089,#57090,#57091,#57092,#57093,#57094,
#57095,#57096,#57097,#57098,#57099,#57100,#57101,#57102,#57103,#57104,#57105,
#57106,#57107,#57108,#57109,#57110,#57111,#57112,#57113,#57114,#57115,#57116,
#57117,#57118,#57119,#57120,#57121,#57122,#57123,#57124,#57125,#57126,#57127,
#57128,#57129,#57130,#57131,#57132,#57133,#57134,#57135,#57136,#57137,#57138,
#57139,#57140,#57141,#57142,#57143,#57144,#57145,#57146,#57147,#57148,#57149,
#57150,#57151,#57152,#57153,#57154,#57155),.UNSPECIFIED.,.F.,.F.,(4,2,2,
2,2,2,2,2,2,2,2,2,2,2,2,2,2,2,2,2,2,2,2,2,2,2,2,2,2,2,2,2,2,2,2,2,2,2,2,
2,2,2,2,2,2,2,2,2,2,2,2,2,2,2,2,2,2,2,2,2,2,2,2,2,2,2,2,2,2,2,2,2,2,2,2,
2,2,2,2,2,2,2,2,2,2,2,2,2,2,2,2,2,2,2,2,2,2,2,2,2,2,2,2,2,2,2,2,2,2,4),
(-2.04107968292539,-2.03912981917729,-2.0048225815275,-1.98351435642058,
-1.97650461157569,-1.97166709581427,-1.96954725840733,-1.9695285662276,
-1.96950978091368,-1.96949089720669,-1.9694719097205,-1.96945281294638,
-1.96943360124378,-1.96941426883361,-1.96939480978555,-1.96937521801775,
-1.96935548728387,-1.96933561116716,-1.96931558306975,-1.96768229331185,
-1.96575619541819,-1.9623010616684,-1.94230173381455,-1.9363019019545,-1.91613618146969,
-1.89421833913387,-1.88892149847947,-1.88569557019274,-1.88275313205163,
-1.87897783864951,-1.87267247716432,-1.83620825638503,-1.81638736440693,
-1.80965665605659,-1.80485646689005,-1.80268618791043,-1.80105282377578,
-1.79912693680099,-1.79567286095932,-1.77571946601929,-1.76913999928947,
-1.74748708344607,-1.72736324038356,-1.72218144260936,-1.71898014772262,
-1.71603030302744,-1.71220343282242,-1.70365209525522,-1.66434714192865,
-1.64292097543161,-1.63818169056154,-1.63602236387148,-1.63439002904643,
-1.63245666470425,-1.62896924848144,-1.6064982183182,-1.58606343303989,
-1.56597522035059,-1.55764800827625,-1.55381889592321,-1.55087769236065,
-1.54764636768968,-1.54232490151658,-1.52256891253161,-1.47895025392957,
-1.47439047428474,-1.47082595849344,-1.46889720594573,-1.46724838536718,
-1.46510913243169,-1.46035444640193,-1.43408802627636,-1.39878650370007,
-1.39078641298447,-1.38701616642852,-1.38408211823684,-1.38081999444658,
-1.37535530481451,-1.35304886052624,-1.3198322720283,-1.31111597266874,
-1.30530757804627,-1.30296768369608,-1.30129696484661,-1.2994563381938,
-1.29630154351432,-1.28399906419146,-1.25639063979944,-1.22812636576549,
-1.22254554291355,-1.21925860776149,-1.21632945573473,-1.21260294499472,
-1.20660840436975,-1.16655994392253,-1.14140035187514,-1.13762737104125,
-1.13565516393516,-1.134011272871,-1.13189571311841,-1.12739418954014,-1.09573079631599,
-1.0624488105668,-1.05630214962849,-1.05289547679305,-1.05027172928781,
-1.04684103859437,-1.0405789325978,-1.00799398371958,-0.991342359623623),
 .UNSPECIFIED.);
#640=B_SPLINE_CURVE_WITH_KNOTS('',3,(#57157,#57158,#57159,#57160,#57161,
#57162,#57163,#57164,#57165,#57166,#57167,#57168,#57169,#57170,#57171,#57172,
#57173,#57174),.UNSPECIFIED.,.F.,.F.,(4,2,2,2,2,2,2,2,4),(-0.0592684060220813,
-0.0476535235343102,-0.0441711697069289,-0.0422389384242401,-0.0406064702951486,
-0.0384455037053382,-0.0360426986767971,-0.0291414406123908,-0.000492293290300633),
 .UNSPECIFIED.);
#641=B_SPLINE_CURVE_WITH_KNOTS('',3,(#57175,#57176,#57177,#57178,#57179,
#57180,#57181,#57182,#57183,#57184,#57185,#57186,#57187,#57188,#57189,#57190,
#57191,#57192,#57193,#57194,#57195,#57196,#57197,#57198,#57199,#57200,#57201,
#57202,#57203,#57204,#57205,#57206,#57207,#57208,#57209,#57210,#57211,#57212,
#57213,#57214,#57215,#57216,#57217,#57218,#57219,#57220,#57221,#57222,#57223,
#57224,#57225,#57226,#57227,#57228,#57229,#57230,#57231,#57232,#57233,#57234,
#57235,#57236,#57237,#57238,#57239,#57240,#57241,#57242,#57243,#57244,#57245,
#57246,#57247,#57248,#57249,#57250,#57251,#57252,#57253,#57254,#57255,#57256,
#57257,#57258,#57259,#57260,#57261,#57262,#57263,#57264,#57265,#57266,#57267,
#57268,#57269,#57270,#57271,#57272,#57273,#57274,#57275,#57276,#57277,#57278,
#57279,#57280,#57281,#57282,#57283,#57284,#57285,#57286,#57287,#57288,#57289,
#57290,#57291,#57292,#57293,#57294,#57295,#57296,#57297,#57298,#57299,#57300,
#57301,#57302,#57303,#57304,#57305,#57306,#57307,#57308,#57309,#57310,#57311,
#57312,#57313,#57314,#57315,#57316,#57317,#57318,#57319,#57320,#57321,#57322,
#57323,#57324,#57325,#57326,#57327,#57328,#57329,#57330,#57331,#57332,#57333,
#57334,#57335,#57336,#57337,#57338,#57339,#57340,#57341,#57342,#57343,#57344,
#57345,#57346,#57347,#57348,#57349,#57350,#57351,#57352,#57353,#57354,#57355,
#57356,#57357,#57358,#57359,#57360,#57361,#57362,#57363,#57364,#57365,#57366),
 .UNSPECIFIED.,.F.,.F.,(4,2,2,2,2,2,2,2,2,2,2,2,2,2,2,2,2,2,2,2,2,2,2,2,
2,2,2,2,2,2,2,2,2,2,2,2,2,2,2,2,2,2,2,2,2,2,2,2,2,2,2,2,2,2,2,2,2,2,2,2,
2,2,2,2,2,2,2,2,2,2,2,2,2,2,2,2,2,2,2,2,2,2,2,2,2,2,2,2,2,2,2,2,2,2,2,4),
(-2.10024321870136,-2.07707792275481,-2.06711782544992,-2.06329783132158,
-2.05972750725702,-2.05709217806112,-2.05379808839827,-2.04818456503473,
-2.02230314793019,-1.99230694904503,-1.98355151667432,-1.97831015024971,
-1.97601402809443,-1.97435004430234,-1.97248918633476,-1.96924172354253,
-1.95559655504945,-1.92250708278932,-1.90068718550792,-1.89539582732966,
-1.89217086591551,-1.88922777510974,-1.88544951258308,-1.87913433710995,
-1.84270016161805,-1.81418127696254,-1.81060830863966,-1.80867775764828,
-1.80702917180144,-1.80489244488389,-1.80015197634527,-1.77433796645994,
-1.75215349924101,-1.73980992255565,-1.73098599752092,-1.7270701043728,
-1.72411665625155,-1.72092460280781,-1.71578717108399,-1.69869766620876,
-1.66678662080639,-1.64883354501731,-1.64446379018397,-1.64237311605805,
-1.64088880077462,-1.63896648074959,-1.6355290666056,-1.61622713407328,
-1.60917179549341,-1.59223406547781,-1.56767410822126,-1.56223672969039,
-1.55898031957867,-1.55604479404011,-1.55226336367259,-1.54608017128318,
-1.50066732507311,-1.48223264758986,-1.47780833117923,-1.47570717308704,
-1.47422164579736,-1.47230651246261,-1.46890164978239,-1.4510590234456,
-1.40576998535077,-1.3974001136669,-1.39356326812386,-1.39062088277286,
-1.38739298356253,-1.38208815819019,-1.3623654816402,-1.31870481884646,
-1.31413282570107,-1.31056085255604,-1.30863044521136,-1.30698172807918,
-1.30484451165599,-1.30010172423279,-1.27420809119123,-1.25207771052209,
-1.23974817930593,-1.23093148578801,-1.22701669035783,-1.22406326691605,
-1.22087046843874,-1.21573011602368,-1.1986107891338,-1.16671382283516,
-1.14877524470587,-1.1444070115815,-1.14231655680953,-1.14083219336127,
-1.13890952443559,-1.1354708287498,-1.11612762531855,-1.10923588654368),
 .UNSPECIFIED.);
#642=B_SPLINE_CURVE_WITH_KNOTS('',3,(#57372,#57373,#57374,#57375,#57376,
#57377,#57378,#57379,#57380,#57381,#57382,#57383,#57384,#57385,#57386,#57387,
#57388,#57389,#57390,#57391,#57392,#57393,#57394,#57395,#57396,#57397,#57398,
#57399,#57400,#57401,#57402,#57403,#57404,#57405,#57406,#57407,#57408,#57409,
#57410,#57411,#57412,#57413,#57414,#57415,#57416,#57417,#57418,#57419,#57420,
#57421,#57422,#57423,#57424,#57425,#57426,#57427,#57428,#57429,#57430,#57431,
#57432,#57433,#57434,#57435,#57436,#57437,#57438,#57439,#57440,#57441,#57442,
#57443,#57444,#57445,#57446,#57447,#57448,#57449,#57450,#57451,#57452,#57453,
#57454,#57455,#57456,#57457,#57458,#57459,#57460,#57461,#57462,#57463,#57464,
#57465,#57466,#57467,#57468,#57469,#57470,#57471,#57472,#57473,#57474,#57475,
#57476,#57477,#57478,#57479,#57480,#57481,#57482,#57483,#57484,#57485,#57486,
#57487,#57488,#57489,#57490,#57491,#57492,#57493,#57494,#57495,#57496,#57497,
#57498,#57499,#57500,#57501,#57502,#57503,#57504,#57505,#57506,#57507,#57508,
#57509,#57510,#57511,#57512,#57513,#57514,#57515,#57516,#57517,#57518,#57519,
#57520,#57521,#57522,#57523,#57524,#57525,#57526,#57527,#57528,#57529,#57530,
#57531,#57532,#57533,#57534,#57535,#57536,#57537,#57538,#57539,#57540,#57541,
#57542,#57543,#57544,#57545,#57546,#57547,#57548,#57549,#57550,#57551,#57552,
#57553,#57554,#57555,#57556,#57557,#57558,#57559,#57560,#57561),
 .UNSPECIFIED.,.F.,.F.,(4,2,2,2,2,2,2,2,2,2,2,2,2,2,2,2,2,2,2,2,2,2,2,2,
2,2,2,2,2,2,2,2,2,2,2,2,2,2,2,2,2,2,2,2,2,2,2,2,2,2,2,2,2,2,2,2,2,2,2,2,
2,2,2,2,2,2,2,2,2,2,2,2,2,2,2,2,2,2,2,2,2,2,2,2,2,2,2,2,2,2,2,2,2,2,4),
(-0.991267371540882,-0.981097406136092,-0.961289637880318,-0.955963818240538,
-0.952730934488633,-0.949789014332813,-0.945959973544135,-0.937636954346978,
-0.917741432724483,-0.899079532049941,-0.874679746066063,-0.871177710298744,
-0.869240758346818,-0.86759270846697,-0.865427943897829,-0.860660623001553,
-0.838957771522791,-0.79880290397272,-0.790989179326245,-0.787252812944483,
-0.784322095269493,-0.781039835244787,-0.775482867469908,-0.747961936710415,
-0.721701316292262,-0.707512672722365,-0.704234828931467,-0.702367217000256,
-0.700704961506073,-0.698421757030807,-0.692967771532784,-0.68497266253003,
-0.657551018852252,-0.628614552485425,-0.622983204284046,-0.619653476414371,
-0.616757809401868,-0.613110873353384,-0.605770555596228,-0.596121644487729,
-0.570173960882816,-0.543192066135581,-0.538460341580936,-0.536325031335904,
-0.534676403898006,-0.532744477392873,-0.529165651271156,-0.524582011701536,
-0.480864614772306,-0.461176484442266,-0.455872907032115,-0.452645234750042,
-0.449702725036517,-0.445865241338196,-0.437491895333081,-0.415543915585245,
-0.376154006902127,-0.371637296527056,-0.369518833154948,-0.367874677932461,
-0.365904570733226,-0.362142035717488,-0.335352594349984,-0.297235673647581,
-0.291046981012426,-0.287264091086249,-0.284328531102157,-0.281073205365896,
-0.275640321869276,-0.251163953398819,-0.235940471739304,-0.209866033016854,
-0.205097771000572,-0.202956161961828,-0.201307155286976,-0.199380178941985,
-0.195823792956285,-0.167698745841791,-0.130677556443954,-0.124434073669649,
-0.120676282483605,-0.117736173207668,-0.114501241627693,-0.110357857457294,
-0.0954997269774895,-0.0680120021072093,-0.0665756166986164,-0.0431806880535247,
-0.0384358331732864,-0.0362985123773095,-0.0346500636920598,-0.0327204332147608,
-0.0306502677252412,-0.027362718736346,-0.000492130215965281),
 .UNSPECIFIED.);
#643=B_SPLINE_CURVE_WITH_KNOTS('',3,(#57562,#57563,#57564,#57565,#57566,
#57567,#57568,#57569,#57570,#57571,#57572,#57573,#57574,#57575,#57576,#57577),
 .UNSPECIFIED.,.F.,.F.,(4,2,2,2,2,2,2,4),(-2.10016741640826,-2.06493740655749,
-2.05955177493146,-2.05604419942285,-2.05269364711443,-2.04977344098074,
-2.04614491118763,-2.04107968292539),.UNSPECIFIED.);
#644=B_SPLINE_CURVE_WITH_KNOTS('',3,(#57578,#57579,#57580,#57581,#57582,
#57583,#57584,#57585,#57586,#57587,#57588,#57589,#57590,#57591,#57592,#57593,
#57594,#57595,#57596,#57597,#57598,#57599,#57600,#57601,#57602,#57603,#57604,
#57605,#57606,#57607,#57608,#57609,#57610,#57611,#57612,#57613,#57614,#57615,
#57616,#57617,#57618,#57619,#57620,#57621,#57622,#57623,#57624,#57625,#57626,
#57627,#57628,#57629,#57630,#57631,#57632,#57633,#57634,#57635,#57636,#57637,
#57638,#57639,#57640,#57641,#57642,#57643,#57644,#57645,#57646,#57647,#57648,
#57649,#57650,#57651,#57652,#57653,#57654,#57655,#57656,#57657,#57658,#57659,
#57660,#57661,#57662,#57663,#57664,#57665,#57666,#57667,#57668,#57669,#57670,
#57671,#57672,#57673,#57674,#57675,#57676,#57677,#57678,#57679,#57680,#57681,
#57682,#57683,#57684,#57685,#57686,#57687,#57688,#57689,#57690,#57691,#57692,
#57693,#57694,#57695,#57696,#57697,#57698,#57699,#57700,#57701,#57702,#57703,
#57704,#57705,#57706,#57707,#57708,#57709,#57710,#57711,#57712,#57713,#57714,
#57715,#57716,#57717,#57718,#57719,#57720,#57721,#57722,#57723,#57724,#57725,
#57726,#57727,#57728,#57729,#57730,#57731,#57732,#57733,#57734,#57735,#57736,
#57737,#57738,#57739,#57740,#57741,#57742,#57743,#57744,#57745,#57746,#57747,
#57748,#57749,#57750,#57751,#57752,#57753,#57754,#57755,#57756,#57757,#57758,
#57759,#57760,#57761,#57762,#57763,#57764,#57765,#57766,#57767,#57768,#57769,
#57770,#57771,#57772,#57773,#57774,#57775,#57776,#57777,#57778,#57779,#57780,
#57781,#57782,#57783,#57784,#57785,#57786,#57787,#57788,#57789,#57790,#57791),
 .UNSPECIFIED.,.F.,.F.,(4,2,2,2,2,2,2,2,2,2,2,2,2,2,2,2,2,2,2,2,2,2,2,2,
2,2,2,2,2,2,2,2,2,2,2,2,2,2,2,2,2,2,2,2,2,2,2,2,2,2,2,2,2,2,2,2,2,2,2,2,
2,2,2,2,2,2,2,2,2,2,2,2,2,2,2,2,2,2,2,2,2,2,2,2,2,2,2,2,2,2,2,2,2,2,2,2,
2,2,2,2,2,2,2,2,2,2,4),(-1.10923588654368,-1.10907489650741,-1.08811016372412,
-1.0742351092368,-1.064630297109,-1.06058510884969,-1.05761126720607,-1.05484576592113,
-1.05027687983568,-1.0368672406629,-1.0139618145347,-0.982338813730652,
-0.977836583040976,-0.975720782895241,-0.974076736880993,-0.97210439253702,
-0.968331230092938,-0.943182445645729,-0.903080754354083,-0.897088202095896,
-0.893362148587139,-0.890432858589156,-0.887145247687724,-0.881561944909125,
-0.853209100684674,-0.825443254516931,-0.813394637755911,-0.810258547377462,
-0.80842192441521,-0.806749511416559,-0.804399805379745,-0.798529409980879,
-0.789683242550104,-0.755268601597045,-0.734188241135488,-0.728801347940153,
-0.725555796140642,-0.722617826945827,-0.718815949577427,-0.710641946634318,
-0.68706843989935,-0.660144754735399,-0.646899933302174,-0.643683003100304,
-0.641828772518293,-0.640162724308558,-0.63785269387803,-0.632232526221822,
-0.623901805757191,-0.597859235588111,-0.568080476315045,-0.562408813783103,
-0.559102368203098,-0.55646887779565,-0.552916361888428,-0.546056153431242,
-0.521217451267762,-0.503977855429484,-0.480816552076902,-0.477327416086255,
-0.475393603404864,-0.473745555206681,-0.471577308491671,-0.466789096983762,
-0.460080209879909,-0.440374969823515,-0.403691347393369,-0.397396071909866,
-0.393623437094854,-0.390681107057097,-0.387453296630241,-0.38214868304125,
-0.360100628016921,-0.330638238472297,-0.322750972856152,-0.313051057321137,
-0.310133127459941,-0.308344368223593,-0.306648647781612,-0.304169277322039,
-0.297416795480203,-0.253609349296573,-0.234068468048544,-0.228773062820673,
-0.225547285533778,-0.222604507906213,-0.218763783217159,-0.210371186849552,
-0.187685857503641,-0.161867181656076,-0.147127221360853,-0.14385974154063,
-0.141975822633647,-0.140318648031415,-0.140299661724828,-0.140280785134233,
-0.140262012701252,-0.14024333899365,-0.140224758702261,-0.138112029931578,
-0.133231174375814,-0.12618494866544,-0.10467721515721,-0.0706109688986338,
-0.0635859596188316,-0.0599556336597502,-0.059542488620295),
 .UNSPECIFIED.);
#645=B_SPLINE_CURVE_WITH_KNOTS('',3,(#57797,#57798,#57799,#57800,#57801,
#57802,#57803,#57804,#57805,#57806),.UNSPECIFIED.,.F.,.F.,(4,3,3,4),(-4.19977379117109,
-4.09016305838479,-3.9901141377464,-3.84638326369218),.UNSPECIFIED.);
#646=B_SPLINE_CURVE_WITH_KNOTS('',3,(#57808,#57809,#57810,#57811,#57812,
#57813,#57814,#57815,#57816,#57817,#57818,#57819,#57820,#57821,#57822,#57823,
#57824,#57825,#57826,#57827,#57828,#57829,#57830,#57831,#57832,#57833,#57834,
#57835,#57836,#57837,#57838,#57839,#57840,#57841,#57842,#57843,#57844,#57845,
#57846,#57847,#57848,#57849,#57850,#57851,#57852,#57853,#57854,#57855,#57856,
#57857,#57858,#57859,#57860,#57861,#57862,#57863,#57864,#57865,#57866,#57867,
#57868,#57869,#57870,#57871,#57872,#57873,#57874,#57875,#57876,#57877,#57878,
#57879,#57880,#57881,#57882,#57883,#57884,#57885,#57886,#57887,#57888,#57889,
#57890,#57891,#57892,#57893,#57894,#57895,#57896,#57897,#57898,#57899,#57900,
#57901,#57902,#57903,#57904,#57905,#57906,#57907,#57908,#57909,#57910,#57911,
#57912,#57913,#57914,#57915,#57916),.UNSPECIFIED.,.F.,.F.,(4,3,3,3,3,3,
3,3,3,3,3,3,3,3,3,3,3,3,3,3,3,3,3,3,3,3,3,3,3,3,3,3,3,3,3,3,4),(-3.84638326322552,
-3.73817105610137,-3.63007941822935,-3.52206551072006,-3.41408661602619,
-3.30602494476234,-3.19792576134903,-3.08962895712806,-2.9925856033098,
-2.88263947138076,-2.77169167106731,-2.66204168456622,-2.55245679950798,
-2.44289661082298,-2.33093672533553,-2.22123487990582,-2.10814597438951,
-1.9950570688732,-1.88644978490181,-1.77533462859366,-1.66702721094067,
-1.55878298609703,-1.45055963187852,-1.33730185751804,-1.22891272071361,
-1.12043521194772,-1.0117545264651,-0.997528534436599,-0.884663102669983,
-0.77203800889968,-0.659554849770297,-0.547180407463164,-0.434881614271142,
-0.322591337129412,-0.210315510204404,-0.0979547765619886,0.),
 .UNSPECIFIED.);
#647=B_SPLINE_CURVE_WITH_KNOTS('',3,(#57920,#57921,#57922,#57923,#57924,
#57925,#57926,#57927,#57928,#57929,#57930,#57931,#57932,#57933,#57934,#57935,
#57936,#57937,#57938,#57939,#57940,#57941,#57942,#57943,#57944,#57945,#57946,
#57947,#57948,#57949,#57950,#57951,#57952,#57953,#57954,#57955,#57956,#57957,
#57958,#57959,#57960,#57961,#57962,#57963,#57964,#57965,#57966,#57967,#57968,
#57969,#57970,#57971,#57972,#57973,#57974,#57975,#57976,#57977,#57978,#57979,
#57980,#57981,#57982,#57983,#57984,#57985,#57986,#57987,#57988,#57989,#57990,
#57991,#57992,#57993,#57994,#57995,#57996,#57997,#57998,#57999,#58000,#58001,
#58002,#58003,#58004,#58005,#58006,#58007,#58008,#58009,#58010,#58011,#58012,
#58013,#58014,#58015,#58016,#58017,#58018,#58019,#58020,#58021,#58022,#58023,
#58024,#58025,#58026,#58027,#58028,#58029,#58030,#58031,#58032,#58033,#58034,
#58035,#58036,#58037,#58038,#58039,#58040,#58041,#58042,#58043,#58044,#58045,
#58046,#58047,#58048,#58049,#58050,#58051,#58052,#58053,#58054,#58055,#58056,
#58057,#58058,#58059,#58060,#58061,#58062,#58063,#58064,#58065,#58066,#58067,
#58068,#58069,#58070,#58071,#58072,#58073),.UNSPECIFIED.,.F.,.F.,(4,3,3,
3,3,3,3,3,3,3,3,3,3,3,3,3,3,3,3,3,3,3,3,3,3,3,3,3,3,3,3,3,3,3,3,3,3,3,3,
3,3,3,3,3,3,3,3,3,3,3,3,4),(2.01461790129682,2.12418716397154,2.23356422085981,
2.34283392492382,2.4520374248202,2.56121577723765,2.67048870477471,2.77980488942863,
2.889327464259,2.9925856033098,3.10257102449589,3.2135139136522,3.3232066348227,
3.43283544876539,3.54244070750851,3.65435906506798,3.76410838117625,3.87711125946132,
3.9901141377464,4.09976168164098,4.21074680545873,4.32008694433128,4.42935866471988,
4.53860290679355,4.65086284814091,4.76024559746015,4.87394413482158,4.987642672183,
5.09746924953473,5.20843199417034,5.31795635452642,5.42741372572691,5.53684474715618,
5.64892636202204,5.75849655049291,5.87183387855625,5.9851712066196,6.09498856633222,
6.20595246317272,6.31546860664133,6.42491816034262,6.53434177815616,6.64643126888117,
6.75599517379492,6.86934745742556,6.98269974105619,7.09372976479652,7.20457605112106,
7.31525682042945,7.42584067486135,7.5363740838632,7.59300756235147),
 .UNSPECIFIED.);
#648=B_SPLINE_CURVE_WITH_KNOTS('',3,(#58074,#58075,#58076,#58077,#58078,
#58079,#58080,#58081,#58082,#58083),.UNSPECIFIED.,.F.,.F.,(4,2,2,2,4),(-2.10021521608555,
-2.08977397566189,-2.04619577452829,-2.04163297633637,-2.04133728664231),
 .UNSPECIFIED.);
#649=B_SPLINE_CURVE_WITH_KNOTS('',3,(#58085,#58086,#58087,#58088,#58089,
#58090,#58091,#58092,#58093,#58094,#58095,#58096,#58097,#58098,#58099,#58100,
#58101,#58102,#58103,#58104,#58105,#58106,#58107,#58108,#58109,#58110,#58111,
#58112,#58113,#58114,#58115,#58116,#58117,#58118,#58119,#58120,#58121,#58122,
#58123,#58124,#58125,#58126,#58127,#58128,#58129,#58130,#58131,#58132,#58133,
#58134,#58135,#58136,#58137,#58138,#58139,#58140,#58141,#58142,#58143,#58144,
#58145,#58146,#58147,#58148,#58149,#58150,#58151,#58152,#58153,#58154,#58155,
#58156,#58157,#58158,#58159,#58160,#58161,#58162,#58163,#58164,#58165,#58166,
#58167,#58168,#58169,#58170,#58171,#58172,#58173,#58174,#58175,#58176,#58177,
#58178,#58179,#58180,#58181,#58182,#58183,#58184,#58185,#58186,#58187,#58188,
#58189,#58190,#58191,#58192,#58193,#58194,#58195,#58196,#58197,#58198,#58199,
#58200,#58201,#58202,#58203,#58204,#58205,#58206,#58207,#58208,#58209,#58210,
#58211,#58212,#58213,#58214,#58215,#58216,#58217,#58218,#58219,#58220,#58221,
#58222,#58223,#58224,#58225,#58226,#58227,#58228,#58229,#58230,#58231,#58232,
#58233,#58234,#58235,#58236,#58237,#58238,#58239,#58240,#58241,#58242,#58243,
#58244,#58245,#58246,#58247,#58248,#58249,#58250,#58251,#58252,#58253,#58254,
#58255,#58256,#58257,#58258,#58259,#58260,#58261,#58262,#58263,#58264,#58265,
#58266,#58267,#58268,#58269,#58270,#58271,#58272,#58273,#58274,#58275,#58276,
#58277,#58278,#58279,#58280,#58281,#58282,#58283,#58284,#58285,#58286,#58287,
#58288,#58289,#58290),.UNSPECIFIED.,.F.,.F.,(4,2,2,2,2,2,2,2,2,2,2,2,2,
2,2,2,2,2,2,2,2,2,2,2,2,2,2,2,2,2,2,2,2,2,2,2,2,2,2,2,2,2,2,2,2,2,2,2,2,
2,2,2,2,2,2,2,2,2,2,2,2,2,2,2,2,2,2,2,2,2,2,2,2,2,2,2,2,2,2,2,2,2,2,2,2,
2,2,2,2,2,2,2,2,2,2,2,2,2,2,2,2,2,4),(-2.04133728664231,-2.03806711232071,
-2.03613907650113,-2.03449055238448,-2.03235217524117,-2.02760496330045,
-2.00202283253427,-1.97591246252407,-1.96559219509398,-1.96019425817351,
-1.95593710094107,-1.95287443123683,-1.94992358151013,-1.94610252245451,
-1.93759501511552,-1.89825821024276,-1.87681852679445,-1.87207606932991,
-1.8699148703817,-1.8682811787169,-1.86634641277876,-1.8628553805761,-1.83968413016769,
-1.82243749714789,-1.79756842834387,-1.79070352001133,-1.78714940531321,
-1.78451508752835,-1.78120805003946,-1.77553653065459,-1.74564750693976,
-1.72396566567071,-1.71301873243646,-1.70619061438184,-1.70370068664817,
-1.70200282576786,-1.70043652798863,-1.69774825086984,-1.69001707168038,
-1.68012220978552,-1.64983524325786,-1.62808615729811,-1.62279842835429,
-1.61957399019187,-1.61663030034402,-1.61284979232203,-1.60456738736788,
-1.56495150346657,-1.54342226860357,-1.53867210557083,-1.53651054213067,
-1.53487761097175,-1.53294478498958,-1.52946168918287,-1.50799234015133,
-1.48675521374221,-1.46170057201891,-1.45623931075393,-1.45297715685123,
-1.4500417908405,-1.44626803601958,-1.43825317764822,-1.39834539656004,
-1.37672504194426,-1.37196540548511,-1.36980178070214,-1.36816840109125,
-1.36623647588984,-1.36275755849242,-1.34162583446689,-1.33696943245491,
-1.316926136774,-1.30217031603712,-1.29213517037851,-1.28802172545601,-1.28503580743141,
-1.2819143899054,-1.27711198179445,-1.26288326346744,-1.22919925276079,
-1.20970439702231,-1.20516353826991,-1.20304024190205,-1.20155196837831,
-1.19965130151577,-1.19631170686557,-1.18038607711524,-1.14977864296839,
-1.12796756740681,-1.12267550373085,-1.11944977035899,-1.1165057593254,
-1.11272602219167,-1.10640773541409,-1.07010882937329,-1.05015950680568,
-1.04028702126582,-1.03735074321361,-1.03555761652194,-1.03386376621982,
-1.03139575260707,-1.02472742835449,-0.991267371540882),.UNSPECIFIED.);
#650=B_SPLINE_CURVE_WITH_KNOTS('',3,(#58292,#58293,#58294,#58295,#58296,
#58297,#58298,#58299,#58300,#58301,#58302,#58303),.UNSPECIFIED.,.F.,.F.,
(4,2,2,2,2,4),(-0.059542488620295,-0.0570356295461016,-0.0536871209915682,
-0.0478149555195779,-0.0135375548234137,-0.000495262918588897),
 .UNSPECIFIED.);
#651=B_SPLINE_CURVE_WITH_KNOTS('',3,(#58304,#58305,#58306,#58307,#58308,
#58309,#58310,#58311,#58312,#58313,#58314,#58315,#58316,#58317,#58318,#58319,
#58320,#58321,#58322,#58323,#58324,#58325,#58326,#58327,#58328,#58329,#58330,
#58331,#58332,#58333,#58334,#58335,#58336,#58337,#58338,#58339,#58340,#58341,
#58342,#58343,#58344,#58345,#58346,#58347,#58348,#58349,#58350,#58351,#58352,
#58353,#58354,#58355,#58356,#58357,#58358,#58359,#58360,#58361,#58362,#58363,
#58364,#58365,#58366,#58367,#58368,#58369,#58370,#58371,#58372,#58373,#58374,
#58375,#58376,#58377,#58378,#58379,#58380,#58381,#58382,#58383,#58384,#58385,
#58386,#58387,#58388,#58389,#58390,#58391,#58392,#58393,#58394,#58395,#58396,
#58397,#58398,#58399,#58400,#58401,#58402,#58403,#58404,#58405,#58406,#58407,
#58408,#58409,#58410,#58411,#58412,#58413,#58414,#58415,#58416,#58417,#58418,
#58419,#58420,#58421,#58422,#58423,#58424,#58425,#58426,#58427,#58428,#58429,
#58430,#58431,#58432,#58433,#58434,#58435,#58436,#58437,#58438,#58439,#58440,
#58441,#58442,#58443,#58444,#58445,#58446,#58447,#58448,#58449,#58450,#58451,
#58452,#58453,#58454,#58455,#58456,#58457,#58458,#58459,#58460,#58461,#58462,
#58463,#58464,#58465,#58466),.UNSPECIFIED.,.F.,.F.,(4,3,3,3,3,3,3,3,3,3,
3,3,3,3,3,3,3,3,3,3,3,3,3,3,3,3,3,3,3,3,3,3,3,3,3,3,3,3,3,3,3,3,3,3,3,3,
3,3,3,3,3,3,3,3,4),(-10.1295685708718,-9.97528534436599,-9.86548762739471,
-9.75452127521155,-9.64502607996208,-9.53559790410113,-9.42619605868901,
-9.31408624649911,-9.20454484153936,-9.09115082573437,-8.97775680992939,
-8.86795596066623,-8.75699000001955,-8.64749148931064,-8.53805993940168,
-8.42865466738962,-8.31654806941542,-8.2070031494851,-8.09361571248895,
-7.9802282754928,-7.87045607245003,-7.7594865310258,-7.65001679670524,-7.54061399239432,
-7.43123738880844,-7.31910297687038,-7.20958620654151,-7.09614297379885,
-6.9826997410562,-6.87287957692727,-6.76191603063881,-6.65239873427587,
-6.54294864619697,-6.43352511152299,-6.32143663529715,-6.21187433502042,
-6.09852277082001,-5.9851712066196,-5.87534579900835,-5.76438290815518,
-5.65485906417595,-5.54540196447979,-5.43597096998016,-5.32388889553087,
-5.21431813074235,-5.10098040146268,-4.987642672183,-4.87803538336313,-4.76858440184659,
-4.65924852673594,-4.54437984284473,-4.43511949060869,-4.32585491445155,
-4.21650483607428,-4.19977379117109),.UNSPECIFIED.);
#652=B_SPLINE_CURVE_WITH_KNOTS('',3,(#58469,#58470,#58471,#58472,#58473,
#58474,#58475,#58476),.UNSPECIFIED.,.F.,.F.,(4,1,1,1,1,4),(17.9345079337947,
18.8442797453129,19.8418082797495,20.8393368141861,21.8368653486227,21.9911485751285),
 .UNSPECIFIED.);
#653=B_SPLINE_CURVE_WITH_KNOTS('',3,(#58477,#58478,#58479,#58480,#58481,
#58482),.UNSPECIFIED.,.F.,.F.,(4,1,1,4),(21.9911485751285,22.8343938830593,
23.8319224174959,24.2177548267501),.UNSPECIFIED.);
#654=B_SPLINE_CURVE_WITH_KNOTS('',3,(#58484,#58485,#58486,#58487,#58488,
#58489),.UNSPECIFIED.,.F.,.F.,(4,1,1,4),(21.9911485751285,22.3783692882697,
23.3758978227063,24.2163931842857),.UNSPECIFIED.);
#655=B_SPLINE_CURVE_WITH_KNOTS('',3,(#58490,#58491,#58492,#58493,#58494,
#58495,#58496,#58497),.UNSPECIFIED.,.F.,.F.,(4,1,1,1,1,4),(17.9337012577548,
18.3882551505233,19.3857836849599,20.3833122193965,21.3808407538331,21.9911485751285),
 .UNSPECIFIED.);
#656=B_SPLINE_CURVE_WITH_KNOTS('',3,(#58499,#58500,#58501,#58502,#58503,
#58504,#58505,#58506,#58507,#58508,#58509,#58510,#58511,#58512,#58513,#58514,
#58515,#58516,#58517,#58518,#58519,#58520,#58521,#58522,#58523,#58524,#58525,
#58526,#58527,#58528,#58529,#58530,#58531,#58532,#58533,#58534,#58535,#58536,
#58537,#58538,#58539,#58540,#58541,#58542,#58543,#58544,#58545,#58546,#58547,
#58548,#58549,#58550,#58551,#58552,#58553,#58554,#58555,#58556,#58557,#58558,
#58559,#58560,#58561,#58562,#58563,#58564,#58565,#58566,#58567,#58568,#58569,
#58570,#58571,#58572,#58573,#58574,#58575,#58576,#58577,#58578,#58579,#58580,
#58581,#58582,#58583,#58584,#58585,#58586),.UNSPECIFIED.,.F.,.F.,(4,3,3,
3,3,3,3,3,3,3,3,3,3,3,3,3,3,3,3,3,3,3,3,3,3,3,3,3,3,4),(-0.378621596831436,
-0.359663577262707,-0.347848706298584,-0.340612126761629,-0.335326919244971,
-0.315444091624407,-0.301124382400315,-0.297137489673917,-0.293208696506955,
-0.272699616571317,-0.251996264868775,-0.231506732846842,-0.228782241774587,
-0.224183786203168,-0.203193217736025,-0.200837552551342,-0.180373385774626,
-0.159349797507194,-0.154347721681245,-0.15081253799708,-0.12949386489982,
-0.107562916419308,-0.085631967938795,-0.0802146534577825,-0.0759481457753231,
-0.0534010597619021,-0.0308288102439276,-0.00877074246183405,-0.00403427920390156,
-4.65348914561155E-5),.UNSPECIFIED.);
#657=B_SPLINE_CURVE_WITH_KNOTS('',3,(#58587,#58588,#58589,#58590,#58591,
#58592,#58593,#58594,#58595,#58596,#58597,#58598,#58599,#58600,#58601,#58602,
#58603,#58604,#58605,#58606,#58607,#58608,#58609,#58610,#58611,#58612,#58613,
#58614,#58615,#58616,#58617,#58618,#58619,#58620,#58621,#58622,#58623,#58624,
#58625,#58626,#58627,#58628,#58629,#58630,#58631,#58632,#58633,#58634,#58635,
#58636,#58637,#58638,#58639,#58640,#58641,#58642,#58643,#58644,#58645,#58646,
#58647,#58648,#58649,#58650,#58651,#58652,#58653,#58654,#58655,#58656,#58657,
#58658,#58659,#58660,#58661,#58662,#58663,#58664,#58665,#58666,#58667,#58668,
#58669,#58670,#58671),.UNSPECIFIED.,.F.,.F.,(4,3,3,3,3,3,3,3,3,3,3,3,3,
3,3,3,3,3,3,3,3,3,3,3,3,3,3,3,4),(-0.376940817211628,-0.354431931598271,
-0.33291050214917,-0.328061832757599,-0.305813770680128,-0.290194499089435,
-0.284255854807366,-0.277973785325902,-0.256315628127061,-0.235159936382763,
-0.214950283336026,-0.208195454784792,-0.204402290359773,-0.183827312742316,
-0.180862865680239,-0.159776092357818,-0.140305803166316,-0.136023358723937,
-0.132589553322146,-0.112137183595652,-0.0919021865118393,-0.0718392599446326,
-0.0676313463151555,-0.0636633141776788,-0.044090905576146,-0.0251703687379681,
-0.00636244806541706,-0.00328482218945705,0.),.UNSPECIFIED.);
#658=B_SPLINE_CURVE_WITH_KNOTS('',3,(#59088,#59089,#59090,#59091,#59092,
#59093,#59094,#59095,#59096,#59097,#59098,#59099,#59100,#59101,#59102,#59103,
#59104,#59105,#59106,#59107,#59108,#59109,#59110,#59111,#59112,#59113,#59114,
#59115,#59116,#59117,#59118,#59119,#59120,#59121,#59122,#59123,#59124,#59125,
#59126,#59127,#59128,#59129,#59130,#59131,#59132,#59133,#59134,#59135,#59136,
#59137,#59138,#59139,#59140,#59141,#59142,#59143,#59144,#59145,#59146,#59147,
#59148,#59149,#59150,#59151,#59152,#59153,#59154,#59155,#59156,#59157,#59158,
#59159,#59160,#59161,#59162,#59163,#59164,#59165,#59166,#59167,#59168,#59169),
 .UNSPECIFIED.,.F.,.F.,(4,3,3,3,3,3,3,3,3,3,3,3,3,3,3,3,3,3,3,3,3,3,3,3,
3,3,3,4),(0.,0.0186931777979472,0.038069582663444,0.0557727123654966,0.0644773333531983,
0.0684521454610112,0.0885308791156241,0.108995971082426,0.125989856347167,
0.133855323484509,0.137288340283486,0.158362746619097,0.177197233492055,
0.197771878148169,0.205648382326712,0.209124428921397,0.22992781965306,
0.251270152758872,0.269193970891297,0.278737264184526,0.284782300229465,
0.307041766598089,0.322965425288574,0.328171269586608,0.333183333893234,
0.355704745759864,0.37292316965919,0.376894465478604),.UNSPECIFIED.);
#659=B_SPLINE_CURVE_WITH_KNOTS('',3,(#59586,#59587,#59588,#59589,#59590,
#59591,#59592,#59593,#59594,#59595,#59596,#59597,#59598,#59599,#59600,#59601,
#59602,#59603,#59604,#59605,#59606,#59607,#59608,#59609,#59610,#59611,#59612,
#59613,#59614,#59615,#59616,#59617,#59618,#59619,#59620,#59621,#59622,#59623,
#59624,#59625,#59626,#59627,#59628,#59629,#59630,#59631,#59632,#59633,#59634,
#59635,#59636,#59637,#59638,#59639,#59640,#59641,#59642,#59643,#59644,#59645,
#59646,#59647,#59648,#59649,#59650,#59651,#59652,#59653,#59654,#59655,#59656,
#59657,#59658,#59659,#59660,#59661,#59662,#59663,#59664,#59665,#59666,#59667,
#59668,#59669,#59670),.UNSPECIFIED.,.F.,.F.,(4,3,3,3,3,3,3,3,3,3,3,3,3,
3,3,3,3,3,3,3,3,3,3,3,3,3,3,3,4),(1.30794053536005E-15,0.0222065049803711,
0.0447372655622252,0.062893202204516,0.0719711705256613,0.0777843945802568,
0.0810491388468067,0.102995977799722,0.124600763208028,0.142866962546818,
0.150422887918052,0.153918794618638,0.157566976032779,0.17833659004605,
0.197155519647457,0.218478442759019,0.224327897336195,0.229401225301518,
0.250048769456985,0.270748189563912,0.291016884823382,0.296885783013855,
0.300621344353643,0.320441444472329,0.334296858333292,0.338763771301729,
0.357786582134865,0.375324744080583,0.378621596831427),.UNSPECIFIED.);
#942=SHAPE_REPRESENTATION_RELATIONSHIP('SRR','None',#94494,#957);
#957=ADVANCED_BREP_SHAPE_REPRESENTATION('',(#987),#94403);
#972=STYLED_ITEM('',(#94577),#987);
#987=MANIFOLD_SOLID_BREP('Body1',#8257);
#1016=FACE_BOUND('',#1737,.T.);
#1106=PLANE('',#8686);
#1107=PLANE('',#8687);
#1108=PLANE('',#8691);
#1109=PLANE('',#8692);
#1322=FACE_OUTER_BOUND('',#1698,.T.);
#1323=FACE_OUTER_BOUND('',#1699,.T.);
#1324=FACE_OUTER_BOUND('',#1700,.T.);
#1325=FACE_OUTER_BOUND('',#1701,.T.);
#1326=FACE_OUTER_BOUND('',#1702,.T.);
#1327=FACE_OUTER_BOUND('',#1703,.T.);
#1328=FACE_OUTER_BOUND('',#1704,.T.);
#1329=FACE_OUTER_BOUND('',#1705,.T.);
#1330=FACE_OUTER_BOUND('',#1706,.T.);
#1331=FACE_OUTER_BOUND('',#1707,.T.);
#1332=FACE_OUTER_BOUND('',#1708,.T.);
#1333=FACE_OUTER_BOUND('',#1709,.T.);
#1334=FACE_OUTER_BOUND('',#1710,.T.);
#1335=FACE_OUTER_BOUND('',#1711,.T.);
#1336=FACE_OUTER_BOUND('',#1712,.T.);
#1337=FACE_OUTER_BOUND('',#1713,.T.);
#1338=FACE_OUTER_BOUND('',#1714,.T.);
#1339=FACE_OUTER_BOUND('',#1715,.T.);
#1340=FACE_OUTER_BOUND('',#1716,.T.);
#1341=FACE_OUTER_BOUND('',#1717,.T.);
#1342=FACE_OUTER_BOUND('',#1718,.T.);
#1343=FACE_OUTER_BOUND('',#1719,.T.);
#1344=FACE_OUTER_BOUND('',#1720,.T.);
#1345=FACE_OUTER_BOUND('',#1721,.T.);
#1346=FACE_OUTER_BOUND('',#1722,.T.);
#1347=FACE_OUTER_BOUND('',#1723,.T.);
#1348=FACE_OUTER_BOUND('',#1724,.T.);
#1349=FACE_OUTER_BOUND('',#1725,.T.);
#1350=FACE_OUTER_BOUND('',#1726,.T.);
#1351=FACE_OUTER_BOUND('',#1727,.T.);
#1352=FACE_OUTER_BOUND('',#1728,.T.);
#1353=FACE_OUTER_BOUND('',#1729,.T.);
#1354=FACE_OUTER_BOUND('',#1730,.T.);
#1355=FACE_OUTER_BOUND('',#1731,.T.);
#1356=FACE_OUTER_BOUND('',#1732,.T.);
#1357=FACE_OUTER_BOUND('',#1733,.T.);
#1358=FACE_OUTER_BOUND('',#1734,.T.);
#1359=FACE_OUTER_BOUND('',#1735,.T.);
#1360=FACE_OUTER_BOUND('',#1736,.T.);
#1361=FACE_OUTER_BOUND('',#1738,.T.);
#1698=EDGE_LOOP('',(#6320,#6321,#6322,#6323));
#1699=EDGE_LOOP('',(#6324,#6325,#6326,#6327,#6328,#6329));
#1700=EDGE_LOOP('',(#6330,#6331,#6332,#6333,#6334,#6335));
#1701=EDGE_LOOP('',(#6336,#6337,#6338,#6339,#6340,#6341));
#1702=EDGE_LOOP('',(#6342,#6343,#6344,#6345,#6346,#6347));
#1703=EDGE_LOOP('',(#6348,#6349,#6350,#6351,#6352,#6353));
#1704=EDGE_LOOP('',(#6354,#6355,#6356,#6357,#6358,#6359));
#1705=EDGE_LOOP('',(#6360,#6361,#6362,#6363,#6364,#6365));
#1706=EDGE_LOOP('',(#6366,#6367,#6368,#6369,#6370,#6371));
#1707=EDGE_LOOP('',(#6372,#6373,#6374,#6375,#6376,#6377));
#1708=EDGE_LOOP('',(#6378,#6379,#6380,#6381,#6382,#6383));
#1709=EDGE_LOOP('',(#6384,#6385,#6386,#6387,#6388,#6389));
#1710=EDGE_LOOP('',(#6390,#6391,#6392,#6393,#6394,#6395));
#1711=EDGE_LOOP('',(#6396,#6397,#6398,#6399,#6400,#6401));
#1712=EDGE_LOOP('',(#6402,#6403,#6404,#6405,#6406,#6407));
#1713=EDGE_LOOP('',(#6408,#6409,#6410,#6411,#6412,#6413));
#1714=EDGE_LOOP('',(#6414,#6415,#6416,#6417,#6418,#6419,#6420,#6421,#6422));
#1715=EDGE_LOOP('',(#6423,#6424,#6425,#6426,#6427,#6428));
#1716=EDGE_LOOP('',(#6429,#6430,#6431,#6432,#6433,#6434));
#1717=EDGE_LOOP('',(#6435,#6436,#6437,#6438));
#1718=EDGE_LOOP('',(#6439,#6440,#6441,#6442,#6443,#6444));
#1719=EDGE_LOOP('',(#6445,#6446,#6447,#6448));
#1720=EDGE_LOOP('',(#6449,#6450,#6451,#6452,#6453,#6454));
#1721=EDGE_LOOP('',(#6455,#6456,#6457,#6458));
#1722=EDGE_LOOP('',(#6459,#6460,#6461,#6462,#6463,#6464));
#1723=EDGE_LOOP('',(#6465,#6466,#6467,#6468,#6469));
#1724=EDGE_LOOP('',(#6470,#6471,#6472,#6473,#6474));
#1725=EDGE_LOOP('',(#6475,#6476,#6477,#6478,#6479));
#1726=EDGE_LOOP('',(#6480,#6481,#6482,#6483,#6484));
#1727=EDGE_LOOP('',(#6485,#6486,#6487,#6488,#6489));
#1728=EDGE_LOOP('',(#6490,#6491,#6492,#6493,#6494,#6495));
#1729=EDGE_LOOP('',(#6496,#6497,#6498,#6499,#6500));
#1730=EDGE_LOOP('',(#6501,#6502,#6503,#6504,#6505,#6506));
#1731=EDGE_LOOP('',(#6507,#6508,#6509,#6510));
#1732=EDGE_LOOP('',(#6511,#6512,#6513,#6514,#6515,#6516,#6517,#6518,#6519,
#6520,#6521,#6522,#6523,#6524,#6525,#6526,#6527,#6528,#6529,#6530,#6531,
#6532,#6533,#6534,#6535,#6536,#6537,#6538,#6539,#6540,#6541,#6542,#6543,
#6544,#6545,#6546,#6547,#6548,#6549,#6550,#6551,#6552,#6553,#6554,#6555,
#6556,#6557,#6558,#6559,#6560,#6561,#6562,#6563,#6564,#6565,#6566,#6567,
#6568,#6569,#6570,#6571,#6572));
#1733=EDGE_LOOP('',(#6573,#6574,#6575,#6576,#6577,#6578,#6579,#6580,#6581,
#6582,#6583,#6584,#6585,#6586,#6587,#6588,#6589,#6590,#6591,#6592,#6593,
#6594,#6595,#6596,#6597,#6598,#6599,#6600,#6601,#6602,#6603,#6604,#6605,
#6606,#6607,#6608,#6609,#6610,#6611,#6612,#6613,#6614,#6615,#6616,#6617,
#6618,#6619,#6620,#6621,#6622,#6623,#6624,#6625,#6626,#6627,#6628,#6629,
#6630,#6631,#6632));
#1734=EDGE_LOOP('',(#6633));
#1735=EDGE_LOOP('',(#6634,#6635,#6636,#6637));
#1736=EDGE_LOOP('',(#6638));
#1737=EDGE_LOOP('',(#6639,#6640,#6641,#6642));
#1738=EDGE_LOOP('',(#6643));
#2128=LINE('',#48402,#2526);
#2129=LINE('',#48444,#2527);
#2130=LINE('',#48655,#2528);
#2131=LINE('',#48872,#2529);
#2132=LINE('',#49202,#2530);
#2133=LINE('',#49480,#2531);
#2134=LINE('',#49688,#2532);
#2135=LINE('',#50018,#2533);
#2136=LINE('',#50296,#2534);
#2137=LINE('',#50504,#2535);
#2138=LINE('',#50837,#2536);
#2139=LINE('',#51112,#2537);
#2140=LINE('',#51323,#2538);
#2141=LINE('',#51656,#2539);
#2142=LINE('',#51931,#2540);
#2143=LINE('',#52029,#2541);
#2144=LINE('',#52114,#2542);
#2145=LINE('',#52266,#2543);
#2146=LINE('',#52448,#2544);
#2147=LINE('',#52656,#2545);
#2148=LINE('',#53071,#2546);
#2149=LINE('',#53489,#2547);
#2150=LINE('',#53931,#2548);
#2151=LINE('',#54361,#2549);
#2152=LINE('',#54789,#2550);
#2153=LINE('',#55205,#2551);
#2154=LINE('',#55675,#2552);
#2155=LINE('',#56097,#2553);
#2156=LINE('',#56512,#2554);
#2157=LINE('',#56935,#2555);
#2158=LINE('',#57370,#2556);
#2159=LINE('',#57795,#2557);
#2160=LINE('',#59676,#2558);
#2526=VECTOR('',#9572,2.05475);
#2527=VECTOR('',#9577,2.05475);
#2528=VECTOR('',#9580,2.05475);
#2529=VECTOR('',#9583,2.05475);
#2530=VECTOR('',#9586,2.05475);
#2531=VECTOR('',#9589,2.05475);
#2532=VECTOR('',#9592,2.05475);
#2533=VECTOR('',#9595,2.05475);
#2534=VECTOR('',#9598,2.05475);
#2535=VECTOR('',#9601,2.05475);
#2536=VECTOR('',#9604,2.05475);
#2537=VECTOR('',#9607,2.05475);
#2538=VECTOR('',#9610,2.05475);
#2539=VECTOR('',#9613,2.05475);
#2540=VECTOR('',#9616,2.05475);
#2541=VECTOR('',#9619,2.05475);
#2542=VECTOR('',#9624,1.666);
#2543=VECTOR('',#9627,1.666);
#2544=VECTOR('',#9632,1.666);
#2545=VECTOR('',#9635,1.666);
#2546=VECTOR('',#9638,1.666);
#2547=VECTOR('',#9641,1.666);
#2548=VECTOR('',#9644,1.666);
#2549=VECTOR('',#9647,1.666);
#2550=VECTOR('',#9650,1.666);
#2551=VECTOR('',#9653,1.666);
#2552=VECTOR('',#9656,1.666);
#2553=VECTOR('',#9659,1.666);
#2554=VECTOR('',#9662,1.666);
#2555=VECTOR('',#9665,1.666);
#2556=VECTOR('',#9668,1.666);
#2557=VECTOR('',#9671,1.666);
#2558=VECTOR('',#9686,5.);
#2777=CIRCLE('',#8649,2.05475);
#2778=CIRCLE('',#8665,2.05475);
#2779=CIRCLE('',#8667,1.666);
#2780=CIRCLE('',#8668,1.666);
#2781=CIRCLE('',#8683,1.666);
#2782=CIRCLE('',#8689,5.);
#2783=CIRCLE('',#8690,5.);
#3311=VERTEX_POINT('',#48400);
#3312=VERTEX_POINT('',#48401);
#3313=VERTEX_POINT('',#48403);
#3314=VERTEX_POINT('',#48408);
#3315=VERTEX_POINT('',#48442);
#3316=VERTEX_POINT('',#48443);
#3317=VERTEX_POINT('',#48445);
#3318=VERTEX_POINT('',#48573);
#3319=VERTEX_POINT('',#48653);
#3320=VERTEX_POINT('',#48654);
#3321=VERTEX_POINT('',#48656);
#3322=VERTEX_POINT('',#48854);
#3323=VERTEX_POINT('',#48870);
#3324=VERTEX_POINT('',#48871);
#3325=VERTEX_POINT('',#48873);
#3326=VERTEX_POINT('',#49068);
#3327=VERTEX_POINT('',#49200);
#3328=VERTEX_POINT('',#49201);
#3329=VERTEX_POINT('',#49203);
#3330=VERTEX_POINT('',#49282);
#3331=VERTEX_POINT('',#49478);
#3332=VERTEX_POINT('',#49479);
#3333=VERTEX_POINT('',#49481);
#3334=VERTEX_POINT('',#49609);
#3335=VERTEX_POINT('',#49686);
#3336=VERTEX_POINT('',#49687);
#3337=VERTEX_POINT('',#49689);
#3338=VERTEX_POINT('',#49884);
#3339=VERTEX_POINT('',#50016);
#3340=VERTEX_POINT('',#50017);
#3341=VERTEX_POINT('',#50019);
#3342=VERTEX_POINT('',#50095);
#3343=VERTEX_POINT('',#50294);
#3344=VERTEX_POINT('',#50295);
#3345=VERTEX_POINT('',#50297);
#3346=VERTEX_POINT('',#50425);
#3347=VERTEX_POINT('',#50502);
#3348=VERTEX_POINT('',#50503);
#3349=VERTEX_POINT('',#50505);
#3350=VERTEX_POINT('',#50703);
#3351=VERTEX_POINT('',#50835);
#3352=VERTEX_POINT('',#50836);
#3353=VERTEX_POINT('',#50838);
#3354=VERTEX_POINT('',#50914);
#3355=VERTEX_POINT('',#51110);
#3356=VERTEX_POINT('',#51111);
#3357=VERTEX_POINT('',#51113);
#3358=VERTEX_POINT('',#51241);
#3359=VERTEX_POINT('',#51321);
#3360=VERTEX_POINT('',#51322);
#3361=VERTEX_POINT('',#51324);
#3362=VERTEX_POINT('',#51522);
#3363=VERTEX_POINT('',#51654);
#3364=VERTEX_POINT('',#51655);
#3365=VERTEX_POINT('',#51657);
#3366=VERTEX_POINT('',#51733);
#3367=VERTEX_POINT('',#51929);
#3368=VERTEX_POINT('',#51930);
#3369=VERTEX_POINT('',#51932);
#3370=VERTEX_POINT('',#51947);
#3371=VERTEX_POINT('',#52027);
#3372=VERTEX_POINT('',#52028);
#3373=VERTEX_POINT('',#52030);
#3374=VERTEX_POINT('',#52037);
#3375=VERTEX_POINT('',#52043);
#3376=VERTEX_POINT('',#52045);
#3377=VERTEX_POINT('',#52112);
#3378=VERTEX_POINT('',#52113);
#3379=VERTEX_POINT('',#52115);
#3380=VERTEX_POINT('',#52252);
#3381=VERTEX_POINT('',#52254);
#3382=VERTEX_POINT('',#52265);
#3383=VERTEX_POINT('',#52268);
#3384=VERTEX_POINT('',#52446);
#3385=VERTEX_POINT('',#52447);
#3386=VERTEX_POINT('',#52449);
#3387=VERTEX_POINT('',#52629);
#3388=VERTEX_POINT('',#52654);
#3389=VERTEX_POINT('',#52655);
#3390=VERTEX_POINT('',#52657);
#3391=VERTEX_POINT('',#52864);
#3392=VERTEX_POINT('',#53069);
#3393=VERTEX_POINT('',#53070);
#3394=VERTEX_POINT('',#53487);
#3395=VERTEX_POINT('',#53488);
#3396=VERTEX_POINT('',#53490);
#3397=VERTEX_POINT('',#53721);
#3398=VERTEX_POINT('',#53929);
#3399=VERTEX_POINT('',#53930);
#3400=VERTEX_POINT('',#54359);
#3401=VERTEX_POINT('',#54360);
#3402=VERTEX_POINT('',#54362);
#3403=VERTEX_POINT('',#54581);
#3404=VERTEX_POINT('',#54787);
#3405=VERTEX_POINT('',#54788);
#3406=VERTEX_POINT('',#55203);
#3407=VERTEX_POINT('',#55204);
#3408=VERTEX_POINT('',#55206);
#3409=VERTEX_POINT('',#55391);
#3410=VERTEX_POINT('',#55673);
#3411=VERTEX_POINT('',#55674);
#3412=VERTEX_POINT('',#55676);
#3413=VERTEX_POINT('',#56095);
#3414=VERTEX_POINT('',#56096);
#3415=VERTEX_POINT('',#56296);
#3416=VERTEX_POINT('',#56510);
#3417=VERTEX_POINT('',#56511);
#3418=VERTEX_POINT('',#56513);
#3419=VERTEX_POINT('',#56933);
#3420=VERTEX_POINT('',#56934);
#3421=VERTEX_POINT('',#57156);
#3422=VERTEX_POINT('',#57368);
#3423=VERTEX_POINT('',#57369);
#3424=VERTEX_POINT('',#57371);
#3425=VERTEX_POINT('',#57793);
#3426=VERTEX_POINT('',#57794);
#3427=VERTEX_POINT('',#57796);
#3428=VERTEX_POINT('',#57807);
#3429=VERTEX_POINT('',#57917);
#3430=VERTEX_POINT('',#57919);
#3431=VERTEX_POINT('',#58291);
#3432=VERTEX_POINT('',#58468);
#3433=VERTEX_POINT('',#58483);
#3434=VERTEX_POINT('',#59673);
#3435=VERTEX_POINT('',#59675);
#4425=EDGE_CURVE('',#3311,#3312,#2128,.T.);
#4426=EDGE_CURVE('',#3312,#3313,#538,.T.);
#4427=EDGE_CURVE('',#3314,#3313,#2777,.T.);
#4428=EDGE_CURVE('',#3311,#3314,#539,.T.);
#4429=EDGE_CURVE('',#3315,#3316,#2129,.T.);
#4430=EDGE_CURVE('',#3316,#3317,#540,.T.);
#4431=EDGE_CURVE('',#3317,#3312,#541,.T.);
#4432=EDGE_CURVE('',#3318,#3311,#542,.T.);
#4433=EDGE_CURVE('',#3315,#3318,#543,.T.);
#4434=EDGE_CURVE('',#3319,#3320,#2130,.T.);
#4435=EDGE_CURVE('',#3320,#3321,#544,.T.);
#4436=EDGE_CURVE('',#3321,#3316,#545,.T.);
#4437=EDGE_CURVE('',#3322,#3315,#546,.T.);
#4438=EDGE_CURVE('',#3319,#3322,#547,.T.);
#4439=EDGE_CURVE('',#3323,#3324,#2131,.T.);
#4440=EDGE_CURVE('',#3324,#3325,#548,.T.);
#4441=EDGE_CURVE('',#3325,#3320,#549,.T.);
#4442=EDGE_CURVE('',#3326,#3319,#550,.T.);
#4443=EDGE_CURVE('',#3323,#3326,#551,.T.);
#4444=EDGE_CURVE('',#3327,#3328,#2132,.T.);
#4445=EDGE_CURVE('',#3328,#3329,#552,.T.);
#4446=EDGE_CURVE('',#3329,#3324,#553,.T.);
#4447=EDGE_CURVE('',#3330,#3323,#554,.T.);
#4448=EDGE_CURVE('',#3327,#3330,#555,.T.);
#4449=EDGE_CURVE('',#3331,#3332,#2133,.T.);
#4450=EDGE_CURVE('',#3332,#3333,#556,.T.);
#4451=EDGE_CURVE('',#3333,#3328,#557,.T.);
#4452=EDGE_CURVE('',#3334,#3327,#558,.T.);
#4453=EDGE_CURVE('',#3331,#3334,#559,.T.);
#4454=EDGE_CURVE('',#3335,#3336,#2134,.T.);
#4455=EDGE_CURVE('',#3336,#3337,#560,.T.);
#4456=EDGE_CURVE('',#3337,#3332,#561,.T.);
#4457=EDGE_CURVE('',#3338,#3331,#562,.T.);
#4458=EDGE_CURVE('',#3335,#3338,#563,.T.);
#4459=EDGE_CURVE('',#3339,#3340,#2135,.T.);
#4460=EDGE_CURVE('',#3340,#3341,#564,.T.);
#4461=EDGE_CURVE('',#3341,#3336,#565,.T.);
#4462=EDGE_CURVE('',#3342,#3335,#566,.T.);
#4463=EDGE_CURVE('',#3339,#3342,#567,.T.);
#4464=EDGE_CURVE('',#3343,#3344,#2136,.T.);
#4465=EDGE_CURVE('',#3344,#3345,#568,.T.);
#4466=EDGE_CURVE('',#3345,#3340,#569,.T.);
#4467=EDGE_CURVE('',#3346,#3339,#570,.T.);
#4468=EDGE_CURVE('',#3343,#3346,#571,.T.);
#4469=EDGE_CURVE('',#3347,#3348,#2137,.T.);
#4470=EDGE_CURVE('',#3348,#3349,#572,.T.);
#4471=EDGE_CURVE('',#3349,#3344,#573,.T.);
#4472=EDGE_CURVE('',#3350,#3343,#574,.T.);
#4473=EDGE_CURVE('',#3347,#3350,#575,.T.);
#4474=EDGE_CURVE('',#3351,#3352,#2138,.T.);
#4475=EDGE_CURVE('',#3352,#3353,#576,.T.);
#4476=EDGE_CURVE('',#3353,#3348,#577,.T.);
#4477=EDGE_CURVE('',#3354,#3347,#578,.T.);
#4478=EDGE_CURVE('',#3351,#3354,#579,.T.);
#4479=EDGE_CURVE('',#3355,#3356,#2139,.T.);
#4480=EDGE_CURVE('',#3356,#3357,#580,.T.);
#4481=EDGE_CURVE('',#3357,#3352,#581,.T.);
#4482=EDGE_CURVE('',#3358,#3351,#582,.T.);
#4483=EDGE_CURVE('',#3355,#3358,#583,.T.);
#4484=EDGE_CURVE('',#3359,#3360,#2140,.T.);
#4485=EDGE_CURVE('',#3360,#3361,#584,.T.);
#4486=EDGE_CURVE('',#3361,#3356,#585,.T.);
#4487=EDGE_CURVE('',#3362,#3355,#586,.T.);
#4488=EDGE_CURVE('',#3359,#3362,#587,.T.);
#4489=EDGE_CURVE('',#3363,#3364,#2141,.T.);
#4490=EDGE_CURVE('',#3364,#3365,#588,.T.);
#4491=EDGE_CURVE('',#3365,#3360,#589,.T.);
#4492=EDGE_CURVE('',#3366,#3359,#590,.T.);
#4493=EDGE_CURVE('',#3363,#3366,#591,.T.);
#4494=EDGE_CURVE('',#3367,#3368,#2142,.T.);
#4495=EDGE_CURVE('',#3368,#3369,#592,.T.);
#4496=EDGE_CURVE('',#3369,#3364,#593,.T.);
#4497=EDGE_CURVE('',#3370,#3363,#594,.T.);
#4498=EDGE_CURVE('',#3367,#3370,#595,.T.);
#4499=EDGE_CURVE('',#3371,#3372,#2143,.T.);
#4500=EDGE_CURVE('',#3373,#3371,#596,.T.);
#4501=EDGE_CURVE('',#3374,#3373,#597,.T.);
#4502=EDGE_CURVE('',#3375,#3374,#2778,.T.);
#4503=EDGE_CURVE('',#3375,#3376,#598,.T.);
#4504=EDGE_CURVE('',#3376,#3372,#599,.T.);
#4505=EDGE_CURVE('',#3377,#3378,#2144,.T.);
#4506=EDGE_CURVE('',#3378,#3379,#600,.T.);
#4507=EDGE_CURVE('',#3379,#3380,#2779,.T.);
#4508=EDGE_CURVE('',#3380,#3381,#601,.T.);
#4509=EDGE_CURVE('',#3381,#3382,#2145,.T.);
#4510=EDGE_CURVE('',#3382,#3382,#2780,.F.);
#4511=EDGE_CURVE('',#3381,#3383,#602,.T.);
#4512=EDGE_CURVE('',#3383,#3377,#603,.T.);
#4513=EDGE_CURVE('',#3384,#3385,#2146,.T.);
#4514=EDGE_CURVE('',#3385,#3386,#604,.T.);
#4515=EDGE_CURVE('',#3386,#3378,#605,.T.);
#4516=EDGE_CURVE('',#3377,#3387,#606,.T.);
#4517=EDGE_CURVE('',#3387,#3384,#607,.T.);
#4518=EDGE_CURVE('',#3388,#3389,#2147,.T.);
#4519=EDGE_CURVE('',#3389,#3390,#608,.T.);
#4520=EDGE_CURVE('',#3390,#3385,#609,.T.);
#4521=EDGE_CURVE('',#3384,#3391,#610,.T.);
#4522=EDGE_CURVE('',#3391,#3388,#611,.T.);
#4523=EDGE_CURVE('',#3392,#3393,#2148,.T.);
#4524=EDGE_CURVE('',#3393,#3389,#612,.T.);
#4525=EDGE_CURVE('',#3388,#3392,#613,.T.);
#4526=EDGE_CURVE('',#3394,#3395,#2149,.T.);
#4527=EDGE_CURVE('',#3395,#3396,#614,.T.);
#4528=EDGE_CURVE('',#3396,#3393,#615,.T.);
#4529=EDGE_CURVE('',#3392,#3397,#616,.T.);
#4530=EDGE_CURVE('',#3397,#3394,#617,.T.);
#4531=EDGE_CURVE('',#3398,#3399,#2150,.T.);
#4532=EDGE_CURVE('',#3399,#3395,#618,.T.);
#4533=EDGE_CURVE('',#3394,#3398,#619,.T.);
#4534=EDGE_CURVE('',#3400,#3401,#2151,.T.);
#4535=EDGE_CURVE('',#3401,#3402,#620,.T.);
#4536=EDGE_CURVE('',#3402,#3399,#621,.T.);
#4537=EDGE_CURVE('',#3398,#3403,#622,.T.);
#4538=EDGE_CURVE('',#3403,#3400,#623,.T.);
#4539=EDGE_CURVE('',#3404,#3405,#2152,.T.);
#4540=EDGE_CURVE('',#3405,#3401,#624,.T.);
#4541=EDGE_CURVE('',#3400,#3404,#625,.T.);
#4542=EDGE_CURVE('',#3406,#3407,#2153,.T.);
#4543=EDGE_CURVE('',#3407,#3408,#626,.T.);
#4544=EDGE_CURVE('',#3408,#3405,#627,.T.);
#4545=EDGE_CURVE('',#3404,#3409,#628,.T.);
#4546=EDGE_CURVE('',#3409,#3406,#629,.T.);
#4547=EDGE_CURVE('',#3410,#3411,#2154,.T.);
#4548=EDGE_CURVE('',#3411,#3412,#630,.T.);
#4549=EDGE_CURVE('',#3412,#3407,#631,.T.);
#4550=EDGE_CURVE('',#3406,#3410,#632,.T.);
#4551=EDGE_CURVE('',#3413,#3414,#2155,.T.);
#4552=EDGE_CURVE('',#3414,#3411,#633,.T.);
#4553=EDGE_CURVE('',#3410,#3415,#634,.T.);
#4554=EDGE_CURVE('',#3415,#3413,#635,.T.);
#4555=EDGE_CURVE('',#3416,#3417,#2156,.T.);
#4556=EDGE_CURVE('',#3417,#3418,#636,.T.);
#4557=EDGE_CURVE('',#3418,#3414,#637,.T.);
#4558=EDGE_CURVE('',#3413,#3416,#638,.T.);
#4559=EDGE_CURVE('',#3419,#3420,#2157,.T.);
#4560=EDGE_CURVE('',#3420,#3417,#639,.T.);
#4561=EDGE_CURVE('',#3416,#3421,#640,.T.);
#4562=EDGE_CURVE('',#3421,#3419,#641,.T.);
#4563=EDGE_CURVE('',#3422,#3423,#2158,.T.);
#4564=EDGE_CURVE('',#3423,#3424,#642,.T.);
#4565=EDGE_CURVE('',#3424,#3420,#643,.T.);
#4566=EDGE_CURVE('',#3419,#3422,#644,.T.);
#4567=EDGE_CURVE('',#3425,#3426,#2159,.T.);
#4568=EDGE_CURVE('',#3425,#3427,#645,.T.);
#4569=EDGE_CURVE('',#3427,#3428,#646,.T.);
#4570=EDGE_CURVE('',#3429,#3428,#2781,.T.);
#4571=EDGE_CURVE('',#3429,#3430,#647,.T.);
#4572=EDGE_CURVE('',#3430,#3426,#648,.T.);
#4573=EDGE_CURVE('',#3426,#3423,#649,.T.);
#4574=EDGE_CURVE('',#3422,#3431,#650,.T.);
#4575=EDGE_CURVE('',#3431,#3425,#651,.T.);
#4576=EDGE_CURVE('',#3372,#3432,#652,.T.);
#4577=EDGE_CURVE('',#3432,#3368,#653,.T.);
#4578=EDGE_CURVE('',#3433,#3367,#654,.T.);
#4579=EDGE_CURVE('',#3371,#3433,#655,.T.);
#4580=EDGE_CURVE('',#3379,#3314,#656,.T.);
#4581=EDGE_CURVE('',#3313,#3380,#657,.T.);
#4582=EDGE_CURVE('',#3428,#3375,#658,.T.);
#4583=EDGE_CURVE('',#3374,#3429,#659,.T.);
#4584=EDGE_CURVE('',#3434,#3434,#2782,.T.);
#4585=EDGE_CURVE('',#3434,#3435,#2160,.T.);
#4586=EDGE_CURVE('',#3435,#3435,#2783,.T.);
#6320=ORIENTED_EDGE('',*,*,#4425,.T.);
#6321=ORIENTED_EDGE('',*,*,#4426,.T.);
#6322=ORIENTED_EDGE('',*,*,#4427,.F.);
#6323=ORIENTED_EDGE('',*,*,#4428,.F.);
#6324=ORIENTED_EDGE('',*,*,#4429,.T.);
#6325=ORIENTED_EDGE('',*,*,#4430,.T.);
#6326=ORIENTED_EDGE('',*,*,#4431,.T.);
#6327=ORIENTED_EDGE('',*,*,#4425,.F.);
#6328=ORIENTED_EDGE('',*,*,#4432,.F.);
#6329=ORIENTED_EDGE('',*,*,#4433,.F.);
#6330=ORIENTED_EDGE('',*,*,#4434,.T.);
#6331=ORIENTED_EDGE('',*,*,#4435,.T.);
#6332=ORIENTED_EDGE('',*,*,#4436,.T.);
#6333=ORIENTED_EDGE('',*,*,#4429,.F.);
#6334=ORIENTED_EDGE('',*,*,#4437,.F.);
#6335=ORIENTED_EDGE('',*,*,#4438,.F.);
#6336=ORIENTED_EDGE('',*,*,#4439,.T.);
#6337=ORIENTED_EDGE('',*,*,#4440,.T.);
#6338=ORIENTED_EDGE('',*,*,#4441,.T.);
#6339=ORIENTED_EDGE('',*,*,#4434,.F.);
#6340=ORIENTED_EDGE('',*,*,#4442,.F.);
#6341=ORIENTED_EDGE('',*,*,#4443,.F.);
#6342=ORIENTED_EDGE('',*,*,#4444,.T.);
#6343=ORIENTED_EDGE('',*,*,#4445,.T.);
#6344=ORIENTED_EDGE('',*,*,#4446,.T.);
#6345=ORIENTED_EDGE('',*,*,#4439,.F.);
#6346=ORIENTED_EDGE('',*,*,#4447,.F.);
#6347=ORIENTED_EDGE('',*,*,#4448,.F.);
#6348=ORIENTED_EDGE('',*,*,#4449,.T.);
#6349=ORIENTED_EDGE('',*,*,#4450,.T.);
#6350=ORIENTED_EDGE('',*,*,#4451,.T.);
#6351=ORIENTED_EDGE('',*,*,#4444,.F.);
#6352=ORIENTED_EDGE('',*,*,#4452,.F.);
#6353=ORIENTED_EDGE('',*,*,#4453,.F.);
#6354=ORIENTED_EDGE('',*,*,#4454,.T.);
#6355=ORIENTED_EDGE('',*,*,#4455,.T.);
#6356=ORIENTED_EDGE('',*,*,#4456,.T.);
#6357=ORIENTED_EDGE('',*,*,#4449,.F.);
#6358=ORIENTED_EDGE('',*,*,#4457,.F.);
#6359=ORIENTED_EDGE('',*,*,#4458,.F.);
#6360=ORIENTED_EDGE('',*,*,#4459,.T.);
#6361=ORIENTED_EDGE('',*,*,#4460,.T.);
#6362=ORIENTED_EDGE('',*,*,#4461,.T.);
#6363=ORIENTED_EDGE('',*,*,#4454,.F.);
#6364=ORIENTED_EDGE('',*,*,#4462,.F.);
#6365=ORIENTED_EDGE('',*,*,#4463,.F.);
#6366=ORIENTED_EDGE('',*,*,#4464,.T.);
#6367=ORIENTED_EDGE('',*,*,#4465,.T.);
#6368=ORIENTED_EDGE('',*,*,#4466,.T.);
#6369=ORIENTED_EDGE('',*,*,#4459,.F.);
#6370=ORIENTED_EDGE('',*,*,#4467,.F.);
#6371=ORIENTED_EDGE('',*,*,#4468,.F.);
#6372=ORIENTED_EDGE('',*,*,#4469,.T.);
#6373=ORIENTED_EDGE('',*,*,#4470,.T.);
#6374=ORIENTED_EDGE('',*,*,#4471,.T.);
#6375=ORIENTED_EDGE('',*,*,#4464,.F.);
#6376=ORIENTED_EDGE('',*,*,#4472,.F.);
#6377=ORIENTED_EDGE('',*,*,#4473,.F.);
#6378=ORIENTED_EDGE('',*,*,#4474,.T.);
#6379=ORIENTED_EDGE('',*,*,#4475,.T.);
#6380=ORIENTED_EDGE('',*,*,#4476,.T.);
#6381=ORIENTED_EDGE('',*,*,#4469,.F.);
#6382=ORIENTED_EDGE('',*,*,#4477,.F.);
#6383=ORIENTED_EDGE('',*,*,#4478,.F.);
#6384=ORIENTED_EDGE('',*,*,#4479,.T.);
#6385=ORIENTED_EDGE('',*,*,#4480,.T.);
#6386=ORIENTED_EDGE('',*,*,#4481,.T.);
#6387=ORIENTED_EDGE('',*,*,#4474,.F.);
#6388=ORIENTED_EDGE('',*,*,#4482,.F.);
#6389=ORIENTED_EDGE('',*,*,#4483,.F.);
#6390=ORIENTED_EDGE('',*,*,#4484,.T.);
#6391=ORIENTED_EDGE('',*,*,#4485,.T.);
#6392=ORIENTED_EDGE('',*,*,#4486,.T.);
#6393=ORIENTED_EDGE('',*,*,#4479,.F.);
#6394=ORIENTED_EDGE('',*,*,#4487,.F.);
#6395=ORIENTED_EDGE('',*,*,#4488,.F.);
#6396=ORIENTED_EDGE('',*,*,#4489,.T.);
#6397=ORIENTED_EDGE('',*,*,#4490,.T.);
#6398=ORIENTED_EDGE('',*,*,#4491,.T.);
#6399=ORIENTED_EDGE('',*,*,#4484,.F.);
#6400=ORIENTED_EDGE('',*,*,#4492,.F.);
#6401=ORIENTED_EDGE('',*,*,#4493,.F.);
#6402=ORIENTED_EDGE('',*,*,#4494,.T.);
#6403=ORIENTED_EDGE('',*,*,#4495,.T.);
#6404=ORIENTED_EDGE('',*,*,#4496,.T.);
#6405=ORIENTED_EDGE('',*,*,#4489,.F.);
#6406=ORIENTED_EDGE('',*,*,#4497,.F.);
#6407=ORIENTED_EDGE('',*,*,#4498,.F.);
#6408=ORIENTED_EDGE('',*,*,#4499,.F.);
#6409=ORIENTED_EDGE('',*,*,#4500,.F.);
#6410=ORIENTED_EDGE('',*,*,#4501,.F.);
#6411=ORIENTED_EDGE('',*,*,#4502,.F.);
#6412=ORIENTED_EDGE('',*,*,#4503,.T.);
#6413=ORIENTED_EDGE('',*,*,#4504,.T.);
#6414=ORIENTED_EDGE('',*,*,#4505,.T.);
#6415=ORIENTED_EDGE('',*,*,#4506,.T.);
#6416=ORIENTED_EDGE('',*,*,#4507,.T.);
#6417=ORIENTED_EDGE('',*,*,#4508,.T.);
#6418=ORIENTED_EDGE('',*,*,#4509,.T.);
#6419=ORIENTED_EDGE('',*,*,#4510,.T.);
#6420=ORIENTED_EDGE('',*,*,#4509,.F.);
#6421=ORIENTED_EDGE('',*,*,#4511,.T.);
#6422=ORIENTED_EDGE('',*,*,#4512,.T.);
#6423=ORIENTED_EDGE('',*,*,#4513,.T.);
#6424=ORIENTED_EDGE('',*,*,#4514,.T.);
#6425=ORIENTED_EDGE('',*,*,#4515,.T.);
#6426=ORIENTED_EDGE('',*,*,#4505,.F.);
#6427=ORIENTED_EDGE('',*,*,#4516,.T.);
#6428=ORIENTED_EDGE('',*,*,#4517,.T.);
#6429=ORIENTED_EDGE('',*,*,#4518,.T.);
#6430=ORIENTED_EDGE('',*,*,#4519,.T.);
#6431=ORIENTED_EDGE('',*,*,#4520,.T.);
#6432=ORIENTED_EDGE('',*,*,#4513,.F.);
#6433=ORIENTED_EDGE('',*,*,#4521,.T.);
#6434=ORIENTED_EDGE('',*,*,#4522,.T.);
#6435=ORIENTED_EDGE('',*,*,#4523,.T.);
#6436=ORIENTED_EDGE('',*,*,#4524,.T.);
#6437=ORIENTED_EDGE('',*,*,#4518,.F.);
#6438=ORIENTED_EDGE('',*,*,#4525,.T.);
#6439=ORIENTED_EDGE('',*,*,#4526,.T.);
#6440=ORIENTED_EDGE('',*,*,#4527,.T.);
#6441=ORIENTED_EDGE('',*,*,#4528,.T.);
#6442=ORIENTED_EDGE('',*,*,#4523,.F.);
#6443=ORIENTED_EDGE('',*,*,#4529,.T.);
#6444=ORIENTED_EDGE('',*,*,#4530,.T.);
#6445=ORIENTED_EDGE('',*,*,#4531,.T.);
#6446=ORIENTED_EDGE('',*,*,#4532,.T.);
#6447=ORIENTED_EDGE('',*,*,#4526,.F.);
#6448=ORIENTED_EDGE('',*,*,#4533,.T.);
#6449=ORIENTED_EDGE('',*,*,#4534,.T.);
#6450=ORIENTED_EDGE('',*,*,#4535,.T.);
#6451=ORIENTED_EDGE('',*,*,#4536,.T.);
#6452=ORIENTED_EDGE('',*,*,#4531,.F.);
#6453=ORIENTED_EDGE('',*,*,#4537,.T.);
#6454=ORIENTED_EDGE('',*,*,#4538,.T.);
#6455=ORIENTED_EDGE('',*,*,#4539,.T.);
#6456=ORIENTED_EDGE('',*,*,#4540,.T.);
#6457=ORIENTED_EDGE('',*,*,#4534,.F.);
#6458=ORIENTED_EDGE('',*,*,#4541,.T.);
#6459=ORIENTED_EDGE('',*,*,#4542,.T.);
#6460=ORIENTED_EDGE('',*,*,#4543,.T.);
#6461=ORIENTED_EDGE('',*,*,#4544,.T.);
#6462=ORIENTED_EDGE('',*,*,#4539,.F.);
#6463=ORIENTED_EDGE('',*,*,#4545,.T.);
#6464=ORIENTED_EDGE('',*,*,#4546,.T.);
#6465=ORIENTED_EDGE('',*,*,#4547,.T.);
#6466=ORIENTED_EDGE('',*,*,#4548,.T.);
#6467=ORIENTED_EDGE('',*,*,#4549,.T.);
#6468=ORIENTED_EDGE('',*,*,#4542,.F.);
#6469=ORIENTED_EDGE('',*,*,#4550,.T.);
#6470=ORIENTED_EDGE('',*,*,#4551,.T.);
#6471=ORIENTED_EDGE('',*,*,#4552,.T.);
#6472=ORIENTED_EDGE('',*,*,#4547,.F.);
#6473=ORIENTED_EDGE('',*,*,#4553,.T.);
#6474=ORIENTED_EDGE('',*,*,#4554,.T.);
#6475=ORIENTED_EDGE('',*,*,#4555,.T.);
#6476=ORIENTED_EDGE('',*,*,#4556,.T.);
#6477=ORIENTED_EDGE('',*,*,#4557,.T.);
#6478=ORIENTED_EDGE('',*,*,#4551,.F.);
#6479=ORIENTED_EDGE('',*,*,#4558,.T.);
#6480=ORIENTED_EDGE('',*,*,#4559,.T.);
#6481=ORIENTED_EDGE('',*,*,#4560,.T.);
#6482=ORIENTED_EDGE('',*,*,#4555,.F.);
#6483=ORIENTED_EDGE('',*,*,#4561,.T.);
#6484=ORIENTED_EDGE('',*,*,#4562,.T.);
#6485=ORIENTED_EDGE('',*,*,#4563,.T.);
#6486=ORIENTED_EDGE('',*,*,#4564,.T.);
#6487=ORIENTED_EDGE('',*,*,#4565,.T.);
#6488=ORIENTED_EDGE('',*,*,#4559,.F.);
#6489=ORIENTED_EDGE('',*,*,#4566,.T.);
#6490=ORIENTED_EDGE('',*,*,#4567,.F.);
#6491=ORIENTED_EDGE('',*,*,#4568,.T.);
#6492=ORIENTED_EDGE('',*,*,#4569,.T.);
#6493=ORIENTED_EDGE('',*,*,#4570,.F.);
#6494=ORIENTED_EDGE('',*,*,#4571,.T.);
#6495=ORIENTED_EDGE('',*,*,#4572,.T.);
#6496=ORIENTED_EDGE('',*,*,#4567,.T.);
#6497=ORIENTED_EDGE('',*,*,#4573,.T.);
#6498=ORIENTED_EDGE('',*,*,#4563,.F.);
#6499=ORIENTED_EDGE('',*,*,#4574,.T.);
#6500=ORIENTED_EDGE('',*,*,#4575,.T.);
#6501=ORIENTED_EDGE('',*,*,#4499,.T.);
#6502=ORIENTED_EDGE('',*,*,#4576,.T.);
#6503=ORIENTED_EDGE('',*,*,#4577,.T.);
#6504=ORIENTED_EDGE('',*,*,#4494,.F.);
#6505=ORIENTED_EDGE('',*,*,#4578,.F.);
#6506=ORIENTED_EDGE('',*,*,#4579,.F.);
#6507=ORIENTED_EDGE('',*,*,#4507,.F.);
#6508=ORIENTED_EDGE('',*,*,#4580,.T.);
#6509=ORIENTED_EDGE('',*,*,#4427,.T.);
#6510=ORIENTED_EDGE('',*,*,#4581,.T.);
#6511=ORIENTED_EDGE('',*,*,#4581,.F.);
#6512=ORIENTED_EDGE('',*,*,#4426,.F.);
#6513=ORIENTED_EDGE('',*,*,#4431,.F.);
#6514=ORIENTED_EDGE('',*,*,#4430,.F.);
#6515=ORIENTED_EDGE('',*,*,#4436,.F.);
#6516=ORIENTED_EDGE('',*,*,#4435,.F.);
#6517=ORIENTED_EDGE('',*,*,#4441,.F.);
#6518=ORIENTED_EDGE('',*,*,#4440,.F.);
#6519=ORIENTED_EDGE('',*,*,#4446,.F.);
#6520=ORIENTED_EDGE('',*,*,#4445,.F.);
#6521=ORIENTED_EDGE('',*,*,#4451,.F.);
#6522=ORIENTED_EDGE('',*,*,#4450,.F.);
#6523=ORIENTED_EDGE('',*,*,#4456,.F.);
#6524=ORIENTED_EDGE('',*,*,#4455,.F.);
#6525=ORIENTED_EDGE('',*,*,#4461,.F.);
#6526=ORIENTED_EDGE('',*,*,#4460,.F.);
#6527=ORIENTED_EDGE('',*,*,#4466,.F.);
#6528=ORIENTED_EDGE('',*,*,#4465,.F.);
#6529=ORIENTED_EDGE('',*,*,#4471,.F.);
#6530=ORIENTED_EDGE('',*,*,#4470,.F.);
#6531=ORIENTED_EDGE('',*,*,#4476,.F.);
#6532=ORIENTED_EDGE('',*,*,#4475,.F.);
#6533=ORIENTED_EDGE('',*,*,#4481,.F.);
#6534=ORIENTED_EDGE('',*,*,#4480,.F.);
#6535=ORIENTED_EDGE('',*,*,#4486,.F.);
#6536=ORIENTED_EDGE('',*,*,#4485,.F.);
#6537=ORIENTED_EDGE('',*,*,#4491,.F.);
#6538=ORIENTED_EDGE('',*,*,#4490,.F.);
#6539=ORIENTED_EDGE('',*,*,#4496,.F.);
#6540=ORIENTED_EDGE('',*,*,#4495,.F.);
#6541=ORIENTED_EDGE('',*,*,#4577,.F.);
#6542=ORIENTED_EDGE('',*,*,#4576,.F.);
#6543=ORIENTED_EDGE('',*,*,#4504,.F.);
#6544=ORIENTED_EDGE('',*,*,#4503,.F.);
#6545=ORIENTED_EDGE('',*,*,#4582,.F.);
#6546=ORIENTED_EDGE('',*,*,#4569,.F.);
#6547=ORIENTED_EDGE('',*,*,#4568,.F.);
#6548=ORIENTED_EDGE('',*,*,#4575,.F.);
#6549=ORIENTED_EDGE('',*,*,#4574,.F.);
#6550=ORIENTED_EDGE('',*,*,#4566,.F.);
#6551=ORIENTED_EDGE('',*,*,#4562,.F.);
#6552=ORIENTED_EDGE('',*,*,#4561,.F.);
#6553=ORIENTED_EDGE('',*,*,#4558,.F.);
#6554=ORIENTED_EDGE('',*,*,#4554,.F.);
#6555=ORIENTED_EDGE('',*,*,#4553,.F.);
#6556=ORIENTED_EDGE('',*,*,#4550,.F.);
#6557=ORIENTED_EDGE('',*,*,#4546,.F.);
#6558=ORIENTED_EDGE('',*,*,#4545,.F.);
#6559=ORIENTED_EDGE('',*,*,#4541,.F.);
#6560=ORIENTED_EDGE('',*,*,#4538,.F.);
#6561=ORIENTED_EDGE('',*,*,#4537,.F.);
#6562=ORIENTED_EDGE('',*,*,#4533,.F.);
#6563=ORIENTED_EDGE('',*,*,#4530,.F.);
#6564=ORIENTED_EDGE('',*,*,#4529,.F.);
#6565=ORIENTED_EDGE('',*,*,#4525,.F.);
#6566=ORIENTED_EDGE('',*,*,#4522,.F.);
#6567=ORIENTED_EDGE('',*,*,#4521,.F.);
#6568=ORIENTED_EDGE('',*,*,#4517,.F.);
#6569=ORIENTED_EDGE('',*,*,#4516,.F.);
#6570=ORIENTED_EDGE('',*,*,#4512,.F.);
#6571=ORIENTED_EDGE('',*,*,#4511,.F.);
#6572=ORIENTED_EDGE('',*,*,#4508,.F.);
#6573=ORIENTED_EDGE('',*,*,#4580,.F.);
#6574=ORIENTED_EDGE('',*,*,#4506,.F.);
#6575=ORIENTED_EDGE('',*,*,#4515,.F.);
#6576=ORIENTED_EDGE('',*,*,#4514,.F.);
#6577=ORIENTED_EDGE('',*,*,#4520,.F.);
#6578=ORIENTED_EDGE('',*,*,#4519,.F.);
#6579=ORIENTED_EDGE('',*,*,#4524,.F.);
#6580=ORIENTED_EDGE('',*,*,#4528,.F.);
#6581=ORIENTED_EDGE('',*,*,#4527,.F.);
#6582=ORIENTED_EDGE('',*,*,#4532,.F.);
#6583=ORIENTED_EDGE('',*,*,#4536,.F.);
#6584=ORIENTED_EDGE('',*,*,#4535,.F.);
#6585=ORIENTED_EDGE('',*,*,#4540,.F.);
#6586=ORIENTED_EDGE('',*,*,#4544,.F.);
#6587=ORIENTED_EDGE('',*,*,#4543,.F.);
#6588=ORIENTED_EDGE('',*,*,#4549,.F.);
#6589=ORIENTED_EDGE('',*,*,#4548,.F.);
#6590=ORIENTED_EDGE('',*,*,#4552,.F.);
#6591=ORIENTED_EDGE('',*,*,#4557,.F.);
#6592=ORIENTED_EDGE('',*,*,#4556,.F.);
#6593=ORIENTED_EDGE('',*,*,#4560,.F.);
#6594=ORIENTED_EDGE('',*,*,#4565,.F.);
#6595=ORIENTED_EDGE('',*,*,#4564,.F.);
#6596=ORIENTED_EDGE('',*,*,#4573,.F.);
#6597=ORIENTED_EDGE('',*,*,#4572,.F.);
#6598=ORIENTED_EDGE('',*,*,#4571,.F.);
#6599=ORIENTED_EDGE('',*,*,#4583,.F.);
#6600=ORIENTED_EDGE('',*,*,#4501,.T.);
#6601=ORIENTED_EDGE('',*,*,#4500,.T.);
#6602=ORIENTED_EDGE('',*,*,#4579,.T.);
#6603=ORIENTED_EDGE('',*,*,#4578,.T.);
#6604=ORIENTED_EDGE('',*,*,#4498,.T.);
#6605=ORIENTED_EDGE('',*,*,#4497,.T.);
#6606=ORIENTED_EDGE('',*,*,#4493,.T.);
#6607=ORIENTED_EDGE('',*,*,#4492,.T.);
#6608=ORIENTED_EDGE('',*,*,#4488,.T.);
#6609=ORIENTED_EDGE('',*,*,#4487,.T.);
#6610=ORIENTED_EDGE('',*,*,#4483,.T.);
#6611=ORIENTED_EDGE('',*,*,#4482,.T.);
#6612=ORIENTED_EDGE('',*,*,#4478,.T.);
#6613=ORIENTED_EDGE('',*,*,#4477,.T.);
#6614=ORIENTED_EDGE('',*,*,#4473,.T.);
#6615=ORIENTED_EDGE('',*,*,#4472,.T.);
#6616=ORIENTED_EDGE('',*,*,#4468,.T.);
#6617=ORIENTED_EDGE('',*,*,#4467,.T.);
#6618=ORIENTED_EDGE('',*,*,#4463,.T.);
#6619=ORIENTED_EDGE('',*,*,#4462,.T.);
#6620=ORIENTED_EDGE('',*,*,#4458,.T.);
#6621=ORIENTED_EDGE('',*,*,#4457,.T.);
#6622=ORIENTED_EDGE('',*,*,#4453,.T.);
#6623=ORIENTED_EDGE('',*,*,#4452,.T.);
#6624=ORIENTED_EDGE('',*,*,#4448,.T.);
#6625=ORIENTED_EDGE('',*,*,#4447,.T.);
#6626=ORIENTED_EDGE('',*,*,#4443,.T.);
#6627=ORIENTED_EDGE('',*,*,#4442,.T.);
#6628=ORIENTED_EDGE('',*,*,#4438,.T.);
#6629=ORIENTED_EDGE('',*,*,#4437,.T.);
#6630=ORIENTED_EDGE('',*,*,#4433,.T.);
#6631=ORIENTED_EDGE('',*,*,#4432,.T.);
#6632=ORIENTED_EDGE('',*,*,#4428,.T.);
#6633=ORIENTED_EDGE('',*,*,#4510,.F.);
#6634=ORIENTED_EDGE('',*,*,#4584,.F.);
#6635=ORIENTED_EDGE('',*,*,#4585,.T.);
#6636=ORIENTED_EDGE('',*,*,#4586,.T.);
#6637=ORIENTED_EDGE('',*,*,#4585,.F.);
#6638=ORIENTED_EDGE('',*,*,#4584,.T.);
#6639=ORIENTED_EDGE('',*,*,#4583,.T.);
#6640=ORIENTED_EDGE('',*,*,#4570,.T.);
#6641=ORIENTED_EDGE('',*,*,#4582,.T.);
#6642=ORIENTED_EDGE('',*,*,#4502,.T.);
#6643=ORIENTED_EDGE('',*,*,#4586,.F.);
#7767=CYLINDRICAL_SURFACE('',#8648,2.05475);
#7768=CYLINDRICAL_SURFACE('',#8650,2.05475);
#7769=CYLINDRICAL_SURFACE('',#8651,2.05475);
#7770=CYLINDRICAL_SURFACE('',#8652,2.05475);
#7771=CYLINDRICAL_SURFACE('',#8653,2.05475);
#7772=CYLINDRICAL_SURFACE('',#8654,2.05475);
#7773=CYLINDRICAL_SURFACE('',#8655,2.05475);
#7774=CYLINDRICAL_SURFACE('',#8656,2.05475);
#7775=CYLINDRICAL_SURFACE('',#8657,2.05475);
#7776=CYLINDRICAL_SURFACE('',#8658,2.05475);
#7777=CYLINDRICAL_SURFACE('',#8659,2.05475);
#7778=CYLINDRICAL_SURFACE('',#8660,2.05475);
#7779=CYLINDRICAL_SURFACE('',#8661,2.05475);
#7780=CYLINDRICAL_SURFACE('',#8662,2.05475);
#7781=CYLINDRICAL_SURFACE('',#8663,2.05475);
#7782=CYLINDRICAL_SURFACE('',#8664,2.05475);
#7783=CYLINDRICAL_SURFACE('',#8666,1.666);
#7784=CYLINDRICAL_SURFACE('',#8669,1.666);
#7785=CYLINDRICAL_SURFACE('',#8670,1.666);
#7786=CYLINDRICAL_SURFACE('',#8671,1.666);
#7787=CYLINDRICAL_SURFACE('',#8672,1.666);
#7788=CYLINDRICAL_SURFACE('',#8673,1.666);
#7789=CYLINDRICAL_SURFACE('',#8674,1.666);
#7790=CYLINDRICAL_SURFACE('',#8675,1.666);
#7791=CYLINDRICAL_SURFACE('',#8676,1.666);
#7792=CYLINDRICAL_SURFACE('',#8677,1.666);
#7793=CYLINDRICAL_SURFACE('',#8678,1.666);
#7794=CYLINDRICAL_SURFACE('',#8679,1.666);
#7795=CYLINDRICAL_SURFACE('',#8680,1.666);
#7796=CYLINDRICAL_SURFACE('',#8681,1.666);
#7797=CYLINDRICAL_SURFACE('',#8682,1.666);
#7798=CYLINDRICAL_SURFACE('',#8684,1.666);
#7799=CYLINDRICAL_SURFACE('',#8685,2.05475);
#7800=CYLINDRICAL_SURFACE('',#8688,5.);
#8059=ADVANCED_FACE('',(#1322),#7767,.F.);
#8060=ADVANCED_FACE('',(#1323),#7768,.F.);
#8061=ADVANCED_FACE('',(#1324),#7769,.F.);
#8062=ADVANCED_FACE('',(#1325),#7770,.F.);
#8063=ADVANCED_FACE('',(#1326),#7771,.F.);
#8064=ADVANCED_FACE('',(#1327),#7772,.F.);
#8065=ADVANCED_FACE('',(#1328),#7773,.F.);
#8066=ADVANCED_FACE('',(#1329),#7774,.F.);
#8067=ADVANCED_FACE('',(#1330),#7775,.F.);
#8068=ADVANCED_FACE('',(#1331),#7776,.F.);
#8069=ADVANCED_FACE('',(#1332),#7777,.F.);
#8070=ADVANCED_FACE('',(#1333),#7778,.F.);
#8071=ADVANCED_FACE('',(#1334),#7779,.F.);
#8072=ADVANCED_FACE('',(#1335),#7780,.F.);
#8073=ADVANCED_FACE('',(#1336),#7781,.F.);
#8074=ADVANCED_FACE('',(#1337),#7782,.F.);
#8075=ADVANCED_FACE('',(#1338),#7783,.F.);
#8076=ADVANCED_FACE('',(#1339),#7784,.F.);
#8077=ADVANCED_FACE('',(#1340),#7785,.F.);
#8078=ADVANCED_FACE('',(#1341),#7786,.F.);
#8079=ADVANCED_FACE('',(#1342),#7787,.F.);
#8080=ADVANCED_FACE('',(#1343),#7788,.F.);
#8081=ADVANCED_FACE('',(#1344),#7789,.F.);
#8082=ADVANCED_FACE('',(#1345),#7790,.F.);
#8083=ADVANCED_FACE('',(#1346),#7791,.F.);
#8084=ADVANCED_FACE('',(#1347),#7792,.F.);
#8085=ADVANCED_FACE('',(#1348),#7793,.F.);
#8086=ADVANCED_FACE('',(#1349),#7794,.F.);
#8087=ADVANCED_FACE('',(#1350),#7795,.F.);
#8088=ADVANCED_FACE('',(#1351),#7796,.F.);
#8089=ADVANCED_FACE('',(#1352),#7797,.F.);
#8090=ADVANCED_FACE('',(#1353),#7798,.F.);
#8091=ADVANCED_FACE('',(#1354),#7799,.F.);
#8092=ADVANCED_FACE('',(#1355),#1106,.T.);
#8093=ADVANCED_FACE('',(#1356),#160,.F.);
#8094=ADVANCED_FACE('',(#1357),#161,.F.);
#8095=ADVANCED_FACE('',(#1358),#1107,.F.);
#8096=ADVANCED_FACE('',(#1359),#7800,.T.);
#8097=ADVANCED_FACE('',(#1360,#1016),#1108,.T.);
#8098=ADVANCED_FACE('',(#1361),#1109,.F.);
#8257=CLOSED_SHELL('',(#8059,#8060,#8061,#8062,#8063,#8064,#8065,#8066,
#8067,#8068,#8069,#8070,#8071,#8072,#8073,#8074,#8075,#8076,#8077,#8078,
#8079,#8080,#8081,#8082,#8083,#8084,#8085,#8086,#8087,#8088,#8089,#8090,
#8091,#8092,#8093,#8094,#8095,#8096,#8097,#8098));
#8647=AXIS2_PLACEMENT_3D('',#48398,#9568,#9569);
#8648=AXIS2_PLACEMENT_3D('',#48399,#9570,#9571);
#8649=AXIS2_PLACEMENT_3D('',#48409,#9573,#9574);
#8650=AXIS2_PLACEMENT_3D('',#48441,#9575,#9576);
#8651=AXIS2_PLACEMENT_3D('',#48652,#9578,#9579);
#8652=AXIS2_PLACEMENT_3D('',#48869,#9581,#9582);
#8653=AXIS2_PLACEMENT_3D('',#49199,#9584,#9585);
#8654=AXIS2_PLACEMENT_3D('',#49477,#9587,#9588);
#8655=AXIS2_PLACEMENT_3D('',#49685,#9590,#9591);
#8656=AXIS2_PLACEMENT_3D('',#50015,#9593,#9594);
#8657=AXIS2_PLACEMENT_3D('',#50293,#9596,#9597);
#8658=AXIS2_PLACEMENT_3D('',#50501,#9599,#9600);
#8659=AXIS2_PLACEMENT_3D('',#50834,#9602,#9603);
#8660=AXIS2_PLACEMENT_3D('',#51109,#9605,#9606);
#8661=AXIS2_PLACEMENT_3D('',#51320,#9608,#9609);
#8662=AXIS2_PLACEMENT_3D('',#51653,#9611,#9612);
#8663=AXIS2_PLACEMENT_3D('',#51928,#9614,#9615);
#8664=AXIS2_PLACEMENT_3D('',#52026,#9617,#9618);
#8665=AXIS2_PLACEMENT_3D('',#52044,#9620,#9621);
#8666=AXIS2_PLACEMENT_3D('',#52111,#9622,#9623);
#8667=AXIS2_PLACEMENT_3D('',#52253,#9625,#9626);
#8668=AXIS2_PLACEMENT_3D('',#52267,#9628,#9629);
#8669=AXIS2_PLACEMENT_3D('',#52445,#9630,#9631);
#8670=AXIS2_PLACEMENT_3D('',#52653,#9633,#9634);
#8671=AXIS2_PLACEMENT_3D('',#53068,#9636,#9637);
#8672=AXIS2_PLACEMENT_3D('',#53486,#9639,#9640);
#8673=AXIS2_PLACEMENT_3D('',#53928,#9642,#9643);
#8674=AXIS2_PLACEMENT_3D('',#54358,#9645,#9646);
#8675=AXIS2_PLACEMENT_3D('',#54786,#9648,#9649);
#8676=AXIS2_PLACEMENT_3D('',#55202,#9651,#9652);
#8677=AXIS2_PLACEMENT_3D('',#55672,#9654,#9655);
#8678=AXIS2_PLACEMENT_3D('',#56094,#9657,#9658);
#8679=AXIS2_PLACEMENT_3D('',#56509,#9660,#9661);
#8680=AXIS2_PLACEMENT_3D('',#56932,#9663,#9664);
#8681=AXIS2_PLACEMENT_3D('',#57367,#9666,#9667);
#8682=AXIS2_PLACEMENT_3D('',#57792,#9669,#9670);
#8683=AXIS2_PLACEMENT_3D('',#57918,#9672,#9673);
#8684=AXIS2_PLACEMENT_3D('',#58084,#9674,#9675);
#8685=AXIS2_PLACEMENT_3D('',#58467,#9676,#9677);
#8686=AXIS2_PLACEMENT_3D('',#58498,#9678,#9679);
#8687=AXIS2_PLACEMENT_3D('',#59671,#9680,#9681);
#8688=AXIS2_PLACEMENT_3D('',#59672,#9682,#9683);
#8689=AXIS2_PLACEMENT_3D('',#59674,#9684,#9685);
#8690=AXIS2_PLACEMENT_3D('',#59677,#9687,#9688);
#8691=AXIS2_PLACEMENT_3D('',#59678,#9689,#9690);
#8692=AXIS2_PLACEMENT_3D('',#59679,#9691,#9692);
#9568=DIRECTION('axis',(0.,0.,1.));
#9569=DIRECTION('refdir',(1.,0.,0.));
#9570=DIRECTION('center_axis',(0.,0.,-1.));
#9571=DIRECTION('ref_axis',(-0.609351707504989,-0.792900054584911,0.));
#9572=DIRECTION('',(0.,0.,-1.));
#9573=DIRECTION('center_axis',(0.,0.,1.));
#9574=DIRECTION('ref_axis',(1.,-8.20798086521558E-14,0.));
#9575=DIRECTION('center_axis',(0.,0.,-1.));
#9576=DIRECTION('ref_axis',(-0.609351707504989,-0.792900054584911,0.));
#9577=DIRECTION('',(0.,0.,-1.));
#9578=DIRECTION('center_axis',(0.,0.,-1.));
#9579=DIRECTION('ref_axis',(-0.609351707504989,-0.792900054584911,0.));
#9580=DIRECTION('',(0.,0.,-1.));
#9581=DIRECTION('center_axis',(0.,0.,-1.));
#9582=DIRECTION('ref_axis',(-0.609351707504989,-0.792900054584911,0.));
#9583=DIRECTION('',(0.,0.,-1.));
#9584=DIRECTION('center_axis',(0.,0.,-1.));
#9585=DIRECTION('ref_axis',(-0.609351707504989,-0.792900054584911,0.));
#9586=DIRECTION('',(0.,0.,-1.));
#9587=DIRECTION('center_axis',(0.,0.,-1.));
#9588=DIRECTION('ref_axis',(-0.609351707504989,-0.792900054584911,0.));
#9589=DIRECTION('',(0.,0.,-1.));
#9590=DIRECTION('center_axis',(0.,0.,-1.));
#9591=DIRECTION('ref_axis',(-0.609351707504989,-0.792900054584911,0.));
#9592=DIRECTION('',(0.,0.,-1.));
#9593=DIRECTION('center_axis',(0.,0.,-1.));
#9594=DIRECTION('ref_axis',(-0.609351707504989,-0.792900054584911,0.));
#9595=DIRECTION('',(0.,0.,-1.));
#9596=DIRECTION('center_axis',(0.,0.,-1.));
#9597=DIRECTION('ref_axis',(-0.609351707504989,-0.792900054584911,0.));
#9598=DIRECTION('',(0.,0.,-1.));
#9599=DIRECTION('center_axis',(0.,0.,-1.));
#9600=DIRECTION('ref_axis',(-0.609351707504989,-0.792900054584911,0.));
#9601=DIRECTION('',(0.,0.,-1.));
#9602=DIRECTION('center_axis',(0.,0.,-1.));
#9603=DIRECTION('ref_axis',(-0.609351707504989,-0.792900054584911,0.));
#9604=DIRECTION('',(0.,0.,-1.));
#9605=DIRECTION('center_axis',(0.,0.,-1.));
#9606=DIRECTION('ref_axis',(-0.609351707504989,-0.792900054584911,0.));
#9607=DIRECTION('',(0.,0.,-1.));
#9608=DIRECTION('center_axis',(0.,0.,-1.));
#9609=DIRECTION('ref_axis',(-0.609351707504989,-0.792900054584911,0.));
#9610=DIRECTION('',(0.,0.,-1.));
#9611=DIRECTION('center_axis',(0.,0.,-1.));
#9612=DIRECTION('ref_axis',(-0.609351707504989,-0.792900054584911,0.));
#9613=DIRECTION('',(0.,0.,-1.));
#9614=DIRECTION('center_axis',(0.,0.,-1.));
#9615=DIRECTION('ref_axis',(-0.609351707504989,-0.792900054584911,0.));
#9616=DIRECTION('',(0.,0.,-1.));
#9617=DIRECTION('center_axis',(0.,0.,-1.));
#9618=DIRECTION('ref_axis',(-0.609351707504989,-0.792900054584911,0.));
#9619=DIRECTION('',(0.,0.,-1.));
#9620=DIRECTION('center_axis',(0.,0.,-1.));
#9621=DIRECTION('ref_axis',(1.,-8.20798086521558E-14,0.));
#9622=DIRECTION('center_axis',(0.,0.,-1.));
#9623=DIRECTION('ref_axis',(0.938434153860821,-0.345458157911382,0.));
#9624=DIRECTION('',(0.,0.,-1.));
#9625=DIRECTION('center_axis',(0.,0.,1.));
#9626=DIRECTION('ref_axis',(1.,0.,0.));
#9627=DIRECTION('',(0.,0.,-1.));
#9628=DIRECTION('center_axis',(0.,0.,1.));
#9629=DIRECTION('ref_axis',(1.,0.,0.));
#9630=DIRECTION('center_axis',(0.,0.,-1.));
#9631=DIRECTION('ref_axis',(0.938434153860821,-0.345458157911382,0.));
#9632=DIRECTION('',(0.,0.,-1.));
#9633=DIRECTION('center_axis',(0.,0.,-1.));
#9634=DIRECTION('ref_axis',(0.938434153860821,-0.345458157911382,0.));
#9635=DIRECTION('',(0.,0.,-1.));
#9636=DIRECTION('center_axis',(0.,0.,-1.));
#9637=DIRECTION('ref_axis',(0.938434153860821,-0.345458157911382,0.));
#9638=DIRECTION('',(0.,0.,-1.));
#9639=DIRECTION('center_axis',(0.,0.,-1.));
#9640=DIRECTION('ref_axis',(0.938434153860821,-0.345458157911382,0.));
#9641=DIRECTION('',(0.,0.,-1.));
#9642=DIRECTION('center_axis',(0.,0.,-1.));
#9643=DIRECTION('ref_axis',(0.938434153860821,-0.345458157911382,0.));
#9644=DIRECTION('',(0.,0.,-1.));
#9645=DIRECTION('center_axis',(0.,0.,-1.));
#9646=DIRECTION('ref_axis',(0.938434153860821,-0.345458157911382,0.));
#9647=DIRECTION('',(0.,0.,-1.));
#9648=DIRECTION('center_axis',(0.,0.,-1.));
#9649=DIRECTION('ref_axis',(0.938434153860821,-0.345458157911382,0.));
#9650=DIRECTION('',(0.,0.,-1.));
#9651=DIRECTION('center_axis',(0.,0.,-1.));
#9652=DIRECTION('ref_axis',(0.938434153860821,-0.345458157911382,0.));
#9653=DIRECTION('',(0.,0.,-1.));
#9654=DIRECTION('center_axis',(0.,0.,-1.));
#9655=DIRECTION('ref_axis',(0.938434153860821,-0.345458157911382,0.));
#9656=DIRECTION('',(0.,0.,-1.));
#9657=DIRECTION('center_axis',(0.,0.,-1.));
#9658=DIRECTION('ref_axis',(0.938434153860821,-0.345458157911382,0.));
#9659=DIRECTION('',(0.,0.,-1.));
#9660=DIRECTION('center_axis',(0.,0.,-1.));
#9661=DIRECTION('ref_axis',(0.938434153860821,-0.345458157911382,0.));
#9662=DIRECTION('',(0.,0.,-1.));
#9663=DIRECTION('center_axis',(0.,0.,-1.));
#9664=DIRECTION('ref_axis',(0.938434153860821,-0.345458157911382,0.));
#9665=DIRECTION('',(0.,0.,-1.));
#9666=DIRECTION('center_axis',(0.,0.,-1.));
#9667=DIRECTION('ref_axis',(0.938434153860821,-0.345458157911382,0.));
#9668=DIRECTION('',(0.,0.,-1.));
#9669=DIRECTION('center_axis',(0.,0.,-1.));
#9670=DIRECTION('ref_axis',(0.938434153860821,-0.345458157911382,0.));
#9671=DIRECTION('',(0.,0.,-1.));
#9672=DIRECTION('center_axis',(0.,0.,-1.));
#9673=DIRECTION('ref_axis',(1.,0.,0.));
#9674=DIRECTION('center_axis',(0.,0.,-1.));
#9675=DIRECTION('ref_axis',(0.938434153860821,-0.345458157911382,0.));
#9676=DIRECTION('center_axis',(0.,0.,-1.));
#9677=DIRECTION('ref_axis',(-0.609351707504989,-0.792900054584911,0.));
#9678=DIRECTION('center_axis',(0.,0.,1.));
#9679=DIRECTION('ref_axis',(1.,0.,0.));
#9680=DIRECTION('center_axis',(0.,0.,-1.));
#9681=DIRECTION('ref_axis',(1.,0.,0.));
#9682=DIRECTION('center_axis',(0.,0.,1.));
#9683=DIRECTION('ref_axis',(1.,0.,0.));
#9684=DIRECTION('center_axis',(0.,0.,1.));
#9685=DIRECTION('ref_axis',(1.,0.,0.));
#9686=DIRECTION('',(0.,0.,-1.));
#9687=DIRECTION('center_axis',(0.,0.,1.));
#9688=DIRECTION('ref_axis',(1.,0.,0.));
#9689=DIRECTION('center_axis',(0.,0.,1.));
#9690=DIRECTION('ref_axis',(1.,0.,0.));
#9691=DIRECTION('center_axis',(0.,0.,1.));
#9692=DIRECTION('ref_axis',(1.,0.,0.));
#48398=CARTESIAN_POINT('',(0.,0.,0.));
#48399=CARTESIAN_POINT('Origin',(0.,0.,18.5459252805377));
#48400=CARTESIAN_POINT('',(1.25206542099588,1.62921138715834,6.10605191404524));
#48401=CARTESIAN_POINT('',(1.24933779518059,1.62565558510666,6.04785047420624));
#48402=CARTESIAN_POINT('',(1.25206542099588,1.62921138715835,18.5459252805377));
#48403=CARTESIAN_POINT('',(1.81742788875953,0.958620587959108,6.));
#48404=CARTESIAN_POINT('Ctrl Pts',(1.24933779518059,1.62565558510666,6.04785047420624));
#48405=CARTESIAN_POINT('Ctrl Pts',(1.48318281877138,1.44625946904293,6.0319003161375));
#48406=CARTESIAN_POINT('Ctrl Pts',(1.68018382414042,1.21881862015088,6.01595015806875));
#48407=CARTESIAN_POINT('Ctrl Pts',(1.81742788875952,0.958620587959134,6.));
#48408=CARTESIAN_POINT('',(2.05337162055578,-0.0752499195754643,6.00000000147866));
#48409=CARTESIAN_POINT('Origin',(0.,0.,6.));
#48410=CARTESIAN_POINT('Ctrl Pts',(1.25206542099588,1.62921138715834,6.10605191404525));
#48411=CARTESIAN_POINT('Ctrl Pts',(1.30822134072944,1.58605499515372,6.10219269208269));
#48412=CARTESIAN_POINT('Ctrl Pts',(1.36224784768931,1.53991148578638,6.09833347012013));
#48413=CARTESIAN_POINT('Ctrl Pts',(1.4138096340505,1.49101974539776,6.09447424815757));
#48414=CARTESIAN_POINT('Ctrl Pts',(1.46640293060909,1.44114990994419,6.09053782121262));
#48415=CARTESIAN_POINT('Ctrl Pts',(1.5164313608693,1.38842093138857,6.08660139426767));
#48416=CARTESIAN_POINT('Ctrl Pts',(1.56357224503334,1.33313142527712,6.08266496732271));
#48417=CARTESIAN_POINT('Ctrl Pts',(1.6096779245744,1.27905606593749,6.0788149835458));
#48418=CARTESIAN_POINT('Ctrl Pts',(1.65302125352251,1.22253188410836,6.07496499976889));
#48419=CARTESIAN_POINT('Ctrl Pts',(1.69333715435579,1.1638757855451,6.07111501599197));
#48420=CARTESIAN_POINT('Ctrl Pts',(1.73363253838607,1.10524953713016,6.06726699147573));
#48421=CARTESIAN_POINT('Ctrl Pts',(1.77090327511889,1.04449392614358,6.06341896695949));
#48422=CARTESIAN_POINT('Ctrl Pts',(1.80492601849622,0.981957040941911,6.05957094244324));
#48423=CARTESIAN_POINT('Ctrl Pts',(1.83894295411342,0.919430830929606,6.05572357479358));
#48424=CARTESIAN_POINT('Ctrl Pts',(1.86971276468624,0.855124379387284,6.05187620714392));
#48425=CARTESIAN_POINT('Ctrl Pts',(1.89705760188735,0.789411184124871,6.04802883949426));
#48426=CARTESIAN_POINT('Ctrl Pts',(1.9255043408027,0.721049975931321,6.04402643632629));
#48427=CARTESIAN_POINT('Ctrl Pts',(1.95024395649681,0.651166749571664,6.04002403315833));
#48428=CARTESIAN_POINT('Ctrl Pts',(1.97113196590956,0.580203701702709,6.03602162999036));
#48429=CARTESIAN_POINT('Ctrl Pts',(1.99123710164174,0.51190031859027,6.03216923518544));
#48430=CARTESIAN_POINT('Ctrl Pts',(2.00777416259453,0.442597125760258,6.02831684038051));
#48431=CARTESIAN_POINT('Ctrl Pts',(2.02066619972994,0.372700512166221,6.02446444557559));
#48432=CARTESIAN_POINT('Ctrl Pts',(2.03356726706987,0.302754939613283,6.02060935236756));
#48433=CARTESIAN_POINT('Ctrl Pts',(2.04281816954012,0.232215602728014,6.01675425915953));
#48434=CARTESIAN_POINT('Ctrl Pts',(2.04839380242372,0.161494249718358,6.0128991659515));
#48435=CARTESIAN_POINT('Ctrl Pts',(2.05397836731133,0.090659603128962,6.00903789699469));
#48436=CARTESIAN_POINT('Ctrl Pts',(2.05587591160232,0.0196428450353519,
6.00517662803788));
#48437=CARTESIAN_POINT('Ctrl Pts',(2.05411337054193,-0.0511451215746277,
6.00131535908107));
#48438=CARTESIAN_POINT('Ctrl Pts',(2.05391323151947,-0.0591831949887535,
6.00087690654694));
#48439=CARTESIAN_POINT('Ctrl Pts',(2.05366595440477,-0.0672183259752531,
6.0004384540128));
#48440=CARTESIAN_POINT('Ctrl Pts',(2.05337162055578,-0.0752499195754648,
6.00000000147866));
#48441=CARTESIAN_POINT('Origin',(0.,0.,18.5459252805377));
#48442=CARTESIAN_POINT('',(1.25156703223363,1.62854649222322,6.80617425834606));
#48443=CARTESIAN_POINT('',(1.25206542099589,1.62921138715833,6.74786344002215));
#48444=CARTESIAN_POINT('',(1.25206542099588,1.62921138715835,18.5459252805377));
#48445=CARTESIAN_POINT('',(-2.05462925654524,-0.0015224618017469,6.29592530139563));
#48446=CARTESIAN_POINT('Ctrl Pts',(1.25206542099589,1.62921138715833,6.74786344002215));
#48447=CARTESIAN_POINT('Ctrl Pts',(1.30854725833057,1.58580452418249,6.74400537831042));
#48448=CARTESIAN_POINT('Ctrl Pts',(1.36281932984893,1.53941850059499,6.7401473165987));
#48449=CARTESIAN_POINT('Ctrl Pts',(1.41455660915229,1.49031109571243,6.73628925488698));
#48450=CARTESIAN_POINT('Ctrl Pts',(1.46627146229503,1.44122497703904,6.7324328654996));
#48451=CARTESIAN_POINT('Ctrl Pts',(1.515453352015,1.38942015202907,6.72857647611223));
#48452=CARTESIAN_POINT('Ctrl Pts',(1.56181186435802,1.3351933428723,6.72472008672485));
#48453=CARTESIAN_POINT('Ctrl Pts',(1.60816577128011,1.28097192080131,6.72086408044503));
#48454=CARTESIAN_POINT('Ctrl Pts',(1.65169654324184,1.22432936221296,6.71700807416521));
#48455=CARTESIAN_POINT('Ctrl Pts',(1.69215320353844,1.16559645600636,6.71315206788539));
#48456=CARTESIAN_POINT('Ctrl Pts',(1.73268093267178,1.10676037570454,6.70928928789072));
#48457=CARTESIAN_POINT('Ctrl Pts',(1.77012346576075,1.04582700106825,6.70542650789604));
#48458=CARTESIAN_POINT('Ctrl Pts',(1.8042724723433,0.983157366876838,6.70156372790137));
#48459=CARTESIAN_POINT('Ctrl Pts',(1.83840916765922,0.920510326097459,6.69770234050107));
#48460=CARTESIAN_POINT('Ctrl Pts',(1.86925451742048,0.856128725321618,6.69384095310078));
#48461=CARTESIAN_POINT('Ctrl Pts',(1.89664781037034,0.790395246643986,6.68997956570048));
#48462=CARTESIAN_POINT('Ctrl Pts',(1.92409242387181,0.724538618172293,6.68611094410122));
#48463=CARTESIAN_POINT('Ctrl Pts',(1.94807189147438,0.657325508925034,6.68224232250196));
#48464=CARTESIAN_POINT('Ctrl Pts',(1.96847472927211,0.589156008810146,6.6783737009027));
#48465=CARTESIAN_POINT('Ctrl Pts',(1.98882329509229,0.521167840998941,6.67451536991824));
#48466=CARTESIAN_POINT('Ctrl Pts',(2.00561420302378,0.452228846973817,6.67065703893378));
#48467=CARTESIAN_POINT('Ctrl Pts',(2.01878791325744,0.382743940233756,6.66679870794932));
#48468=CARTESIAN_POINT('Ctrl Pts',(2.0320020065519,0.313046032511898,6.66292854952885));
#48469=CARTESIAN_POINT('Ctrl Pts',(2.04162817079777,0.242527197504543,6.65905839110839));
#48470=CARTESIAN_POINT('Ctrl Pts',(2.04757284006439,0.171589705782855,6.65518823268792));
#48471=CARTESIAN_POINT('Ctrl Pts',(2.05350867604944,0.100757621243658,6.65132382499933));
#48472=CARTESIAN_POINT('Ctrl Pts',(2.05577383564748,0.0295085947020155,
6.64745941731074));
#48473=CARTESIAN_POINT('Ctrl Pts',(2.05432589106127,-0.0417456083355204,
6.64359500962215));
#48474=CARTESIAN_POINT('Ctrl Pts',(2.05287963868512,-0.112916536723224,
6.63973511825939));
#48475=CARTESIAN_POINT('Ctrl Pts',(2.04772891178417,-0.18409214656408,6.63587522689661));
#48476=CARTESIAN_POINT('Ctrl Pts',(2.03888326303558,-0.25485800402063,6.63201533553385));
#48477=CARTESIAN_POINT('Ctrl Pts',(2.03004316454245,-0.325579459014725,
6.62815786608311));
#48478=CARTESIAN_POINT('Ctrl Pts',(2.01751280404875,-0.395891191136253,
6.62430039663237));
#48479=CARTESIAN_POINT('Ctrl Pts',(2.00135366856377,-0.465382698245589,
6.62044292718163));
#48480=CARTESIAN_POINT('Ctrl Pts',(1.98519927542666,-0.534853811138811,
6.61658658981262));
#48481=CARTESIAN_POINT('Ctrl Pts',(1.96541833149422,-0.603504704330993,
6.61273025244361));
#48482=CARTESIAN_POINT('Ctrl Pts',(1.94212331801147,-0.670935600587797,
6.6088739150746));
#48483=CARTESIAN_POINT('Ctrl Pts',(1.91882736130922,-0.738369227134346,
6.60501742156176));
#48484=CARTESIAN_POINT('Ctrl Pts',(1.89201721316103,-0.804582300537594,
6.60116092804892));
#48485=CARTESIAN_POINT('Ctrl Pts',(1.86185450043045,-0.869192373256286,
6.59730443453608));
#48486=CARTESIAN_POINT('Ctrl Pts',(1.83166022187499,-0.933870061585644,
6.59344390513297));
#48487=CARTESIAN_POINT('Ctrl Pts',(1.79810658072365,-0.996940959639327,
6.58958337572986));
#48488=CARTESIAN_POINT('Ctrl Pts',(1.76140206117851,-1.05804552897127,6.58572284632675));
#48489=CARTESIAN_POINT('Ctrl Pts',(1.72467674727163,-1.11918471612506,6.58186012980211));
#48490=CARTESIAN_POINT('Ctrl Pts',(1.68479727279809,-1.17835495413582,6.57799741327746));
#48491=CARTESIAN_POINT('Ctrl Pts',(1.64201500142225,-1.23522641552239,6.57413469675282));
#48492=CARTESIAN_POINT('Ctrl Pts',(1.599158006467,-1.29219720868879,6.5702652336017));
#48493=CARTESIAN_POINT('Ctrl Pts',(1.5533884038574,-1.34686083670187,6.56639577045058));
#48494=CARTESIAN_POINT('Ctrl Pts',(1.5049968323029,-1.39892176237924,6.56252630729946));
#48495=CARTESIAN_POINT('Ctrl Pts',(1.47639674996706,-1.42969048331602,6.56023940151892));
#48496=CARTESIAN_POINT('Ctrl Pts',(1.4468815172348,-1.45955079845428,6.55795249573838));
#48497=CARTESIAN_POINT('Ctrl Pts',(1.41651657404932,-1.48844830543206,6.55566558995783));
#48498=CARTESIAN_POINT('Ctrl Pts',(1.36521646640748,-1.53726925034495,6.55180197289153));
#48499=CARTESIAN_POINT('Ctrl Pts',(1.31128724265687,-1.58353219853699,6.54793835582523));
#48500=CARTESIAN_POINT('Ctrl Pts',(1.255014660813,-1.62694061466435,6.54407473875893));
#48501=CARTESIAN_POINT('Ctrl Pts',(1.19882623299308,-1.67028411475675,6.54021689962058));
#48502=CARTESIAN_POINT('Ctrl Pts',(1.14030178525658,-1.71078126046051,6.53635906048222));
#48503=CARTESIAN_POINT('Ctrl Pts',(1.07976287558482,-1.74817324513584,6.53250122134386));
#48504=CARTESIAN_POINT('Ctrl Pts',(1.01929498024369,-1.78552136766076,6.52864790759035));
#48505=CARTESIAN_POINT('Ctrl Pts',(0.956817728828559,-1.81977130880502,
6.52479459383683));
#48506=CARTESIAN_POINT('Ctrl Pts',(0.892683194147317,-1.85070642658066,
6.52094128008331));
#48507=CARTESIAN_POINT('Ctrl Pts',(0.828589006849113,-1.8816220829062,6.51709039047034));
#48508=CARTESIAN_POINT('Ctrl Pts',(0.762840042435076,-1.90922684157126,
6.51323950085737));
#48509=CARTESIAN_POINT('Ctrl Pts',(0.695813303091591,-1.93334978980545,
6.5093886112444));
#48510=CARTESIAN_POINT('Ctrl Pts',(0.628806142268257,-1.957465691723,6.50553884647684));
#48511=CARTESIAN_POINT('Ctrl Pts',(0.5605224056806,-1.97810163717773,6.50168908170928));
#48512=CARTESIAN_POINT('Ctrl Pts',(0.491357788836919,-1.99513535527024,
6.49783931694172));
#48513=CARTESIAN_POINT('Ctrl Pts',(0.422190066630577,-2.012169838145,6.49398937932688));
#48514=CARTESIAN_POINT('Ctrl Pts',(0.352141859343161,-2.02560165820165,
6.49013944171204));
#48515=CARTESIAN_POINT('Ctrl Pts',(0.281620981923863,-2.0353592275174,6.4862895040972));
#48516=CARTESIAN_POINT('Ctrl Pts',(0.211024891169831,-2.04512720367087,
6.48243546036999));
#48517=CARTESIAN_POINT('Ctrl Pts',(0.139955607671059,-2.05121303969876,
6.47858141664279));
#48518=CARTESIAN_POINT('Ctrl Pts',(0.068827126234984,-2.05359693932238,
6.47472737291559));
#48519=CARTESIAN_POINT('Ctrl Pts',(-0.00234226611308243,-2.05598221009164,
6.47087111246113));
#48520=CARTESIAN_POINT('Ctrl Pts',(-0.0735704367650953,-2.05466131556808,
6.46701485200667));
#48521=CARTESIAN_POINT('Ctrl Pts',(-0.144445123139336,-2.04966659945008,
6.4631585915522));
#48522=CARTESIAN_POINT('Ctrl Pts',(-0.21544595536584,-2.0446629935189,6.45929546755751));
#48523=CARTESIAN_POINT('Ctrl Pts',(-0.286091563497953,-2.03597257107392,
6.45543234356281));
#48524=CARTESIAN_POINT('Ctrl Pts',(-0.355977220656732,-2.02367926828179,
6.45156921956811));
#48525=CARTESIAN_POINT('Ctrl Pts',(-0.398409867662541,-2.01621511327314,
6.44922363703414));
#48526=CARTESIAN_POINT('Ctrl Pts',(-0.440562574257773,-2.00742372133879,
6.44687805450017));
#48527=CARTESIAN_POINT('Ctrl Pts',(-0.482347616612758,-1.99733280633148,
6.4445324719662));
#48528=CARTESIAN_POINT('Ctrl Pts',(-0.551405647416069,-1.98065557734873,
6.44065593381395));
#48529=CARTESIAN_POINT('Ctrl Pts',(-0.61973077906983,-1.96036049456912,
6.4367793956617));
#48530=CARTESIAN_POINT('Ctrl Pts',(-0.686916947322909,-1.93652850998393,
6.43290285750945));
#48531=CARTESIAN_POINT('Ctrl Pts',(-0.754002799907351,-1.91273210893521,
6.42903210741636));
#48532=CARTESIAN_POINT('Ctrl Pts',(-0.819952612775803,-1.88540945021994,
6.42516135732327));
#48533=CARTESIAN_POINT('Ctrl Pts',(-0.884372772943357,-1.85469198547265,
6.42129060723018));
#48534=CARTESIAN_POINT('Ctrl Pts',(-0.948716347889046,-1.82401103885643,
6.41742445883715));
#48535=CARTESIAN_POINT('Ctrl Pts',(-1.01153344826937,-1.78994351123954,
6.41355831044411));
#48536=CARTESIAN_POINT('Ctrl Pts',(-1.07244946898083,-1.75266930679542,
6.40969216205108));
#48537=CARTESIAN_POINT('Ctrl Pts',(-1.13332644277837,-1.71541899496009,
6.40582849184296));
#48538=CARTESIAN_POINT('Ctrl Pts',(-1.19230434322614,-1.67496633677039,
6.40196482163484));
#48539=CARTESIAN_POINT('Ctrl Pts',(-1.24903353557167,-1.63153694089878,
6.39810115142672));
#48540=CARTESIAN_POINT('Ctrl Pts',(-1.30574514939581,-1.58812100237659,
6.39423867844363));
#48541=CARTESIAN_POINT('Ctrl Pts',(-1.36020905472129,-1.54173045150558,
6.39037620546055));
#48542=CARTESIAN_POINT('Ctrl Pts',(-1.41210637222193,-1.49263296092181,
6.38651373247746));
#48543=CARTESIAN_POINT('Ctrl Pts',(-1.46400479239372,-1.4435344271553,6.38265117742776));
#48544=CARTESIAN_POINT('Ctrl Pts',(-1.51333616654172,-1.39172917353487,
6.37878862237805));
#48545=CARTESIAN_POINT('Ctrl Pts',(-1.55981761405094,-1.3375225506123,6.37492606732835));
#48546=CARTESIAN_POINT('Ctrl Pts',(-1.6063457778695,-1.28326144717115,6.37105963020684));
#48547=CARTESIAN_POINT('Ctrl Pts',(-1.65001798132448,-1.22659452423105,
6.36719319308534));
#48548=CARTESIAN_POINT('Ctrl Pts',(-1.6905914870465,-1.16786043105583,6.36332675596384));
#48549=CARTESIAN_POINT('Ctrl Pts',(-1.73118712286992,-1.10909430240785,
6.35945820996256));
#48550=CARTESIAN_POINT('Ctrl Pts',(-1.76868044147491,-1.04825917046698,
6.35558966396129));
#48551=CARTESIAN_POINT('Ctrl Pts',(-1.80287338849916,-0.985720603184072,
6.35172111796001));
#48552=CARTESIAN_POINT('Ctrl Pts',(-1.83712432758889,-0.923075968977871,
6.34784601081111));
#48553=CARTESIAN_POINT('Ctrl Pts',(-1.86806350901278,-0.858722567140702,
6.34397090366222));
#48554=CARTESIAN_POINT('Ctrl Pts',(-1.8955402628438,-0.793047712586098,
6.34009579651332));
#48555=CARTESIAN_POINT('Ctrl Pts',(-1.91136748138743,-0.755217542317477,
6.33786364900045));
#48556=CARTESIAN_POINT('Ctrl Pts',(-1.92604677240116,-0.71694924401247,
6.33563150148759));
#48557=CARTESIAN_POINT('Ctrl Pts',(-1.93955690842656,-0.67831892312895,
6.33339935397472));
#48558=CARTESIAN_POINT('Ctrl Pts',(-1.96671951453605,-0.600651297276029,
6.3289115424859));
#48559=CARTESIAN_POINT('Ctrl Pts',(-1.98923851869651,-0.521277422665017,
6.32442373099708));
#48560=CARTESIAN_POINT('Ctrl Pts',(-2.00692889343075,-0.440719842091111,
6.31993591950826));
#48561=CARTESIAN_POINT('Ctrl Pts',(-2.02446373253168,-0.360870532229469,
6.31548756532957));
#48562=CARTESIAN_POINT('Ctrl Pts',(-2.03725438909028,-0.279858398211875,
6.31103921115088));
#48563=CARTESIAN_POINT('Ctrl Pts',(-2.04516728440973,-0.198212868603796,
6.30659085697219));
#48564=CARTESIAN_POINT('Ctrl Pts',(-2.05149137716537,-0.132960659206291,
6.30303567226416));
#48565=CARTESIAN_POINT('Ctrl Pts',(-2.05470069136051,-0.0673042961116859,
6.29948048755612));
#48566=CARTESIAN_POINT('Ctrl Pts',(-2.05474943588193,-0.00152257770586607,
6.29592530284809));
#48567=CARTESIAN_POINT('Ctrl Pts',(-2.05290342576851,-0.00152079736506813,
6.29592528053768));
#48568=CARTESIAN_POINT('Ctrl Pts',(-2.04996245021167,0.452378852210551,
6.27137226568616));
#48569=CARTESIAN_POINT('Ctrl Pts',(-1.67847430924827,1.59588320600937,6.20977487817079));
#48570=CARTESIAN_POINT('Ctrl Pts',(-0.0899020486618461,2.28520748800009,
6.1270832760603));
#48571=CARTESIAN_POINT('Ctrl Pts',(0.940075837502264,1.86290841692593,6.06894468880133));
#48572=CARTESIAN_POINT('Ctrl Pts',(1.24933779518059,1.62565558510666,6.04785047420624));
#48573=CARTESIAN_POINT('',(-2.05474920289297,0.00180989245198827,6.35407471946232));
#48574=CARTESIAN_POINT('Ctrl Pts',(-2.05474920289297,0.00180989245198827,
6.35407471946232));
#48575=CARTESIAN_POINT('Ctrl Pts',(-2.05466014208798,0.102919556662241,
6.34858528835285));
#48576=CARTESIAN_POINT('Ctrl Pts',(-2.04710452302201,0.203708660391641,
6.34309585724339));
#48577=CARTESIAN_POINT('Ctrl Pts',(-2.03224380207686,0.303286484071088,
6.33760642613394));
#48578=CARTESIAN_POINT('Ctrl Pts',(-2.02648140179202,0.341898828764958,
6.33547784169275));
#48579=CARTESIAN_POINT('Ctrl Pts',(-2.01962109224582,0.380329380421406,
6.33334925725156));
#48580=CARTESIAN_POINT('Ctrl Pts',(-2.01167405834273,0.418527233870032,
6.33122067281038));
#48581=CARTESIAN_POINT('Ctrl Pts',(-1.99724932624694,0.487860498248844,
6.32735706021204));
#48582=CARTESIAN_POINT('Ctrl Pts',(-1.97920723753694,0.55658526441417,6.3234934476137));
#48583=CARTESIAN_POINT('Ctrl Pts',(-1.95761415720994,0.624295101687676,
6.31962983501537));
#48584=CARTESIAN_POINT('Ctrl Pts',(-1.93605336879913,0.691903680578496,
6.31577200035387));
#48585=CARTESIAN_POINT('Ctrl Pts',(-1.91095227567684,0.758499882712945,
6.31191416569237));
#48586=CARTESIAN_POINT('Ctrl Pts',(-1.8824281473951,0.823687946005434,6.30805633103088));
#48587=CARTESIAN_POINT('Ctrl Pts',(-1.85393747893297,0.888799541375144,
6.304203021747));
#48588=CARTESIAN_POINT('Ctrl Pts',(-1.82203194472304,0.952505834385205,
6.30034971246313));
#48589=CARTESIAN_POINT('Ctrl Pts',(-1.78687789504914,1.01442838617851,6.29649640317925));
#48590=CARTESIAN_POINT('Ctrl Pts',(-1.7517459609449,1.07631198221794,6.29264551802946));
#48591=CARTESIAN_POINT('Ctrl Pts',(-1.71336980552832,1.13641364039341,6.28879463287967));
#48592=CARTESIAN_POINT('Ctrl Pts',(-1.67196229335458,1.19437835383119,6.28494374772987));
#48593=CARTESIAN_POINT('Ctrl Pts',(-1.63056687620076,1.2523261359363,6.28109398741299));
#48594=CARTESIAN_POINT('Ctrl Pts',(-1.5861421430789,1.3081378160752,6.27724422709611));
#48595=CARTESIAN_POINT('Ctrl Pts',(-1.53894400043637,1.36148776197985,6.27339446677923));
#48596=CARTESIAN_POINT('Ctrl Pts',(-1.49174373845498,1.41484010345786,6.26954453359651));
#48597=CARTESIAN_POINT('Ctrl Pts',(-1.44177014427008,1.46573012775092,6.26569460041379));
#48598=CARTESIAN_POINT('Ctrl Pts',(-1.38931792025673,1.51386699513316,6.26184466723107));
#48599=CARTESIAN_POINT('Ctrl Pts',(-1.33680975299792,1.56205520319043,6.25799062787819));
#48600=CARTESIAN_POINT('Ctrl Pts',(-1.28181803861058,1.60748406262357,6.25413658852532));
#48601=CARTESIAN_POINT('Ctrl Pts',(-1.22467202077841,1.64990181647955,6.25028254917244));
#48602=CARTESIAN_POINT('Ctrl Pts',(-1.16749313389932,1.69234396803103,6.24642629306667));
#48603=CARTESIAN_POINT('Ctrl Pts',(-1.10815788334922,1.73177129709322,6.24257003696089));
#48604=CARTESIAN_POINT('Ctrl Pts',(-1.04702374466157,1.76797591629945,6.23871378085512));
#48605=CARTESIAN_POINT('Ctrl Pts',(-0.985780795263479,1.80424497495672,
6.23485066112167));
#48606=CARTESIAN_POINT('Ctrl Pts',(-0.922732997265713,1.83727964592423,
6.23098754138821));
#48607=CARTESIAN_POINT('Ctrl Pts',(-0.858260973366345,1.86691876205052,
6.22712442165476));
#48608=CARTESIAN_POINT('Ctrl Pts',(-0.819114628949602,1.88491514215329,
6.2247787993761));
#48609=CARTESIAN_POINT('Ctrl Pts',(-0.779443596283827,1.90166062200296,
6.22243317709744));
#48610=CARTESIAN_POINT('Ctrl Pts',(-0.739335794758498,1.91712809824717,
6.22008755481877));
#48611=CARTESIAN_POINT('Ctrl Pts',(-0.673050825505878,1.94269073564617,
6.21621101472666));
#48612=CARTESIAN_POINT('Ctrl Pts',(-0.605310861272263,1.96486087863528,
6.21233447463455));
#48613=CARTESIAN_POINT('Ctrl Pts',(-0.536495928273019,1.98347414438567,
6.20845793454244));
#48614=CARTESIAN_POINT('Ctrl Pts',(-0.467783743147285,2.00205961858862,
6.20458718252907));
#48615=CARTESIAN_POINT('Ctrl Pts',(-0.398000238841365,2.01709863318447,
6.2007164305157));
#48616=CARTESIAN_POINT('Ctrl Pts',(-0.327543924189893,2.02847542263304,
6.19684567850233));
#48617=CARTESIAN_POINT('Ctrl Pts',(-0.257171371421285,2.03983868680272,
6.19297952822663));
#48618=CARTESIAN_POINT('Ctrl Pts',(-0.186128072653157,2.04754829854207,
6.18911337795092));
#48619=CARTESIAN_POINT('Ctrl Pts',(-0.114824462259788,2.0515391552117,6.18524722767522));
#48620=CARTESIAN_POINT('Ctrl Pts',(-0.0435665576071448,2.05552745373514,
6.1813835556087));
#48621=CARTESIAN_POINT('Ctrl Pts',(0.0279508457125155,2.05580170015229,
6.17751988354218));
#48622=CARTESIAN_POINT('Ctrl Pts',(0.0993118548629316,2.05234858588488,
6.17365621147566));
#48623=CARTESIAN_POINT('Ctrl Pts',(0.17065075108685,2.04889654164805,6.16979373666093));
#48624=CARTESIAN_POINT('Ctrl Pts',(0.241832866438303,2.04171945339401,6.16593126184621));
#48625=CARTESIAN_POINT('Ctrl Pts',(0.312443678438297,2.03085610280589,6.16206878703149));
#48626=CARTESIAN_POINT('Ctrl Pts',(0.383055990182576,2.01999252148473,6.1582062301794));
#48627=CARTESIAN_POINT('Ctrl Pts',(0.453096496670009,2.00544259809723,6.15434367332732));
#48628=CARTESIAN_POINT('Ctrl Pts',(0.522158853022968,1.98729657945404,6.15048111647524));
#48629=CARTESIAN_POINT('Ctrl Pts',(0.591290619653305,1.96913232337654,6.14661467760759));
#48630=CARTESIAN_POINT('Ctrl Pts',(0.659441804753107,1.9473648800184,6.14274823873994));
#48631=CARTESIAN_POINT('Ctrl Pts',(0.726220140700263,1.92213471685553,6.13888179987229));
#48632=CARTESIAN_POINT('Ctrl Pts',(0.793034899188124,1.89689079254346,6.13501325215414));
#48633=CARTESIAN_POINT('Ctrl Pts',(0.858474874195766,1.86818058209607,6.131144704436));
#48634=CARTESIAN_POINT('Ctrl Pts',(0.922169238106877,1.83619210835614,6.12727615671785));
#48635=CARTESIAN_POINT('Ctrl Pts',(0.985971628101802,1.80414938194246,6.12340104791589));
#48636=CARTESIAN_POINT('Ctrl Pts',(1.04802207512344,1.76881753034704,6.11952593911392));
#48637=CARTESIAN_POINT('Ctrl Pts',(1.1079763550629,1.73042941466028,6.11565083031196));
#48638=CARTESIAN_POINT('Ctrl Pts',(1.14251107998624,1.70831718152353,6.11341869915037));
#48639=CARTESIAN_POINT('Ctrl Pts',(1.17635086489013,1.68519168236722,6.11118656798877));
#48640=CARTESIAN_POINT('Ctrl Pts',(1.20943496396806,1.66110343760754,6.10895443682718));
#48641=CARTESIAN_POINT('Ctrl Pts',(1.22377512356468,1.65066249214178,6.1079869292332));
#48642=CARTESIAN_POINT('Ctrl Pts',(1.23798712249006,1.64003070187989,6.10701942163922));
#48643=CARTESIAN_POINT('Ctrl Pts',(1.25206542099588,1.62921138715834,6.10605191404525));
#48644=CARTESIAN_POINT('Ctrl Pts',(1.2515670322334,1.6285464922234,6.80617425834608));
#48645=CARTESIAN_POINT('Ctrl Pts',(1.40105728510831,1.51592380612735,6.79603388715624));
#48646=CARTESIAN_POINT('Ctrl Pts',(2.02408552329212,0.900327067227945,6.74884914330253));
#48647=CARTESIAN_POINT('Ctrl Pts',(2.27789949074807,-0.842191245823211,
6.664620026785));
#48648=CARTESIAN_POINT('Ctrl Pts',(0.527846155910302,-2.37052290404747,
6.55348690879344));
#48649=CARTESIAN_POINT('Ctrl Pts',(-1.55202449963455,-1.7731560393209,6.4499719160968));
#48650=CARTESIAN_POINT('Ctrl Pts',(-2.05038434453856,-0.540370480513924,
6.383501296064));
#48651=CARTESIAN_POINT('Ctrl Pts',(-2.05538931506001,0.00180439026243735,
6.35407504869506));
#48652=CARTESIAN_POINT('Origin',(0.,0.,18.5459252805377));
#48653=CARTESIAN_POINT('',(1.25017377660034,1.6267706489614,7.50603355970618));
#48654=CARTESIAN_POINT('',(1.25206542099588,1.62921138715835,7.44794391597819));
#48655=CARTESIAN_POINT('',(1.25206542099588,1.62921138715835,18.5459252805377));
#48656=CARTESIAN_POINT('',(-2.05474994334797,-0.000482505435243929,6.99592528050785));
#48657=CARTESIAN_POINT('Ctrl Pts',(1.25206542099588,1.62921138715835,7.44794391597819));
#48658=CARTESIAN_POINT('Ctrl Pts',(1.26764871117023,1.61723547112532,7.44687278861555));
#48659=CARTESIAN_POINT('Ctrl Pts',(1.28305223476815,1.60504204850324,7.44580166125291));
#48660=CARTESIAN_POINT('Ctrl Pts',(1.29826972672408,1.59263720889969,7.44473053389027));
#48661=CARTESIAN_POINT('Ctrl Pts',(1.35323787633299,1.54782883435431,7.44086144105353));
#48662=CARTESIAN_POINT('Ctrl Pts',(1.40599119458351,1.50008360802498,7.43699234821679));
#48663=CARTESIAN_POINT('Ctrl Pts',(1.45619913804349,1.44964879638532,7.43312325538005));
#48664=CARTESIAN_POINT('Ctrl Pts',(1.50633227283071,1.39928913144674,7.42925992740201));
#48665=CARTESIAN_POINT('Ctrl Pts',(1.55392722100258,1.34624817728394,7.42539659942398));
#48666=CARTESIAN_POINT('Ctrl Pts',(1.59868643162176,1.29081340861044,7.42153327144594));
#48667=CARTESIAN_POINT('Ctrl Pts',(1.64339313728927,1.23544366789005,7.41767447535857));
#48668=CARTESIAN_POINT('Ctrl Pts',(1.68527040921453,1.17768606656781,7.41381567927119));
#48669=CARTESIAN_POINT('Ctrl Pts',(1.724058735042,1.11786360555543,7.40995688318382));
#48670=CARTESIAN_POINT('Ctrl Pts',(1.76282262571665,1.05807883039171,7.40610051798951));
#48671=CARTESIAN_POINT('Ctrl Pts',(1.79850116730473,0.996232182905278,7.4022441527952));
#48672=CARTESIAN_POINT('Ctrl Pts',(1.83087710417188,0.932677110215103,7.39838778760088));
#48673=CARTESIAN_POINT('Ctrl Pts',(1.86324347560073,0.869140814807854,7.39453256176583));
#48674=CARTESIAN_POINT('Ctrl Pts',(1.89230895906421,0.803897528887979,7.39067733593077));
#48675=CARTESIAN_POINT('Ctrl Pts',(1.91790221462563,0.737325340425854,7.38682211009571));
#48676=CARTESIAN_POINT('Ctrl Pts',(1.94349646970277,0.670750552062018,7.38296673369916));
#48677=CARTESIAN_POINT('Ctrl Pts',(1.96561805539294,0.602847212335397,7.37911135730261));
#48678=CARTESIAN_POINT('Ctrl Pts',(1.98414438906916,0.534011803076818,7.37525598090605));
#48679=CARTESIAN_POINT('Ctrl Pts',(2.002690113212,0.465104347684967,7.37139656930488));
#48680=CARTESIAN_POINT('Ctrl Pts',(2.01763294714544,0.395263345404606,7.3675371577037));
#48681=CARTESIAN_POINT('Ctrl Pts',(2.02890090929962,0.324897926652613,7.36367774610253));
#48682=CARTESIAN_POINT('Ctrl Pts',(2.04017525097089,0.254492669517639,7.35981614944056));
#48683=CARTESIAN_POINT('Ctrl Pts',(2.04777052731898,0.183562888110837,7.35595455277859));
#48684=CARTESIAN_POINT('Ctrl Pts',(2.05166669540355,0.112522590940064,7.35209295611663));
#48685=CARTESIAN_POINT('Ctrl Pts',(2.05556967960491,0.0413580129498467,
7.34822460381854));
#48686=CARTESIAN_POINT('Ctrl Pts',(2.05576063396187,-0.0299169808821453,
7.34435625152046));
#48687=CARTESIAN_POINT('Ctrl Pts',(2.05227164517212,-0.10088933007269,7.34048789922238));
#48688=CARTESIAN_POINT('Ctrl Pts',(2.05020006385277,-0.143029044939606,
7.33819107144783));
#48689=CARTESIAN_POINT('Ctrl Pts',(2.04683216072677,-0.185062161817784,
7.33589424367327));
#48690=CARTESIAN_POINT('Ctrl Pts',(2.04218320150506,-0.226903798977777,
7.33359741589872));
#48691=CARTESIAN_POINT('Ctrl Pts',(2.03435179900029,-0.297388113085845,
7.32972829553675));
#48692=CARTESIAN_POINT('Ctrl Pts',(2.02285171200631,-0.367604541133105,
7.32585917517479));
#48693=CARTESIAN_POINT('Ctrl Pts',(2.00771140280094,-0.437141264996901,
7.32199005481283));
#48694=CARTESIAN_POINT('Ctrl Pts',(1.99259365061969,-0.506574388495813,
7.31812669891975));
#48695=CARTESIAN_POINT('Ctrl Pts',(1.97384654412021,-0.575329347144338,
7.31426334302667));
#48696=CARTESIAN_POINT('Ctrl Pts',(1.95155022025858,-0.643000233521494,
7.31039998713359));
#48697=CARTESIAN_POINT('Ctrl Pts',(1.92928004845726,-0.710591746585247,
7.30654116269229));
#48698=CARTESIAN_POINT('Ctrl Pts',(1.90346907968105,-0.777101253957358,
7.30268233825098));
#48699=CARTESIAN_POINT('Ctrl Pts',(1.87424792885537,-0.84213553759556,7.29882351380968));
#48700=CARTESIAN_POINT('Ctrl Pts',(1.84504518416558,-0.907128856732772,
7.29496712000663));
#48701=CARTESIAN_POINT('Ctrl Pts',(1.81243671773462,-0.970648353663312,
7.29111072620358));
#48702=CARTESIAN_POINT('Ctrl Pts',(1.77660164236917,-1.03231979872091,7.28725433240053));
#48703=CARTESIAN_POINT('Ctrl Pts',(1.74077715240483,-1.09397302651577,7.28339907774606));
#48704=CARTESIAN_POINT('Ctrl Pts',(1.70172818962766,-1.15377886641638,7.27954382309159));
#48705=CARTESIAN_POINT('Ctrl Pts',(1.65967947199295,-1.21138829973928,7.27568856843712));
#48706=CARTESIAN_POINT('Ctrl Pts',(1.61762911038624,-1.26899998540898,7.27183316305438));
#48707=CARTESIAN_POINT('Ctrl Pts',(1.57257904924475,-1.32441470293893,7.26797775767164));
#48708=CARTESIAN_POINT('Ctrl Pts',(1.52479590461656,-1.37731442008155,7.26412235228889));
#48709=CARTESIAN_POINT('Ctrl Pts',(1.47696274781209,-1.4302695046555,7.2602629116503));
#48710=CARTESIAN_POINT('Ctrl Pts',(1.42639112344778,-1.48070397291409,7.25640347101171));
#48711=CARTESIAN_POINT('Ctrl Pts',(1.37338571891157,-1.52833544406643,7.25254403037312));
#48712=CARTESIAN_POINT('Ctrl Pts',(1.32035030384078,-1.57599388314639,7.24868240460119));
#48713=CARTESIAN_POINT('Ctrl Pts',(1.26487874343397,-1.62084586032309,7.24482077882926));
#48714=CARTESIAN_POINT('Ctrl Pts',(1.20730799371582,-1.6626499844555,7.24095915305733));
#48715=CARTESIAN_POINT('Ctrl Pts',(1.14963653116646,-1.70452723967824,7.23709077185375));
#48716=CARTESIAN_POINT('Ctrl Pts',(1.08985895505129,-1.74334573204196,7.23322239065017));
#48717=CARTESIAN_POINT('Ctrl Pts',(1.02833969894506,-1.77890838046078,7.2293540094466));
#48718=CARTESIAN_POINT('Ctrl Pts',(0.991817106643526,-1.80002112127676,
7.22705743893343));
#48719=CARTESIAN_POINT('Ctrl Pts',(0.954681113454435,-1.81998721792624,
7.22476086842027));
#48720=CARTESIAN_POINT('Ctrl Pts',(0.917011283475248,-1.83877346850532,
7.22246429790711));
#48721=CARTESIAN_POINT('Ctrl Pts',(0.85354996579394,-1.87042214376343,7.21859532926579));
#48722=CARTESIAN_POINT('Ctrl Pts',(0.788323957946326,-1.89884362351522,
7.21472636062447));
#48723=CARTESIAN_POINT('Ctrl Pts',(0.721694646449377,-1.92383845470099,
7.21085739198316));
#48724=CARTESIAN_POINT('Ctrl Pts',(0.655164614492342,-1.94879604288839,
7.20699418821345));
#48725=CARTESIAN_POINT('Ctrl Pts',(0.58723588053482,-1.97033694812449,7.20313098444375));
#48726=CARTESIAN_POINT('Ctrl Pts',(0.51829289493829,-1.98830833563522,7.19926778067405));
#48727=CARTESIAN_POINT('Ctrl Pts',(0.449430775593098,-2.00625864371739,
7.19540910822547));
#48728=CARTESIAN_POINT('Ctrl Pts',(0.379557235495024,-2.02064762859855,
7.19155043577689));
#48729=CARTESIAN_POINT('Ctrl Pts',(0.309073444491057,-2.0313717454987,7.18769176332832));
#48730=CARTESIAN_POINT('Ctrl Pts',(0.238634049373333,-2.04208910755965,
7.18383552135603));
#48731=CARTESIAN_POINT('Ctrl Pts',(0.167585645105574,-2.04914610856388,
7.17997927938375));
#48732=CARTESIAN_POINT('Ctrl Pts',(0.0963397545169107,-2.05249024704129,
7.17612303741146));
#48733=CARTESIAN_POINT('Ctrl Pts',(0.0251149031738014,-2.05583339797893,
7.17226793420551));
#48734=CARTESIAN_POINT('Ctrl Pts',(-0.0463068336956827,-2.05546584032901,
7.16841283099957));
#48735=CARTESIAN_POINT('Ctrl Pts',(-0.117510377601777,-2.05138706090681,
7.16455772779362));
#48736=CARTESIAN_POINT('Ctrl Pts',(-0.188716716584823,-2.04730812137317,
7.16070247325657));
#48737=CARTESIAN_POINT('Ctrl Pts',(-0.259704360706126,-2.03951770081616,
7.15684721871953));
#48738=CARTESIAN_POINT('Ctrl Pts',(-0.330061539169524,-2.02806729248835,
7.15299196418249));
#48739=CARTESIAN_POINT('Ctrl Pts',(-0.400492395360941,-2.01660489334328,
7.14913267243984));
#48740=CARTESIAN_POINT('Ctrl Pts',(-0.470290987458039,-2.00147493365622,
7.1452733806972));
#48741=CARTESIAN_POINT('Ctrl Pts',(-0.539054847388912,-1.98278022836786,
7.14141408895455));
#48742=CARTESIAN_POINT('Ctrl Pts',(-0.60785765704541,-1.96407493388858,
7.13755261120381));
#48743=CARTESIAN_POINT('Ctrl Pts',(-0.675624106053599,-1.94180102604834,
7.13369113345307));
#48744=CARTESIAN_POINT('Ctrl Pts',(-0.74196866205707,-1.91611066147685,
7.12982965570232));
#48745=CARTESIAN_POINT('Ctrl Pts',(-0.808429335272795,-1.89037533325354,
7.12596141953675));
#48746=CARTESIAN_POINT('Ctrl Pts',(-0.873462703469705,-1.86121180885213,
7.12209318337116));
#48747=CARTESIAN_POINT('Ctrl Pts',(-0.936705558148894,-1.82881936227528,
7.11822494720559));
#48748=CARTESIAN_POINT('Ctrl Pts',(-0.974274922604166,-1.80957665672038,
7.1159270247756));
#48749=CARTESIAN_POINT('Ctrl Pts',(-1.01121292152412,-1.78919535023045,
7.11362910234561));
#48750=CARTESIAN_POINT('Ctrl Pts',(-1.0474483806814,-1.76772437113593,7.11133117991563));
#48751=CARTESIAN_POINT('Ctrl Pts',(-1.10846071388344,-1.73157208933364,
7.10746199729088));
#48752=CARTESIAN_POINT('Ctrl Pts',(-1.16771865797709,-1.69218657582534,
7.10359281466615));
#48753=CARTESIAN_POINT('Ctrl Pts',(-1.22485861391118,-1.64976329769685,
7.09972363204141));
#48754=CARTESIAN_POINT('Ctrl Pts',(-1.28191342573315,-1.60740323439396,
7.09586021487647));
#48755=CARTESIAN_POINT('Ctrl Pts',(-1.33685612715621,-1.56201467879785,
7.09199679771154));
#48756=CARTESIAN_POINT('Ctrl Pts',(-1.38934977746784,-1.51383775826542,
7.08813338054661));
#48757=CARTESIAN_POINT('Ctrl Pts',(-1.44178183362564,-1.46571736679197,
7.08427449657587));
#48758=CARTESIAN_POINT('Ctrl Pts',(-1.49177019053785,-1.41481543609068,
7.08041561260514));
#48759=CARTESIAN_POINT('Ctrl Pts',(-1.5390102509223,-1.36141287273776,7.07655672863441));
#48760=CARTESIAN_POINT('Ctrl Pts',(-1.58622054216656,-1.30804396193275,
7.07270027640608));
#48761=CARTESIAN_POINT('Ctrl Pts',(-1.63068565183867,-1.25217790785008,
7.06884382417774));
#48762=CARTESIAN_POINT('Ctrl Pts',(-1.67213825123546,-1.1941319990919,7.06498737194941));
#48763=CARTESIAN_POINT('Ctrl Pts',(-1.71357859336585,-1.13610325413473,
7.06113206004914));
#48764=CARTESIAN_POINT('Ctrl Pts',(-1.75200791152176,-1.07589632924174,
7.05727674814888));
#48765=CARTESIAN_POINT('Ctrl Pts',(-1.78720062565951,-1.01385969746423,
7.05342143624861));
#48766=CARTESIAN_POINT('Ctrl Pts',(-1.82239470423566,-0.951820660496772,
7.04956597487605));
#48767=CARTESIAN_POINT('Ctrl Pts',(-1.85435169189239,-0.88795219939876,
7.04571051350349));
#48768=CARTESIAN_POINT('Ctrl Pts',(-1.88289149465536,-0.82262821605783,
7.04185505213093));
#48769=CARTESIAN_POINT('Ctrl Pts',(-1.91146115126503,-0.757235901053905,
7.03799555778191));
#48770=CARTESIAN_POINT('Ctrl Pts',(-1.93660629255638,-0.690385470517167,
7.03413606343289));
#48771=CARTESIAN_POINT('Ctrl Pts',(-1.95819498690959,-0.622470847303041,
7.03027656908387));
#48772=CARTESIAN_POINT('Ctrl Pts',(-1.97979589741874,-0.554517793991437,
7.02641489080542));
#48773=CARTESIAN_POINT('Ctrl Pts',(-1.99783623190938,-0.485499819428284,
7.02255321252697));
#48774=CARTESIAN_POINT('Ctrl Pts',(-2.01223469734867,-0.415823382322472,
7.01869153424853));
#48775=CARTESIAN_POINT('Ctrl Pts',(-2.0266583416096,-0.346025100941707,
7.0148231029929));
#48776=CARTESIAN_POINT('Ctrl Pts',(-2.03742732831468,-0.275566538420227,
7.01095467173727));
#48777=CARTESIAN_POINT('Ctrl Pts',(-2.04451205699333,-0.204860956038284,
7.00708624048164));
#48778=CARTESIAN_POINT('Ctrl Pts',(-2.04871711006231,-0.162894532244804,
7.00479018096243));
#48779=CARTESIAN_POINT('Ctrl Pts',(-2.05162524471206,-0.120841139796805,
7.00249412144322));
#48780=CARTESIAN_POINT('Ctrl Pts',(-2.05323895034625,-0.0787868979021409,
7.000198061924));
#48781=CARTESIAN_POINT('Ctrl Pts',(-2.05423994231227,-0.0527003816366956,
6.9987738014619));
#48782=CARTESIAN_POINT('Ctrl Pts',(-2.05474381156835,-0.0265946663309218,
6.99734954099979));
#48783=CARTESIAN_POINT('Ctrl Pts',(-2.05474994334785,-0.000482505981838667,
6.99592528053767));
#48784=CARTESIAN_POINT('Ctrl Pts',(-2.05474994334797,-0.000482505435243929,
6.99592528050786));
#48785=CARTESIAN_POINT('Ctrl Pts',(-2.05476649816122,0.0700161855421443,
6.99208000317933));
#48786=CARTESIAN_POINT('Ctrl Pts',(-2.05115055191818,0.140660126107189,
6.98823472585081));
#48787=CARTESIAN_POINT('Ctrl Pts',(-2.04388336541941,0.211041112254987,
6.98438944852229));
#48788=CARTESIAN_POINT('Ctrl Pts',(-2.03637696109566,0.283738866581148,
6.98041759416438));
#48789=CARTESIAN_POINT('Ctrl Pts',(-2.0249746271749,0.356155527681318,6.97644573980647));
#48790=CARTESIAN_POINT('Ctrl Pts',(-2.0097141915556,0.427839258086527,6.97247388544856));
#48791=CARTESIAN_POINT('Ctrl Pts',(-1.99497874903466,0.497056907924543,
6.96863867175921));
#48792=CARTESIAN_POINT('Ctrl Pts',(-1.97664644609815,0.565590706630233,
6.96480345806987));
#48793=CARTESIAN_POINT('Ctrl Pts',(-1.95480391551666,0.633039662565255,
6.96096824438053));
#48794=CARTESIAN_POINT('Ctrl Pts',(-1.93297398344573,0.70044971474872,6.9571352427966));
#48795=CARTESIAN_POINT('Ctrl Pts',(-1.90763799081597,0.766775697756702,
6.95330224121267));
#48796=CARTESIAN_POINT('Ctrl Pts',(-1.87893281749727,0.831630344463081,
6.94946923962874));
#48797=CARTESIAN_POINT('Ctrl Pts',(-1.8502342985522,0.896469956700014,6.94563712660327));
#48798=CARTESIAN_POINT('Ctrl Pts',(-1.81816834880263,0.959838459735692,
6.9418050135778));
#48799=CARTESIAN_POINT('Ctrl Pts',(-1.78291984061563,1.02136888754217,6.93797290055234));
#48800=CARTESIAN_POINT('Ctrl Pts',(-1.7476673440786,1.08290627748397,6.93414035392531));
#48801=CARTESIAN_POINT('Ctrl Pts',(-1.70923182180326,1.14260475376583,6.93030780729828));
#48802=CARTESIAN_POINT('Ctrl Pts',(-1.66784300479209,1.20012385771889,6.92647526067126));
#48803=CARTESIAN_POINT('Ctrl Pts',(-1.62640938656058,1.25770522308064,6.92263856551382));
#48804=CARTESIAN_POINT('Ctrl Pts',(-1.58201638538156,1.31310211060008,6.91880187035639));
#48805=CARTESIAN_POINT('Ctrl Pts',(-1.53493515674473,1.36600572000597,6.91496517519895));
#48806=CARTESIAN_POINT('Ctrl Pts',(-1.48782324497298,1.41894380702921,6.91112597964298));
#48807=CARTESIAN_POINT('Ctrl Pts',(-1.43801996747691,1.46938503482276,6.90728678408701));
#48808=CARTESIAN_POINT('Ctrl Pts',(-1.38583263452308,1.51705816354905,6.90344758853104));
#48809=CARTESIAN_POINT('Ctrl Pts',(-1.33355967559132,1.5648095116063,6.89960209384354));
#48810=CARTESIAN_POINT('Ctrl Pts',(-1.27889524014262,1.60978339213117,6.89575659915605));
#48811=CARTESIAN_POINT('Ctrl Pts',(-1.22217805839316,1.65175008887008,6.89191110446856));
#48812=CARTESIAN_POINT('Ctrl Pts',(-1.20818538926298,1.66210367280781,6.89096238428987));
#48813=CARTESIAN_POINT('Ctrl Pts',(-1.19406790386411,1.67227443734968,6.89001366411119));
#48814=CARTESIAN_POINT('Ctrl Pts',(-1.17983092207496,1.68225936104269,6.8890649439325));
#48815=CARTESIAN_POINT('Ctrl Pts',(-1.12178147454127,1.7229715929349,6.88519666039794));
#48816=CARTESIAN_POINT('Ctrl Pts',(-1.0615083071561,1.76075557326182,6.88132837686337));
#48817=CARTESIAN_POINT('Ctrl Pts',(-0.999339045620557,1.79536041907974,
6.87746009332881));
#48818=CARTESIAN_POINT('Ctrl Pts',(-0.937262455615625,1.8299136817849,6.87359757598395));
#48819=CARTESIAN_POINT('Ctrl Pts',(-0.873295802853424,1.86129698204855,
6.8697350586391));
#48820=CARTESIAN_POINT('Ctrl Pts',(-0.807796451145422,1.8893021081915,6.86587254129424));
#48821=CARTESIAN_POINT('Ctrl Pts',(-0.742373917871417,1.9172743895829,6.86201455395657));
#48822=CARTESIAN_POINT('Ctrl Pts',(-0.675422700874369,1.94187617640339,
6.85815656661889));
#48823=CARTESIAN_POINT('Ctrl Pts',(-0.607324023697059,1.96294551446045,
6.85429857928122));
#48824=CARTESIAN_POINT('Ctrl Pts',(-0.5392682270093,1.98400158554131,6.8504430212475));
#48825=CARTESIAN_POINT('Ctrl Pts',(-0.470066866807601,2.00152947749453,
6.84658746321378));
#48826=CARTESIAN_POINT('Ctrl Pts',(-0.400118988439783,2.01541617478622,
6.84273190518006));
#48827=CARTESIAN_POINT('Ctrl Pts',(-0.330191730537803,2.02929877831305,
6.83887748375555));
#48828=CARTESIAN_POINT('Ctrl Pts',(-0.259518867808598,2.0395422235871,6.83502306233104));
#48829=CARTESIAN_POINT('Ctrl Pts',(-0.188510683422475,2.04608437869399,
6.83116864090653));
#48830=CARTESIAN_POINT('Ctrl Pts',(-0.1174996532212,2.0526267959927,6.82731406500728));
#48831=CARTESIAN_POINT('Ctrl Pts',(-0.046153758839543,2.05546758622967,
6.82345948910803));
#48832=CARTESIAN_POINT('Ctrl Pts',(0.0251122658282849,2.05459653864329,
6.81960491320877));
#48833=CARTESIAN_POINT('Ctrl Pts',(0.0964531072273813,2.05372457661087,
6.81574629068604));
#48834=CARTESIAN_POINT('Ctrl Pts',(0.167713424566388,2.04913300390706,6.8118876681633));
#48835=CARTESIAN_POINT('Ctrl Pts',(0.238480064451791,2.04086374394742,6.80802904564056));
#48836=CARTESIAN_POINT('Ctrl Pts',(0.309286874236735,2.03258979003392,6.80416823281348));
#48837=CARTESIAN_POINT('Ctrl Pts',(0.379598969382153,2.02063407471531,6.80030741998639));
#48838=CARTESIAN_POINT('Ctrl Pts',(0.449012623742548,2.0050898299627,6.7964466071593));
#48839=CARTESIAN_POINT('Ctrl Pts',(0.518548039110839,1.98951831848676,6.79257902194045));
#48840=CARTESIAN_POINT('Ctrl Pts',(0.587181398984335,1.97034584076531,6.7887114367216));
#48841=CARTESIAN_POINT('Ctrl Pts',(0.654524062957153,1.94771553711266,6.78484385150275));
#48842=CARTESIAN_POINT('Ctrl Pts',(0.694641620247931,1.93423415028099,6.78253984298213));
#48843=CARTESIAN_POINT('Ctrl Pts',(0.734301491181396,1.919526565114,6.78023583446152));
#48844=CARTESIAN_POINT('Ctrl Pts',(0.773425401480044,1.90363092821204,6.77793182594091));
#48845=CARTESIAN_POINT('Ctrl Pts',(0.839137179113808,1.87693291798056,6.77406205693221));
#48846=CARTESIAN_POINT('Ctrl Pts',(0.903593417992809,1.84677624309011,6.7701922879235));
#48847=CARTESIAN_POINT('Ctrl Pts',(0.966405487979356,1.81330030477673,6.7663225189148));
#48848=CARTESIAN_POINT('Ctrl Pts',(1.02911755148771,1.77987766530696,6.76245891117368));
#48849=CARTESIAN_POINT('Ctrl Pts',(1.09019021993631,1.7431464839298,6.75859530343255));
#48850=CARTESIAN_POINT('Ctrl Pts',(1.14925471029172,1.70329421221711,6.75473169569142));
#48851=CARTESIAN_POINT('Ctrl Pts',(1.18425395175351,1.67967935882414,6.752442277135));
#48852=CARTESIAN_POINT('Ctrl Pts',(1.21854844377853,1.65496952297849,6.75015285857857));
#48853=CARTESIAN_POINT('Ctrl Pts',(1.25206542099589,1.62921138715833,6.74786344002215));
#48854=CARTESIAN_POINT('',(-2.05138364312766,-4.97672492245568E-5,7.05407471946232));
#48855=CARTESIAN_POINT('Ctrl Pts',(-2.05138364312766,-4.97672492245568E-5,
7.05407471946232));
#48856=CARTESIAN_POINT('Ctrl Pts',(-2.05130984591811,0.345894061862528,
7.03538960656144));
#48857=CARTESIAN_POINT('Ctrl Pts',(-1.80422556460434,1.37779248996311,6.97966012099671));
#48858=CARTESIAN_POINT('Ctrl Pts',(-0.348743598875701,2.30840998533453,
6.89702663395796));
#48859=CARTESIAN_POINT('Ctrl Pts',(0.854945852554142,1.92735221205475,6.8330782598201));
#48860=CARTESIAN_POINT('Ctrl Pts',(1.2515670322334,1.6285464922234,6.80617425834608));
#48861=CARTESIAN_POINT('Ctrl Pts',(1.25017377660034,1.6267706489614,7.50603355970618));
#48862=CARTESIAN_POINT('Ctrl Pts',(1.5598047990933,1.38694935814498,7.48487299071277));
#48863=CARTESIAN_POINT('Ctrl Pts',(2.23443033275686,0.494010394005184,7.42666804905549));
#48864=CARTESIAN_POINT('Ctrl Pts',(1.93017314387361,-1.47391051494563,7.33141873473435));
#48865=CARTESIAN_POINT('Ctrl Pts',(-0.191394880396712,-2.42102228346136,
7.2202856167428));
#48866=CARTESIAN_POINT('Ctrl Pts',(-1.81053415964382,-1.36562854594273,
7.12783761165212));
#48867=CARTESIAN_POINT('Ctrl Pts',(-2.05145615337403,-0.339960617975842,
7.07243397922529));
#48868=CARTESIAN_POINT('Ctrl Pts',(-2.05138364312766,-4.97672492245568E-5,
7.05407471946232));
#48869=CARTESIAN_POINT('Origin',(0.,0.,18.5459252805377));
#48870=CARTESIAN_POINT('',(1.25206542099588,1.62921138715834,8.20601752898817));
#48871=CARTESIAN_POINT('',(1.25206542099587,1.62921138715835,8.14797786267567));
#48872=CARTESIAN_POINT('',(1.25206542099588,1.62921138715835,18.5459252805377));
#48873=CARTESIAN_POINT('',(-2.05474915274975,0.00186595128382746,7.69592528050275));
#48874=CARTESIAN_POINT('Ctrl Pts',(1.25206542099587,1.62921138715835,8.14797786267567));
#48875=CARTESIAN_POINT('Ctrl Pts',(1.30862937348997,1.58574141785237,8.14411762025649));
#48876=CARTESIAN_POINT('Ctrl Pts',(1.36288888657392,1.53935147309315,8.14025737783731));
#48877=CARTESIAN_POINT('Ctrl Pts',(1.41454133522346,1.49032559309844,8.13639713541813));
#48878=CARTESIAN_POINT('Ctrl Pts',(1.46623000761081,1.4412653313722,8.13253418582025));
#48879=CARTESIAN_POINT('Ctrl Pts',(1.51530764476965,1.38956580912633,8.12867123622236));
#48880=CARTESIAN_POINT('Ctrl Pts',(1.56151034420752,1.33554595856261,8.12480828662448));
#48881=CARTESIAN_POINT('Ctrl Pts',(1.60778777584696,1.28143873166783,8.12093908876119));
#48882=CARTESIAN_POINT('Ctrl Pts',(1.65118070213744,1.22500407644762,8.11706989089792));
#48883=CARTESIAN_POINT('Ctrl Pts',(1.69146772913563,1.1665909667886,8.11320069303463));
#48884=CARTESIAN_POINT('Ctrl Pts',(1.69726891427347,1.15817969177384,8.1126435426363));
#48885=CARTESIAN_POINT('Ctrl Pts',(1.70300577641057,1.14972743544356,8.11208639223796));
#48886=CARTESIAN_POINT('Ctrl Pts',(1.70867773369655,1.14123528024225,8.11152924183962));
#48887=CARTESIAN_POINT('Ctrl Pts',(1.74806615162049,1.08226224125779,8.10766015897639));
#48888=CARTESIAN_POINT('Ctrl Pts',(1.78447505278231,1.0211321340826,8.10379107611316));
#48889=CARTESIAN_POINT('Ctrl Pts',(1.81766106723981,0.958178379604047,8.09992199324993));
#48890=CARTESIAN_POINT('Ctrl Pts',(1.85079763616627,0.895318423126603,8.09605867513007));
#48891=CARTESIAN_POINT('Ctrl Pts',(1.88072062542548,0.830640639033089,8.09219535701021));
#48892=CARTESIAN_POINT('Ctrl Pts',(1.90723000933527,0.764507196820929,8.08833203889035));
#48893=CARTESIAN_POINT('Ctrl Pts',(1.93370829771863,0.698451329184138,8.08447325244542));
#48894=CARTESIAN_POINT('Ctrl Pts',(1.95678075450588,0.63094364379623,8.0806144660005));
#48895=CARTESIAN_POINT('Ctrl Pts',(1.97629414719287,0.562369101454931,8.07675567955558));
#48896=CARTESIAN_POINT('Ctrl Pts',(1.99579524785997,0.493837756093833,8.0728993238658));
#48897=CARTESIAN_POINT('Ctrl Pts',(2.0117415997834,0.424241353231035,8.06904296817602));
#48898=CARTESIAN_POINT('Ctrl Pts',(2.02402930427195,0.353981550293792,8.06518661248625));
#48899=CARTESIAN_POINT('Ctrl Pts',(2.0363133788412,0.283742502853662,8.06133139600518));
#48900=CARTESIAN_POINT('Ctrl Pts',(2.04494086802811,0.212840922664285,8.05747617952411));
#48901=CARTESIAN_POINT('Ctrl Pts',(2.04985900006653,0.141688539925573,8.05362096304304));
#48902=CARTESIAN_POINT('Ctrl Pts',(2.05477732438586,0.0705333753898392,
8.04976559583716));
#48903=CARTESIAN_POINT('Ctrl Pts',(2.05598597233378,-0.00087212638403536,
8.04591022863127));
#48904=CARTESIAN_POINT('Ctrl Pts',(2.0534841811616,-0.0721129684526676,
8.04205486142539));
#48905=CARTESIAN_POINT('Ctrl Pts',(2.05097977129884,-0.143428380183379,
8.03819545870531));
#48906=CARTESIAN_POINT('Ctrl Pts',(2.04475718643642,-0.214578301673897,
8.03433605598523));
#48907=CARTESIAN_POINT('Ctrl Pts',(2.03486774836884,-0.28515050262682,8.03047665326515));
#48908=CARTESIAN_POINT('Ctrl Pts',(2.02497271082948,-0.355762662073375,
8.02661506532316));
#48909=CARTESIAN_POINT('Ctrl Pts',(2.01140677943915,-0.425795972664315,
8.02275347738118));
#48910=CARTESIAN_POINT('Ctrl Pts',(1.99427235752724,-0.494848791554304,
8.0188918894392));
#48911=CARTESIAN_POINT('Ctrl Pts',(1.97710795834521,-0.564022420764869,
8.01502354551412));
#48912=CARTESIAN_POINT('Ctrl Pts',(1.95636274535452,-0.632211668522653,
8.01115520158904));
#48913=CARTESIAN_POINT('Ctrl Pts',(1.93218867531514,-0.699031104804307,
8.00728685766396));
#48914=CARTESIAN_POINT('Ctrl Pts',(1.91783480837926,-0.738706562662871,
8.004989946392));
#48915=CARTESIAN_POINT('Ctrl Pts',(1.90227297183507,-0.777899457293998,
8.00269303512003));
#48916=CARTESIAN_POINT('Ctrl Pts',(1.88554268645341,-0.816533122452525,
8.00039612384806));
#48917=CARTESIAN_POINT('Ctrl Pts',(1.85736098084715,-0.881610468902424,
7.99652703998047));
#48918=CARTESIAN_POINT('Ctrl Pts',(1.82575101799983,-0.945354574838809,
7.99265795611289));
#48919=CARTESIAN_POINT('Ctrl Pts',(1.79086091697388,-1.00738013607351,7.9887888722453));
#48920=CARTESIAN_POINT('Ctrl Pts',(1.75602280040168,-1.06931328241617,7.98492555311343));
#48921=CARTESIAN_POINT('Ctrl Pts',(1.71791448290529,-1.12953254671932,7.98106223398155));
#48922=CARTESIAN_POINT('Ctrl Pts',(1.67673174527057,-1.18767344708128,7.97719891484968));
#48923=CARTESIAN_POINT('Ctrl Pts',(1.63559731493566,-1.2457461482397,7.97334012738632));
#48924=CARTESIAN_POINT('Ctrl Pts',(1.59139590720388,-1.30174493350011,7.96948133992297));
#48925=CARTESIAN_POINT('Ctrl Pts',(1.54436783027611,-1.35533227192016,7.96562255245962));
#48926=CARTESIAN_POINT('Ctrl Pts',(1.4973693775712,-1.40888585426597,7.961766195748));
#48927=CARTESIAN_POINT('Ctrl Pts',(1.44754810800904,-1.46003063925531,7.95790983903638));
#48928=CARTESIAN_POINT('Ctrl Pts',(1.39518511486163,-1.50846148700208,7.95405348232477));
#48929=CARTESIAN_POINT('Ctrl Pts',(1.34283759027272,-1.55687802778593,7.95019826481998));
#48930=CARTESIAN_POINT('Ctrl Pts',(1.28795018918138,-1.60258189330383,7.94634304731519));
#48931=CARTESIAN_POINT('Ctrl Pts',(1.23084019755949,-1.64530543382428,7.94248782981041));
#48932=CARTESIAN_POINT('Ctrl Pts',(1.17372797314172,-1.68803064468196,7.93863246158044));
#48933=CARTESIAN_POINT('Ctrl Pts',(1.11439337597587,-1.7277750099764,7.93477709335047));
#48934=CARTESIAN_POINT('Ctrl Pts',(1.05318464519525,-1.76431280265857,7.93092172512051));
#48935=CARTESIAN_POINT('Ctrl Pts',(0.991911845747888,-1.80088884033673,
7.92706232138287));
#48936=CARTESIAN_POINT('Ctrl Pts',(0.928761414662859,-1.83425135577758,
7.92320291764524));
#48937=CARTESIAN_POINT('Ctrl Pts',(0.864107516350061,-1.86421988045599,
7.9193435139076));
#48938=CARTESIAN_POINT('Ctrl Pts',(0.799417010575119,-1.89420537351002,
7.91548192495021));
#48939=CARTESIAN_POINT('Ctrl Pts',(0.733221793944371,-1.9207928691467,7.91162033599281));
#48940=CARTESIAN_POINT('Ctrl Pts',(0.66591484161939,-1.9438505565529,7.90775874703542));
#48941=CARTESIAN_POINT('Ctrl Pts',(0.598490133711226,-1.96694858409238,
7.90389040210937));
#48942=CARTESIAN_POINT('Ctrl Pts',(0.529950274118068,-1.98650434049851,
7.90002205718333));
#48943=CARTESIAN_POINT('Ctrl Pts',(0.460701493880856,-2.00243643994908,
7.89615371225729));
#48944=CARTESIAN_POINT('Ctrl Pts',(0.41958373573966,-2.01189642191044,7.8938568101237));
#48945=CARTESIAN_POINT('Ctrl Pts',(0.37821621810489,-2.02007982598716,7.8915599079901));
#48946=CARTESIAN_POINT('Ctrl Pts',(0.336684785059664,-2.02697827270282,
7.88926300585651));
#48947=CARTESIAN_POINT('Ctrl Pts',(0.266726007745194,-2.03859855310758,
7.88539392518447));
#48948=CARTESIAN_POINT('Ctrl Pts',(0.196027910386645,-2.04661552383361,
7.88152484451243));
#48949=CARTESIAN_POINT('Ctrl Pts',(0.124994536013101,-2.05094464295526,
7.87765576384039));
#48950=CARTESIAN_POINT('Ctrl Pts',(0.0540669978723382,-2.05526731190242,
7.87379244790819));
#48951=CARTESIAN_POINT('Ctrl Pts',(-0.0171943447640447,-2.05591300679656,
7.86992913197598));
#48952=CARTESIAN_POINT('Ctrl Pts',(-0.0883770915285675,-2.05284852149226,
7.86606581604377));
#48953=CARTESIAN_POINT('Ctrl Pts',(-0.159476341118476,-2.04978763082116,
7.86220703177099));
#48954=CARTESIAN_POINT('Ctrl Pts',(-0.230496694983797,-2.0430252253523,
7.8583482474982));
#48955=CARTESIAN_POINT('Ctrl Pts',(-0.301024244314913,-2.03258012556323,
7.85448946322541));
#48956=CARTESIAN_POINT('Ctrl Pts',(-0.371507366584102,-2.02214160540297,
7.85063310969706));
#48957=CARTESIAN_POINT('Ctrl Pts',(-0.441497820800681,-2.00802506441071,
7.84677675616871));
#48958=CARTESIAN_POINT('Ctrl Pts',(-0.510586789906049,-1.99030115622572,
7.84292040264035));
#48959=CARTESIAN_POINT('Ctrl Pts',(-0.579655349626495,-1.97258248381236,
7.83906518830693));
#48960=CARTESIAN_POINT('Ctrl Pts',(-0.647822482635188,-1.95125868044958,
7.83520997397351));
#48961=CARTESIAN_POINT('Ctrl Pts',(-0.714691238369664,-1.92645114038681,
7.83135475964009));
#48962=CARTESIAN_POINT('Ctrl Pts',(-0.781562608720652,-1.90164263033136,
7.82749939456501));
#48963=CARTESIAN_POINT('Ctrl Pts',(-0.847135046320205,-1.87335028416826,
7.82364402948994));
#48964=CARTESIAN_POINT('Ctrl Pts',(-0.911030032849573,-1.84174423896102,
7.81978866441486));
#48965=CARTESIAN_POINT('Ctrl Pts',(-0.974991900642846,-1.81010511052824,
7.81592926378546));
#48966=CARTESIAN_POINT('Ctrl Pts',(-1.03727237597784,-1.77514557483067,
7.81206986315606));
#48967=CARTESIAN_POINT('Ctrl Pts',(-1.09751690236007,-1.73708209694705,
7.80821046252666));
#48968=CARTESIAN_POINT('Ctrl Pts',(-1.15779553995399,-1.69899706704154,
7.80434887665588));
#48969=CARTESIAN_POINT('Ctrl Pts',(-1.21603553697043,-1.65780487697403,
7.8004872907851));
#48970=CARTESIAN_POINT('Ctrl Pts',(-1.27191301330507,-1.61376418633121,
7.79662570491432));
#48971=CARTESIAN_POINT('Ctrl Pts',(-1.32788825005739,-1.56964644431466,
7.79275736300744));
#48972=CARTESIAN_POINT('Ctrl Pts',(-1.38149234832285,-1.5226705721095,7.78888902110056));
#48973=CARTESIAN_POINT('Ctrl Pts',(-1.43243660198821,-1.47313371551413,
7.78502067919368));
#48974=CARTESIAN_POINT('Ctrl Pts',(-1.46268610163228,-1.44371989514897,
7.78272374875077));
#48975=CARTESIAN_POINT('Ctrl Pts',(-1.49199854774675,-1.41340383043145,
7.78042681830785));
#48976=CARTESIAN_POINT('Ctrl Pts',(-1.52032033835932,-1.38225309957004,
7.77812988786494));
#48977=CARTESIAN_POINT('Ctrl Pts',(-1.56750900270051,-1.33035096517784,
7.77430283182995));
#48978=CARTESIAN_POINT('Ctrl Pts',(-1.61213921803362,-1.27591667902572,
7.77047577579496));
#48979=CARTESIAN_POINT('Ctrl Pts',(-1.65392332358744,-1.21923549907042,
7.76664871975997));
#48980=CARTESIAN_POINT('Ctrl Pts',(-1.69565022628001,-1.16263191622123,
7.76282690300322));
#48981=CARTESIAN_POINT('Ctrl Pts',(-1.73453845065562,-1.10378793291417,
7.75900508624648));
#48982=CARTESIAN_POINT('Ctrl Pts',(-1.77033843346293,-1.04302415767997,
7.75518326948973));
#48983=CARTESIAN_POINT('Ctrl Pts',(-1.80610200917414,-0.98232217668228,
7.75136533936195));
#48984=CARTESIAN_POINT('Ctrl Pts',(-1.83878332051712,-0.91970470131575,
7.74754740923417));
#48985=CARTESIAN_POINT('Ctrl Pts',(-1.8681753626088,-0.855522283194004,
7.74372947910639));
#48986=CARTESIAN_POINT('Ctrl Pts',(-1.89884344211489,-0.788553424898569,
7.73974579589233));
#48987=CARTESIAN_POINT('Ctrl Pts',(-1.92592979667686,-0.719881098031171,
7.73576211267827));
#48988=CARTESIAN_POINT('Ctrl Pts',(-1.94925262780642,-0.649932116062723,
7.73177842946421));
#48989=CARTESIAN_POINT('Ctrl Pts',(-1.97158882915295,-0.582942198048359,
7.72796326869424));
#48990=CARTESIAN_POINT('Ctrl Pts',(-1.99047337491429,-0.514781984415854,
7.72414810792428));
#48991=CARTESIAN_POINT('Ctrl Pts',(-2.00579666901848,-0.445844462850394,
7.72033294715431));
#48992=CARTESIAN_POINT('Ctrl Pts',(-2.02112012375057,-0.376906218640789,
7.71651774639156));
#48993=CARTESIAN_POINT('Ctrl Pts',(-2.03288215514213,-0.307191137845921,
7.71270254562881));
#48994=CARTESIAN_POINT('Ctrl Pts',(-2.04102422708131,-0.237102650696173,
7.70888734486606));
#48995=CARTESIAN_POINT('Ctrl Pts',(-2.04917190604306,-0.166965897241075,
7.70506951677245));
#48996=CARTESIAN_POINT('Ctrl Pts',(-2.05369461174166,-0.0964557197208807,
7.70125168867884));
#48997=CARTESIAN_POINT('Ctrl Pts',(-2.05458575673003,-0.0259794292098742,
7.69743386058524));
#48998=CARTESIAN_POINT('Ctrl Pts',(-2.05470313267573,-0.0166967408083679,
7.69693100056938));
#48999=CARTESIAN_POINT('Ctrl Pts',(-2.05475758060194,-0.0074146383491741,
7.69642814055353));
#49000=CARTESIAN_POINT('Ctrl Pts',(-2.05474915275033,0.00186595063910761,
7.69592528053768));
#49001=CARTESIAN_POINT('Ctrl Pts',(-2.05474915274975,0.00186595128382797,
7.69592528050275));
#49002=CARTESIAN_POINT('Ctrl Pts',(-2.05466653542133,0.0928425416364572,
7.69099579922465));
#49003=CARTESIAN_POINT('Ctrl Pts',(-2.04853795670126,0.183549917638068,
7.68606631794656));
#49004=CARTESIAN_POINT('Ctrl Pts',(-2.03649277600636,0.273303376806667,
7.68113683666846));
#49005=CARTESIAN_POINT('Ctrl Pts',(-2.0249756981114,0.359121730783211,7.67642348107011));
#49006=CARTESIAN_POINT('Ctrl Pts',(-2.00804990481639,0.444068412205174,
7.67171012547175));
#49007=CARTESIAN_POINT('Ctrl Pts',(-1.9858683953167,0.527564478506904,7.66699676987339));
#49008=CARTESIAN_POINT('Ctrl Pts',(-1.96766008569713,0.596104549112073,
7.66312768070779));
#49009=CARTESIAN_POINT('Ctrl Pts',(-1.9458635701162,0.663835094034513,7.65925859154218));
#49010=CARTESIAN_POINT('Ctrl Pts',(-1.92056812646636,0.730353088650609,
7.65538950237658));
#49011=CARTESIAN_POINT('Ctrl Pts',(-1.89531037146572,0.796771975561802,
7.65152617791494));
#49012=CARTESIAN_POINT('Ctrl Pts',(-1.86656420769144,0.861981447908525,
7.6476628534533));
#49013=CARTESIAN_POINT('Ctrl Pts',(-1.83446913779108,0.925591997044075,
7.64379952899166));
#49014=CARTESIAN_POINT('Ctrl Pts',(-1.80241171513912,0.989127931537845,
7.63994073617728));
#49015=CARTESIAN_POINT('Ctrl Pts',(-1.76701340693965,1.0510682366476,7.6360819433629));
#49016=CARTESIAN_POINT('Ctrl Pts',(-1.72846175085154,1.11104344574963,7.63222315054852));
#49017=CARTESIAN_POINT('Ctrl Pts',(-1.6899343793302,1.17098087510061,7.62836678847568));
#49018=CARTESIAN_POINT('Ctrl Pts',(-1.64825786288973,1.22895525666185,7.62451042640283));
#49019=CARTESIAN_POINT('Ctrl Pts',(-1.60366488094096,1.28462310119997,7.62065406432999));
#49020=CARTESIAN_POINT('Ctrl Pts',(-1.55908507216608,1.3402745009487,7.6167988414617));
#49021=CARTESIAN_POINT('Ctrl Pts',(-1.51159081184357,1.39362033745739,7.61294361859342));
#49022=CARTESIAN_POINT('Ctrl Pts',(-1.46145613665084,1.44434882322297,7.60908839572513));
#49023=CARTESIAN_POINT('Ctrl Pts',(-1.41131950144824,1.4950792922134,7.60523302213731));
#49024=CARTESIAN_POINT('Ctrl Pts',(-1.35854258947012,1.54319186334069,7.60137764854948));
#49025=CARTESIAN_POINT('Ctrl Pts',(-1.30343627122762,1.58841161206667,7.59752227496166));
#49026=CARTESIAN_POINT('Ctrl Pts',(-1.24827227259226,1.63367869280384,7.59366286591165));
#49027=CARTESIAN_POINT('Ctrl Pts',(-1.19077437676783,1.67604659788638,7.58980345686166));
#49028=CARTESIAN_POINT('Ctrl Pts',(-1.13128581116102,1.71528131102911,7.58594404781165));
#49029=CARTESIAN_POINT('Ctrl Pts',(-1.07176356305579,1.75453823891429,7.58208245355954));
#49030=CARTESIAN_POINT('Ctrl Pts',(-1.01024882052389,1.79065819725059,7.57822085930742));
#49031=CARTESIAN_POINT('Ctrl Pts',(-0.947110636835177,1.82345249570524,
7.57435926505531));
#49032=CARTESIAN_POINT('Ctrl Pts',(-0.883861992499758,1.85630416798986,
7.57049091491993));
#49033=CARTESIAN_POINT('Ctrl Pts',(-0.818984678742866,1.88581836284658,
7.56662256478455));
#49034=CARTESIAN_POINT('Ctrl Pts',(-0.752868343745366,1.91185428824639,
7.56275421464917));
#49035=CARTESIAN_POINT('Ctrl Pts',(-0.713611404714169,1.92731326273552,
7.56045736039339));
#49036=CARTESIAN_POINT('Ctrl Pts',(-0.673917976614465,1.94154693435799,
7.55816050613761));
#49037=CARTESIAN_POINT('Ctrl Pts',(-0.633871702905928,1.95453427361997,
7.55586365188183));
#49038=CARTESIAN_POINT('Ctrl Pts',(-0.56641216747749,1.97641196140288,7.55199450984455));
#49039=CARTESIAN_POINT('Ctrl Pts',(-0.497686524259488,1.99483591590095,
7.54812536780728));
#49040=CARTESIAN_POINT('Ctrl Pts',(-0.428081808244282,2.00966254081383,
7.54425622577));
#49041=CARTESIAN_POINT('Ctrl Pts',(-0.355888897998268,2.02504048160384,
7.54024321286201));
#49042=CARTESIAN_POINT('Ctrl Pts',(-0.282750718369647,2.03654804692583,
7.53623019995401));
#49043=CARTESIAN_POINT('Ctrl Pts',(-0.209119137405439,2.04408090565682,
7.53221718704602));
#49044=CARTESIAN_POINT('Ctrl Pts',(-0.138320348723011,2.05132395634901,
7.52835856484706));
#49045=CARTESIAN_POINT('Ctrl Pts',(-0.0670659642655545,2.05489247764792,
7.5244999426481));
#49046=CARTESIAN_POINT('Ctrl Pts',(0.00423168083114419,2.05474564250112,
7.52064132044915));
#49047=CARTESIAN_POINT('Ctrl Pts',(0.0754847679454185,2.05459889912001,
7.51678510972423));
#49048=CARTESIAN_POINT('Ctrl Pts',(0.14678057739818,2.05074140756313,7.51292889899931));
#49049=CARTESIAN_POINT('Ctrl Pts',(0.217704390364775,2.04318436782291,7.50907268827439));
#49050=CARTESIAN_POINT('Ctrl Pts',(0.288607604665075,2.03562952290179,7.50521759752307));
#49051=CARTESIAN_POINT('Ctrl Pts',(0.359138554266875,2.02437731495336,7.50136250677175));
#49052=CARTESIAN_POINT('Ctrl Pts',(0.428886997541334,2.00949085736661,7.49750741602043));
#49053=CARTESIAN_POINT('Ctrl Pts',(0.498638515149956,1.99460374362262,7.4936521553465));
#49054=CARTESIAN_POINT('Ctrl Pts',(0.567606983521711,1.97608216631118,7.48979689467257));
#49055=CARTESIAN_POINT('Ctrl Pts',(0.635393421224808,1.95404011288516,7.48594163399864));
#49056=CARTESIAN_POINT('Ctrl Pts',(0.703245154887088,1.93197682723231,7.48208265970659));
#49057=CARTESIAN_POINT('Ctrl Pts',(0.769912123410777,1.90638644967083,7.47822368541454));
#49058=CARTESIAN_POINT('Ctrl Pts',(0.835012522395941,1.87743219583078,7.47436471112249));
#49059=CARTESIAN_POINT('Ctrl Pts',(0.900150331727464,1.84846130324992,7.47050351924703));
#49060=CARTESIAN_POINT('Ctrl Pts',(0.96371934678332,1.81612290688363,7.46664232737156));
#49061=CARTESIAN_POINT('Ctrl Pts',(1.02536206200968,1.78062635167832,7.4627811354961));
#49062=CARTESIAN_POINT('Ctrl Pts',(1.08709925014214,1.74507539486669,7.45891402600302));
#49063=CARTESIAN_POINT('Ctrl Pts',(1.14690384139378,1.70635688624157,7.45504691650995));
#49064=CARTESIAN_POINT('Ctrl Pts',(1.20444782450804,1.66472310025958,7.45117980701687));
#49065=CARTESIAN_POINT('Ctrl Pts',(1.22049823284037,1.65311043062381,7.45010117667064));
#49066=CARTESIAN_POINT('Ctrl Pts',(1.2363729737087,1.64127119153606,7.44902254632442));
#49067=CARTESIAN_POINT('Ctrl Pts',(1.25206542099588,1.62921138715835,7.44794391597819));
#49068=CARTESIAN_POINT('',(-2.05474920663131,-0.0018056433735876,7.75407471946232));
#49069=CARTESIAN_POINT('Ctrl Pts',(-2.05549758983786,-0.00179924508355834,
7.75407433641555));
#49070=CARTESIAN_POINT('Ctrl Pts',(-2.05046538848476,0.546255807336168,
7.72432225384672));
#49071=CARTESIAN_POINT('Ctrl Pts',(-1.5430773566099,1.78491604847996,7.65752579861402));
#49072=CARTESIAN_POINT('Ctrl Pts',(0.122430998286581,2.24741296338508,7.57484553971088));
#49073=CARTESIAN_POINT('Ctrl Pts',(1.0177547725044,1.80678822318179,7.5219173633766));
#49074=CARTESIAN_POINT('Ctrl Pts',(1.25017377660034,1.6267706489614,7.50603355970618));
#49075=CARTESIAN_POINT('Ctrl Pts',(1.25206542099588,1.62921138715834,8.20601752898817));
#49076=CARTESIAN_POINT('Ctrl Pts',(1.31084998697262,1.58403485394241,8.2019897386418));
#49077=CARTESIAN_POINT('Ctrl Pts',(1.36727460896177,1.53560488054058,8.19796194829543));
#49078=CARTESIAN_POINT('Ctrl Pts',(1.42096375839729,1.48420334180376,8.19393415794906));
#49079=CARTESIAN_POINT('Ctrl Pts',(1.47238898730883,1.43496926147769,8.19007620820041));
#49080=CARTESIAN_POINT('Ctrl Pts',(1.52130440251306,1.38300955213352,8.18621825845176));
#49081=CARTESIAN_POINT('Ctrl Pts',(1.56741308865996,1.32861347727525,8.18236030870311));
#49082=CARTESIAN_POINT('Ctrl Pts',(1.61349719502314,1.27424640007159,8.17850441556415));
#49083=CARTESIAN_POINT('Ctrl Pts',(1.65677722761158,1.21744590438802,8.17464852242519));
#49084=CARTESIAN_POINT('Ctrl Pts',(1.69699459227755,1.15853654076198,8.17079262928623));
#49085=CARTESIAN_POINT('Ctrl Pts',(1.73720397099022,1.09963887475538,8.16693750181112));
#49086=CARTESIAN_POINT('Ctrl Pts',(1.77435161589447,1.03863357366415,8.16308237433602));
#49087=CARTESIAN_POINT('Ctrl Pts',(1.80822157548012,0.975875143893002,8.15922724686091));
#49088=CARTESIAN_POINT('Ctrl Pts',(1.84209613916057,0.913108183088351,8.15537159534112));
#49089=CARTESIAN_POINT('Ctrl Pts',(1.87269190463754,0.848588049220232,8.15151594382132));
#49090=CARTESIAN_POINT('Ctrl Pts',(1.89983912488471,0.782693338452113,8.14766029230153));
#49091=CARTESIAN_POINT('Ctrl Pts',(1.92701636873427,0.716725751102979,8.14380037660489));
#49092=CARTESIAN_POINT('Ctrl Pts',(1.95073727309514,0.649381003814497,8.13994046090824));
#49093=CARTESIAN_POINT('Ctrl Pts',(1.97088081729802,0.581056250725073,8.1360805452116));
#49094=CARTESIAN_POINT('Ctrl Pts',(1.99103751614682,0.512686878479993,8.13221810881533));
#49095=CARTESIAN_POINT('Ctrl Pts',(2.00761209388234,0.443336699235825,8.12835567241907));
#49096=CARTESIAN_POINT('Ctrl Pts',(2.02053448880331,0.373413901798468,8.1244932360228));
#49097=CARTESIAN_POINT('Ctrl Pts',(2.03347837417841,0.303374819981901,8.12062437624196));
#49098=CARTESIAN_POINT('Ctrl Pts',(2.0427578967901,0.232761700841292,8.11675551646111));
#49099=CARTESIAN_POINT('Ctrl Pts',(2.04835483194737,0.161987792558138,8.11288665668027));
#49100=CARTESIAN_POINT('Ctrl Pts',(2.05006001135172,0.140425596931635,8.11170795801194));
#49101=CARTESIAN_POINT('Ctrl Pts',(2.05142374079295,0.118848470036735,8.11052925934361));
#49102=CARTESIAN_POINT('Ctrl Pts',(2.05244646447078,0.0972680470730852,
8.10935056067527));
#49103=CARTESIAN_POINT('Ctrl Pts',(2.05580355895899,0.0264302239588488,
8.10548147766828));
#49104=CARTESIAN_POINT('Ctrl Pts',(2.0554955948121,-0.0447203466931932,
8.10161239466129));
#49105=CARTESIAN_POINT('Ctrl Pts',(2.05148587354752,-0.115772505954377,
8.0977433116543));
#49106=CARTESIAN_POINT('Ctrl Pts',(2.04748212656679,-0.186718801057286,
8.09387999338719));
#49107=CARTESIAN_POINT('Ctrl Pts',(2.03978759759765,-0.257566494761722,
8.09001667512007));
#49108=CARTESIAN_POINT('Ctrl Pts',(2.0284175491114,-0.32790213319968,8.08615335685296));
#49109=CARTESIAN_POINT('Ctrl Pts',(2.01706083768672,-0.398155267966526,
8.08229457025637));
#49110=CARTESIAN_POINT('Ctrl Pts',(2.00203724775699,-0.467897063312294,
8.07843578365979));
#49111=CARTESIAN_POINT('Ctrl Pts',(1.98341388769491,-0.536718653112556,
8.0745769970632));
#49112=CARTESIAN_POINT('Ctrl Pts',(1.96480225898364,-0.605496890359343,
8.07072064121913));
#49113=CARTESIAN_POINT('Ctrl Pts',(1.94259548559621,-0.673355604291606,
8.06686428537505));
#49114=CARTESIAN_POINT('Ctrl Pts',(1.9169115576161,-0.739897048769495,8.06300792953097));
#49115=CARTESIAN_POINT('Ctrl Pts',(1.89123521692681,-0.806418836234995,
8.05915271289322));
#49116=CARTESIAN_POINT('Ctrl Pts',(1.86208393572596,-0.871623673837934,
8.05529749625548));
#49117=CARTESIAN_POINT('Ctrl Pts',(1.82962470828325,-0.93513153584906,8.05144227961773));
#49118=CARTESIAN_POINT('Ctrl Pts',(1.79716421178593,-0.998641880819646,
8.04758691225303));
#49119=CARTESIAN_POINT('Ctrl Pts',(1.76139573532314,-1.06045468691979,8.04373154488833));
#49120=CARTESIAN_POINT('Ctrl Pts',(1.72253252524606,-1.12021393580397,8.03987617752363));
#49121=CARTESIAN_POINT('Ctrl Pts',(1.68362863600564,-1.18003573629524,8.0360167746426));
#49122=CARTESIAN_POINT('Ctrl Pts',(1.64162381208422,-1.23779928058551,8.03215737176157));
#49123=CARTESIAN_POINT('Ctrl Pts',(1.59677450687319,-1.29317776685955,8.02829796888054));
#49124=CARTESIAN_POINT('Ctrl Pts',(1.5518998076435,-1.34858760885489,8.02443638077617));
#49125=CARTESIAN_POINT('Ctrl Pts',(1.50417774611702,-1.40160934328618,8.02057479267179));
#49126=CARTESIAN_POINT('Ctrl Pts',(1.45390309217126,-1.45195156981039,8.01671320456742));
#49127=CARTESIAN_POINT('Ctrl Pts',(1.40354048095847,-1.50238187182222,8.01284486047948));
#49128=CARTESIAN_POINT('Ctrl Pts',(1.35061672195277,-1.55012298092874,8.00897651639153));
#49129=CARTESIAN_POINT('Ctrl Pts',(1.2954606925744,-1.59492293120848,8.00510817230359));
#49130=CARTESIAN_POINT('Ctrl Pts',(1.26271065132406,-1.62152383479437,8.0028112624303));
#49131=CARTESIAN_POINT('Ctrl Pts',(1.22917418557495,-1.64708859639868,8.000514352557));
#49132=CARTESIAN_POINT('Ctrl Pts',(1.19492467762601,-1.67157188816407,7.99821744268371));
#49133=CARTESIAN_POINT('Ctrl Pts',(1.13723230782943,-1.71281333094543,7.99434836012647));
#49134=CARTESIAN_POINT('Ctrl Pts',(1.07728933315006,-1.75114526561477,7.99047927756924));
#49135=CARTESIAN_POINT('Ctrl Pts',(1.01542127717664,-1.7863138560614,7.986610195012));
#49136=CARTESIAN_POINT('Ctrl Pts',(0.953645401522744,-1.82143004706128,
7.98274687719491));
#49137=CARTESIAN_POINT('Ctrl Pts',(0.889950556900871,-1.8533920113503,7.97888355937782));
#49138=CARTESIAN_POINT('Ctrl Pts',(0.824692377558463,-1.88198832219995,
7.97502024156073));
#49139=CARTESIAN_POINT('Ctrl Pts',(0.759510746009658,-1.91055108959921,
7.97116145541244));
#49140=CARTESIAN_POINT('Ctrl Pts',(0.692769865048533,-1.93575585141558,
7.96730266926414));
#49141=CARTESIAN_POINT('Ctrl Pts',(0.624849634808915,-1.95743722667655,
7.96344388311585));
#49142=CARTESIAN_POINT('Ctrl Pts',(0.556972189314334,-1.97910494426719,
7.95958752771876));
#49143=CARTESIAN_POINT('Ctrl Pts',(0.487917330132223,-1.99725353132691,
7.95573117232168));
#49144=CARTESIAN_POINT('Ctrl Pts',(0.418083212371424,-2.01176638555106,
7.95187481692459));
#49145=CARTESIAN_POINT('Ctrl Pts',(0.348269724278994,-2.02627495253885,
7.94801960073188));
#49146=CARTESIAN_POINT('Ctrl Pts',(0.277677909981633,-2.03714982015024,
7.94416438453917));
#49147=CARTESIAN_POINT('Ctrl Pts',(0.206717615993114,-2.04432516732004,
7.94030916834647));
#49148=CARTESIAN_POINT('Ctrl Pts',(0.135754547630296,-2.0515007950284,7.93645380142422));
#49149=CARTESIAN_POINT('Ctrl Pts',(0.0644234545139279,-2.05497656844665,
7.93259843450196));
#49150=CARTESIAN_POINT('Ctrl Pts',(-0.00686090002047612,-2.05473854554561,
7.92874306757971));
#49151=CARTESIAN_POINT('Ctrl Pts',(-0.0782198699361268,-2.05450027349917,
7.92488366513417));
#49152=CARTESIAN_POINT('Ctrl Pts',(-0.149531516833611,-2.05054044676251,
7.92102426268864));
#49153=CARTESIAN_POINT('Ctrl Pts',(-0.220382188502956,-2.04289726944128,
7.9171648602431));
#49154=CARTESIAN_POINT('Ctrl Pts',(-0.291272976427429,-2.03524976448781,
7.91330327257095));
#49155=CARTESIAN_POINT('Ctrl Pts',(-0.361701789698669,-2.02391483449982,
7.9094416848988));
#49156=CARTESIAN_POINT('Ctrl Pts',(-0.431263935949848,-2.00898207559178,
7.90558009722665));
#49157=CARTESIAN_POINT('Ctrl Pts',(-0.500947783801651,-1.99402319125835,
7.90171175356111));
#49158=CARTESIAN_POINT('Ctrl Pts',(-0.569761468208529,-1.97545403738304,
7.89784340989556));
#49159=CARTESIAN_POINT('Ctrl Pts',(-0.637314927708768,-1.95341425340852,
7.89397506623002));
#49160=CARTESIAN_POINT('Ctrl Pts',(-0.677426275066602,-1.94032764855906,
7.89167815238407));
#49161=CARTESIAN_POINT('Ctrl Pts',(-0.717093664948321,-1.92601835521994,
7.88938123853811));
#49162=CARTESIAN_POINT('Ctrl Pts',(-0.756239214398889,-1.91052343955926,
7.88708432469216));
#49163=CARTESIAN_POINT('Ctrl Pts',(-0.822178724847217,-1.88442271629842,
7.8832152418291));
#49164=CARTESIAN_POINT('Ctrl Pts',(-0.886894544863902,-1.85485312506099,
7.87934615896604));
#49165=CARTESIAN_POINT('Ctrl Pts',(-0.949996860707018,-1.8219504732969,
7.87547707610299));
#49166=CARTESIAN_POINT('Ctrl Pts',(-1.01300515719984,-1.78909684486739,
7.8716137579833));
#49167=CARTESIAN_POINT('Ctrl Pts',(-1.07440429424018,-1.75292023624344,
7.86775043986362));
#49168=CARTESIAN_POINT('Ctrl Pts',(-1.13382375618332,-1.71360475384913,
7.86388712174393));
#49169=CARTESIAN_POINT('Ctrl Pts',(-1.19317351905456,-1.67433538854415,
7.8600283352992));
#49170=CARTESIAN_POINT('Ctrl Pts',(-1.25054781626174,-1.63193472972845,
7.85616954885447));
#49171=CARTESIAN_POINT('Ctrl Pts',(-1.30560165538449,-1.58663224471119,
7.85231076240974));
#49172=CARTESIAN_POINT('Ctrl Pts',(-1.36062081458777,-1.54135829696867,
7.84845440672016));
#49173=CARTESIAN_POINT('Ctrl Pts',(-1.41332204151208,-1.4931864575685,7.84459805103058));
#49174=CARTESIAN_POINT('Ctrl Pts',(-1.46339142316949,-1.44238798701805,
7.840741695341));
#49175=CARTESIAN_POINT('Ctrl Pts',(-1.51344601379599,-1.39160452287917,
7.83688647886014));
#49176=CARTESIAN_POINT('Ctrl Pts',(-1.56086996183677,-1.33819631382218,
7.83303126237929));
#49177=CARTESIAN_POINT('Ctrl Pts',(-1.60538567611349,-1.28247198543657,
7.82917604589843));
#49178=CARTESIAN_POINT('Ctrl Pts',(-1.64990313079121,-1.2267454784343,7.82532067869276));
#49179=CARTESIAN_POINT('Ctrl Pts',(-1.69151182448562,-1.16870305324428,
7.8214653114871));
#49180=CARTESIAN_POINT('Ctrl Pts',(-1.72997508452341,-1.10868560441101,
7.81760994428143));
#49181=CARTESIAN_POINT('Ctrl Pts',(-1.7684786050665,-1.04860533373648,7.81375054156157));
#49182=CARTESIAN_POINT('Ctrl Pts',(-1.80382985691664,-0.986546322444212,
7.8098911388417));
#49183=CARTESIAN_POINT('Ctrl Pts',(-1.8358365797444,-0.922876814624989,
7.80603173612184));
#49184=CARTESIAN_POINT('Ctrl Pts',(-1.86786142501153,-0.859171256667153,
7.80217014818007));
#49185=CARTESIAN_POINT('Ctrl Pts',(-1.89653777611546,-0.793853831934715,
7.79830856023831));
#49186=CARTESIAN_POINT('Ctrl Pts',(-1.92172140849375,-0.727313131076846,
7.79444697229655));
#49187=CARTESIAN_POINT('Ctrl Pts',(-1.94694910051717,-0.6606560149369,7.7905786283717));
#49188=CARTESIAN_POINT('Ctrl Pts',(-1.96867172566271,-0.59277181259146,
7.78671028444685));
#49189=CARTESIAN_POINT('Ctrl Pts',(-1.98679503793688,-0.524063965303268,
7.782841940522));
#49190=CARTESIAN_POINT('Ctrl Pts',(-1.99755613909279,-0.483267223312214,
7.7805450292482));
#49191=CARTESIAN_POINT('Ctrl Pts',(-2.00704922822886,-0.44218030315848,
7.7782481179744));
#49192=CARTESIAN_POINT('Ctrl Pts',(-2.01526320370241,-0.400888740554147,
7.7759512067006));
#49193=CARTESIAN_POINT('Ctrl Pts',(-2.03523538600266,-0.300488804073767,
7.77036629463998));
#49194=CARTESIAN_POINT('Ctrl Pts',(-2.04770968318372,-0.198551497556471,
7.76478138257937));
#49195=CARTESIAN_POINT('Ctrl Pts',(-2.05250622663751,-0.0959987089196925,
7.75919647051875));
#49196=CARTESIAN_POINT('Ctrl Pts',(-2.05397248079007,-0.0646493729564441,
7.75748922016661));
#49197=CARTESIAN_POINT('Ctrl Pts',(-2.05472158081271,-0.0332427087908737,
7.75578196981447));
#49198=CARTESIAN_POINT('Ctrl Pts',(-2.05474920663131,-0.0018056433735876,
7.75407471946232));
#49199=CARTESIAN_POINT('Origin',(0.,0.,18.5459252805377));
#49200=CARTESIAN_POINT('',(1.25206542099588,1.62921138715834,8.90613916330362));
#49201=CARTESIAN_POINT('',(1.25051812704728,1.62722676461094,8.84785675763342));
#49202=CARTESIAN_POINT('',(1.25206542099588,1.62921138715835,18.5459252805377));
#49203=CARTESIAN_POINT('',(-2.05451192518334,-0.000653016369823574,8.39592531845778));
#49204=CARTESIAN_POINT('Ctrl Pts',(1.25051812704735,1.62722676461089,8.84785675763342));
#49205=CARTESIAN_POINT('Ctrl Pts',(1.58873501929067,1.36387014211555,8.82468048835194));
#49206=CARTESIAN_POINT('Ctrl Pts',(2.26673114618394,0.412739085322609,8.76445984640662));
#49207=CARTESIAN_POINT('Ctrl Pts',(1.84698007748907,-1.57690952787191,8.6671948317974));
#49208=CARTESIAN_POINT('Ctrl Pts',(-0.323048206860337,-2.40699375331995,
8.55606171380587));
#49209=CARTESIAN_POINT('Ctrl Pts',(-1.84811520434371,-1.28994634362903,
8.46563869868007));
#49210=CARTESIAN_POINT('Ctrl Pts',(-2.05243358460716,-0.303009497723999,
8.41226005621812));
#49211=CARTESIAN_POINT('Ctrl Pts',(-2.05157518345028,-0.000660745958733733,
8.39592578642004));
#49212=CARTESIAN_POINT('Ctrl Pts',(-2.05474989643199,-0.000652390022636229,
8.39592528053767));
#49213=CARTESIAN_POINT('Ctrl Pts',(-2.05477316158455,0.0726229026154983,
8.3919727248606));
#49214=CARTESIAN_POINT('Ctrl Pts',(-2.05087243556388,0.145865091084949,
8.38802016918352));
#49215=CARTESIAN_POINT('Ctrl Pts',(-2.04308448283436,0.218639791669856,
8.38406761350645));
#49216=CARTESIAN_POINT('Ctrl Pts',(-2.03529044046684,0.291471397015037,
8.38011196720542));
#49217=CARTESIAN_POINT('Ctrl Pts',(-2.02360317415942,0.3638343400088,8.37615632090438));
#49218=CARTESIAN_POINT('Ctrl Pts',(-2.00811093276723,0.43530224465388,8.37220067460335));
#49219=CARTESIAN_POINT('Ctrl Pts',(-1.99259007572178,0.506902157362047,
8.36823772184484));
#49220=CARTESIAN_POINT('Ctrl Pts',(-1.97325031090492,0.577603291101814,
8.36427476908632));
#49221=CARTESIAN_POINT('Ctrl Pts',(-1.95023029805764,0.646992540171847,
8.36031181632781));
#49222=CARTESIAN_POINT('Ctrl Pts',(-1.92718562648172,0.716456118073708,
8.35634461850752));
#49223=CARTESIAN_POINT('Ctrl Pts',(-1.90045301963665,0.784604594021689,
8.35237742068722));
#49224=CARTESIAN_POINT('Ctrl Pts',(-1.87021901282319,0.851045478558368,
8.34841022286693));
#49225=CARTESIAN_POINT('Ctrl Pts',(-1.83992267930305,0.917623329443823,
8.34443484675996));
#49226=CARTESIAN_POINT('Ctrl Pts',(-1.80611074383731,0.982486162956809,
8.34045947065301));
#49227=CARTESIAN_POINT('Ctrl Pts',(-1.76901511959829,1.04526698461811,8.33648409454604));
#49228=CARTESIAN_POINT('Ctrl Pts',(-1.76065231207126,1.05942024227889,8.33558788897161));
#49229=CARTESIAN_POINT('Ctrl Pts',(-1.75212278665681,1.0734678111016,8.33469168339718));
#49230=CARTESIAN_POINT('Ctrl Pts',(-1.74342948855721,1.0874057112822,8.33379547782275));
#49231=CARTESIAN_POINT('Ctrl Pts',(-1.70589893428835,1.14757816978168,8.32992639481628));
#49232=CARTESIAN_POINT('Ctrl Pts',(-1.66517604049293,1.20592321640611,8.32605731180981));
#49233=CARTESIAN_POINT('Ctrl Pts',(-1.62146448556,1.26208180581436,8.32218822880335));
#49234=CARTESIAN_POINT('Ctrl Pts',(-1.57781805865443,1.31815672173736,8.31832491053676));
#49235=CARTESIAN_POINT('Ctrl Pts',(-1.53119210555474,1.3720512666889,8.31446159227018));
#49236=CARTESIAN_POINT('Ctrl Pts',(-1.48183434704247,1.42343406254916,8.31059827400359));
#49237=CARTESIAN_POINT('Ctrl Pts',(-1.43253448515796,1.4747565864138,8.30673948740754));
#49238=CARTESIAN_POINT('Ctrl Pts',(-1.38050951779156,1.52357286486347,8.30288070081147));
#49239=CARTESIAN_POINT('Ctrl Pts',(-1.32604719870036,1.56958478245647,8.29902191421542));
#49240=CARTESIAN_POINT('Ctrl Pts',(-1.27161918687533,1.6155677159164,8.29516555837187));
#49241=CARTESIAN_POINT('Ctrl Pts',(-1.21475723964478,1.65874948054823,8.29130920252832));
#49242=CARTESIAN_POINT('Ctrl Pts',(-1.15578463524892,1.69887004783254,8.28745284668477));
#49243=CARTESIAN_POINT('Ctrl Pts',(-1.0968294519539,1.73897876309748,8.28359763004755));
#49244=CARTESIAN_POINT('Ctrl Pts',(-1.03576525076006,1.77602780321708,8.27974241341033));
#49245=CARTESIAN_POINT('Ctrl Pts',(-0.972945535912756,1.80979958742603,
8.27588719677311));
#49246=CARTESIAN_POINT('Ctrl Pts',(-0.91012336501046,1.84357269200645,8.27203182940893));
#49247=CARTESIAN_POINT('Ctrl Pts',(-0.845545973103761,1.87406805820691,
8.26817646204476));
#49248=CARTESIAN_POINT('Ctrl Pts',(-0.779591250925281,1.90111415858721,
8.26432109468059));
#49249=CARTESIAN_POINT('Ctrl Pts',(-0.713567492171636,1.92818856884556,
8.26046169180008));
#49250=CARTESIAN_POINT('Ctrl Pts',(-0.646163975594236,1.95180632135027,
8.25660228891957));
#49251=CARTESIAN_POINT('Ctrl Pts',(-0.577777511014386,1.97184449444322,
8.25274288603907));
#49252=CARTESIAN_POINT('Ctrl Pts',(-0.509352325496681,1.9918940133026,8.24888129793521));
#49253=CARTESIAN_POINT('Ctrl Pts',(-0.439943556940449,2.00835980586299,
8.24501970983135));
#49254=CARTESIAN_POINT('Ctrl Pts',(-0.369959393931269,2.02116986157572,
8.2411581217275));
#49255=CARTESIAN_POINT('Ctrl Pts',(-0.299852791178743,2.03400232892939,
8.23728977764006));
#49256=CARTESIAN_POINT('Ctrl Pts',(-0.229169266026279,2.04316622748358,
8.23342143355262));
#49257=CARTESIAN_POINT('Ctrl Pts',(-0.158322630141146,2.04864138083882,
8.22955308946518));
#49258=CARTESIAN_POINT('Ctrl Pts',(-0.116255964376895,2.05189236718878,
8.22725617958718));
#49259=CARTESIAN_POINT('Ctrl Pts',(-0.0741318222005703,2.05384383432988,
8.22495926970918));
#49260=CARTESIAN_POINT('Ctrl Pts',(-0.0320363413327623,2.05450023979897,
8.22266235983118));
#49261=CARTESIAN_POINT('Ctrl Pts',(0.0388583812382214,2.0556057191204,8.21879403987821));
#49262=CARTESIAN_POINT('Ctrl Pts',(0.109949219424514,2.05303950652832,8.21492571992523));
#49263=CARTESIAN_POINT('Ctrl Pts',(0.180824300462245,2.04677798865982,8.21105739997225));
#49264=CARTESIAN_POINT('Ctrl Pts',(0.251600846644332,2.04052517593493,8.20719445799334));
#49265=CARTESIAN_POINT('Ctrl Pts',(0.322161751218005,2.03058729266115,8.20333151601444));
#49266=CARTESIAN_POINT('Ctrl Pts',(0.392094373796085,2.01699270314433,8.19946857403553));
#49267=CARTESIAN_POINT('Ctrl Pts',(0.461953175883252,2.00341246400126,8.19560970975688));
#49268=CARTESIAN_POINT('Ctrl Pts',(0.53118453789183,1.98618327218889,8.19175084547824));
#49269=CARTESIAN_POINT('Ctrl Pts',(0.599381904191762,1.96538517737045,8.18789198119959));
#49270=CARTESIAN_POINT('Ctrl Pts',(0.667536212769918,1.94460021383007,8.18403555328929));
#49271=CARTESIAN_POINT('Ctrl Pts',(0.734657357271598,1.92025095925107,8.18017912537899));
#49272=CARTESIAN_POINT('Ctrl Pts',(0.800351513123296,1.89246797012294,8.17632269746868));
#49273=CARTESIAN_POINT('Ctrl Pts',(0.866021363619131,1.86469526007411,8.17246769634972));
#49274=CARTESIAN_POINT('Ctrl Pts',(0.930264828230893,1.83349153086389,8.16861269523076));
#49275=CARTESIAN_POINT('Ctrl Pts',(0.992707432808873,1.79903571819628,8.1647576941118));
#49276=CARTESIAN_POINT('Ctrl Pts',(1.05516574029779,1.76457124066658,8.16090172354674));
#49277=CARTESIAN_POINT('Ctrl Pts',(1.11582185755692,1.72685328081183,8.15704575298169));
#49278=CARTESIAN_POINT('Ctrl Pts',(1.17432654764215,1.6861063792071,8.15318978241663));
#49279=CARTESIAN_POINT('Ctrl Pts',(1.20068582122837,1.66774787281,8.15145247583631));
#49280=CARTESIAN_POINT('Ctrl Pts',(1.22660874853696,1.64877509728869,8.14971516925599));
#49281=CARTESIAN_POINT('Ctrl Pts',(1.25206542099587,1.62921138715835,8.14797786267567));
#49282=CARTESIAN_POINT('',(-2.05474966036672,0.00118140715606992,8.45407471951265));
#49283=CARTESIAN_POINT('Ctrl Pts',(-2.05474966036618,0.0011814080800246,
8.45407471946232));
#49284=CARTESIAN_POINT('Ctrl Pts',(-2.05470981683469,0.0704787865199796,
8.45029978452486));
#49285=CARTESIAN_POINT('Ctrl Pts',(-2.05116461443229,0.139673811090078,
8.4465248495874));
#49286=CARTESIAN_POINT('Ctrl Pts',(-2.04414330436285,0.208508306137984,
8.44274991464995));
#49287=CARTESIAN_POINT('Ctrl Pts',(-2.03694688085526,0.279059552756773,
8.43888083177868));
#49288=CARTESIAN_POINT('Ctrl Pts',(-2.02607958224214,0.349375980540898,
8.4350117489074));
#49289=CARTESIAN_POINT('Ctrl Pts',(-2.01156615579492,0.419045538528258,
8.43114266603613));
#49290=CARTESIAN_POINT('Ctrl Pts',(-1.9970743536289,0.488611292350709,8.42727934790527));
#49291=CARTESIAN_POINT('Ctrl Pts',(-1.97894730535087,0.557531617800781,
8.42341602977442));
#49292=CARTESIAN_POINT('Ctrl Pts',(-1.95726148410381,0.625399908333671,
8.41955271164356));
#49293=CARTESIAN_POINT('Ctrl Pts',(-1.93560110031659,0.693188589388313,
8.41569392518335));
#49294=CARTESIAN_POINT('Ctrl Pts',(-1.91039038254942,0.759927226251012,
8.41183513872315));
#49295=CARTESIAN_POINT('Ctrl Pts',(-1.88175639426221,0.825221446130244,
8.40797635226295));
#49296=CARTESIAN_POINT('Ctrl Pts',(-1.853140443288,0.890474535438722,8.40411999655527));
#49297=CARTESIAN_POINT('Ctrl Pts',(-1.82110569471359,0.954284569112658,
8.40026364084759));
#49298=CARTESIAN_POINT('Ctrl Pts',(-1.78582787905737,1.01627572483133,8.3964072851399));
#49299=CARTESIAN_POINT('Ctrl Pts',(-1.75056048482158,1.0782485677411,8.39255206863836));
#49300=CARTESIAN_POINT('Ctrl Pts',(-1.71205216560505,1.13840317743994,8.38869685213682));
#49301=CARTESIAN_POINT('Ctrl Pts',(-1.67052448239039,1.19638853063472,8.38484163563528));
#49302=CARTESIAN_POINT('Ctrl Pts',(-1.62899517556853,1.25437615088198,8.38098626840639));
#49303=CARTESIAN_POINT('Ctrl Pts',(-1.58444655502027,1.31019395258132,8.37713090117751));
#49304=CARTESIAN_POINT('Ctrl Pts',(-1.53714235724309,1.36352152020756,8.37327553394862));
#49305=CARTESIAN_POINT('Ctrl Pts',(-1.48978864487407,1.41690490725088,8.36941613120188));
#49306=CARTESIAN_POINT('Ctrl Pts',(-1.43967392051527,1.4677924927167,8.36555672845514));
#49307=CARTESIAN_POINT('Ctrl Pts',(-1.38710031154951,1.51589916821642,8.3616973257084));
#49308=CARTESIAN_POINT('Ctrl Pts',(-1.3344969349954,1.56403308209186,8.35783573773766));
#49309=CARTESIAN_POINT('Ctrl Pts',(-1.27943227747534,1.6093826425411,8.35397414976692));
#49310=CARTESIAN_POINT('Ctrl Pts',(-1.22224110270172,1.65170343868579,8.35011256179617));
#49311=CARTESIAN_POINT('Ctrl Pts',(-1.16494986992548,1.69409827657467,8.34624421783937));
#49312=CARTESIAN_POINT('Ctrl Pts',(-1.10552509712036,1.73345350237821,8.34237587388257));
#49313=CARTESIAN_POINT('Ctrl Pts',(-1.04432942330775,1.76956876614437,8.33850752992577));
#49314=CARTESIAN_POINT('Ctrl Pts',(-1.00799319691305,1.79101296830366,8.33621061883665));
#49315=CARTESIAN_POINT('Ctrl Pts',(-0.971033081498362,1.81131575915701,
8.33391370774752));
#49316=CARTESIAN_POINT('Ctrl Pts',(-0.933528375546205,1.83044320713593,
8.33161679665839));
#49317=CARTESIAN_POINT('Ctrl Pts',(-0.870352742076924,1.86266286096445,
8.3277477138488));
#49318=CARTESIAN_POINT('Ctrl Pts',(-0.805383377294136,1.89167113018795,
8.3238786310392));
#49319=CARTESIAN_POINT('Ctrl Pts',(-0.738979881261259,1.91726531747463,
8.32000954822961));
#49320=CARTESIAN_POINT('Ctrl Pts',(-0.672675323125341,1.94282137069887,
8.31614623016042));
#49321=CARTESIAN_POINT('Ctrl Pts',(-0.604941324782959,1.96497326588098,
8.31228291209123));
#49322=CARTESIAN_POINT('Ctrl Pts',(-0.536160967358015,1.98356471524922,
8.30841959402204));
#49323=CARTESIAN_POINT('Ctrl Pts',(-0.467461289261398,2.00213435685571,
8.3045608076232));
#49324=CARTESIAN_POINT('Ctrl Pts',(-0.397718156749575,2.01715172225172,
8.30070202122437));
#49325=CARTESIAN_POINT('Ctrl Pts',(-0.327331812158638,2.02850966161094,
8.29684323482554));
#49326=CARTESIAN_POINT('Ctrl Pts',(-0.256989805800319,2.03986044630174,
8.292986879179));
#49327=CARTESIAN_POINT('Ctrl Pts',(-0.186005869672279,2.04755630117204,
8.28913052353247));
#49328=CARTESIAN_POINT('Ctrl Pts',(-0.114791057301673,2.05154102461139,
8.28527416788593));
#49329=CARTESIAN_POINT('Ctrl Pts',(-0.0435972824952619,2.05552457092379,
8.28141895144523));
#49330=CARTESIAN_POINT('Ctrl Pts',(0.0278267483912949,2.05579913515123,
8.27756373500453));
#49331=CARTESIAN_POINT('Ctrl Pts',(0.0990659587721552,2.05236046987671,
8.27370851856382));
#49332=CARTESIAN_POINT('Ctrl Pts',(0.170307954398715,2.0489216701604,8.26985315139538));
#49333=CARTESIAN_POINT('Ctrl Pts',(0.241364630061478,2.04176937833479,8.26599778422694));
#49334=CARTESIAN_POINT('Ctrl Pts',(0.311823748603643,2.03095138107902,8.2621424170585));
#49335=CARTESIAN_POINT('Ctrl Pts',(0.382356618643337,2.02012206032794,8.25828301437119));
#49336=CARTESIAN_POINT('Ctrl Pts',(0.452290201824877,2.00561944851768,8.25442361168388));
#49337=CARTESIAN_POINT('Ctrl Pts',(0.521221101224195,1.98754273567605,8.25056420899658));
#49338=CARTESIAN_POINT('Ctrl Pts',(0.590191029846752,1.9694557876559,8.24670262108478));
#49339=CARTESIAN_POINT('Ctrl Pts',(0.658156681460076,1.94779085767811,8.24284103317299));
#49340=CARTESIAN_POINT('Ctrl Pts',(0.724731149162215,1.92269662815901,8.2389794452612));
#49341=CARTESIAN_POINT('Ctrl Pts',(0.791422091298898,1.89755849537947,8.23511110136196));
#49342=CARTESIAN_POINT('Ctrl Pts',(0.85671654495917,1.86897927936765,8.23124275746271));
#49343=CARTESIAN_POINT('Ctrl Pts',(0.920249501264119,1.83715497928812,8.22737441356347));
#49344=CARTESIAN_POINT('Ctrl Pts',(0.957973548082761,1.81825862287731,8.22507750193125));
#49345=CARTESIAN_POINT('Ctrl Pts',(0.995077042346118,1.79821903709245,8.22278059029904));
#49346=CARTESIAN_POINT('Ctrl Pts',(1.03148846703391,1.77708443943332,8.22048367866683));
#49347=CARTESIAN_POINT('Ctrl Pts',(1.09282082805986,1.74148476749291,8.21661470032612));
#49348=CARTESIAN_POINT('Ctrl Pts',(1.15242817648098,1.70263650639596,8.21274572198541));
#49349=CARTESIAN_POINT('Ctrl Pts',(1.20994520886422,1.66073181280017,8.20887674364469));
#49350=CARTESIAN_POINT('Ctrl Pts',(1.22411376771944,1.65040914674942,8.20792367209252));
#49351=CARTESIAN_POINT('Ctrl Pts',(1.23815558639144,1.63990123566865,8.20697060054034));
#49352=CARTESIAN_POINT('Ctrl Pts',(1.25206542099588,1.62921138715834,8.20601752898817));
#49353=CARTESIAN_POINT('Ctrl Pts',(1.25206542099588,1.62921138715834,8.90613916330362));
#49354=CARTESIAN_POINT('Ctrl Pts',(1.30858031424556,1.58577912037765,8.90227086778885));
#49355=CARTESIAN_POINT('Ctrl Pts',(1.36275963984382,1.53945896042727,8.89840257227408));
#49356=CARTESIAN_POINT('Ctrl Pts',(1.41431082657472,1.49054434631565,8.89453427675932));
#49357=CARTESIAN_POINT('Ctrl Pts',(1.44652514779997,1.45997761853446,8.89211698004494));
#49358=CARTESIAN_POINT('Ctrl Pts',(1.47771392678912,1.42839848807823,8.88969968333056));
#49359=CARTESIAN_POINT('Ctrl Pts',(1.50781381874179,1.39588504201144,8.88728238661619));
#49360=CARTESIAN_POINT('Ctrl Pts',(1.55599117939921,1.34384458884843,8.88341330377005));
#49361=CARTESIAN_POINT('Ctrl Pts',(1.60156556405218,1.289205101346,8.87954422092392));
#49362=CARTESIAN_POINT('Ctrl Pts',(1.64424416955661,1.23225755156099,8.87567513807778));
#49363=CARTESIAN_POINT('Ctrl Pts',(1.68685918606722,1.17539485078519,8.87181181997214));
#49364=CARTESIAN_POINT('Ctrl Pts',(1.72658669876803,1.11623129940836,8.8679485018665));
#49365=CARTESIAN_POINT('Ctrl Pts',(1.76317218510371,1.05509308033775,8.86408518376085));
#49366=CARTESIAN_POINT('Ctrl Pts',(1.79971475667791,0.994026576374739,8.86022639732587));
#49367=CARTESIAN_POINT('Ctrl Pts',(1.83312237449395,0.930990420468526,8.85636761089089));
#49368=CARTESIAN_POINT('Ctrl Pts',(1.86318313994246,0.866340665982001,8.85250882445591));
#49369=CARTESIAN_POINT('Ctrl Pts',(1.89322496931296,0.801731636100334,8.84865246877344));
#49370=CARTESIAN_POINT('Ctrl Pts',(1.91992392475803,0.73551146370853,8.84479611309096));
#49371=CARTESIAN_POINT('Ctrl Pts',(1.94311419961833,0.668060453657902,8.84093975740849));
#49372=CARTESIAN_POINT('Ctrl Pts',(1.9662976238392,0.60062936931113,8.8370845409321));
#49373=CARTESIAN_POINT('Ctrl Pts',(1.98597426735778,0.531968628295968,8.83322932445571));
#49374=CARTESIAN_POINT('Ctrl Pts',(2.00202722852745,0.462476527766211,8.82937410797933));
#49375=CARTESIAN_POINT('Ctrl Pts',(2.01808081731988,0.392981710303225,8.82551874077551));
#49376=CARTESIAN_POINT('Ctrl Pts',(2.03051033529391,0.322655942608069,8.82166337357169));
#49377=CARTESIAN_POINT('Ctrl Pts',(2.03924972787343,0.251908931695832,8.81780800636788));
#49378=CARTESIAN_POINT('Ctrl Pts',(2.04799826821387,0.181087867954917,8.8139486036459));
#49379=CARTESIAN_POINT('Ctrl Pts',(2.05304891295617,0.109845163914514,8.81008920092393));
#49380=CARTESIAN_POINT('Ctrl Pts',(2.05438747855597,0.0385959901084021,
8.80622979820195));
#49381=CARTESIAN_POINT('Ctrl Pts',(2.05572680206213,-0.0326935255395951,
8.80236821025584));
#49382=CARTESIAN_POINT('Ctrl Pts',(2.05334987856776,-0.103989032502454,
8.79850662230973));
#49383=CARTESIAN_POINT('Ctrl Pts',(2.04729463568034,-0.174877777932225,
8.79464503436362));
#49384=CARTESIAN_POINT('Ctrl Pts',(2.04122879892843,-0.245890545763207,
8.79077669043098));
#49385=CARTESIAN_POINT('Ctrl Pts',(2.03147186094257,-0.316494649881803,
8.78690834649833));
#49386=CARTESIAN_POINT('Ctrl Pts',(2.0181132365875,-0.386285550869183,8.78304000256569));
#49387=CARTESIAN_POINT('Ctrl Pts',(2.01018126984653,-0.427725379607586,
8.780743091252));
#49388=CARTESIAN_POINT('Ctrl Pts',(2.00098044883844,-0.468878735330665,
8.77844617993832));
#49389=CARTESIAN_POINT('Ctrl Pts',(1.99053773827548,-0.509663688132791,
8.77614926862464));
#49390=CARTESIAN_POINT('Ctrl Pts',(1.9729472844728,-0.578364800146326,8.7722801857741));
#49391=CARTESIAN_POINT('Ctrl Pts',(1.95176149298502,-0.6462887309913,8.76841110292356));
#49392=CARTESIAN_POINT('Ctrl Pts',(1.92706600839946,-0.713031669543074,
8.76454202007303));
#49393=CARTESIAN_POINT('Ctrl Pts',(1.90240731885422,-0.779675164445281,
8.76067870196297));
#49394=CARTESIAN_POINT('Ctrl Pts',(1.87424948336426,-0.845140707965953,
8.75681538385291));
#49395=CARTESIAN_POINT('Ctrl Pts',(1.84272849095502,-0.909037552097063,
8.75295206574285));
#49396=CARTESIAN_POINT('Ctrl Pts',(1.81124447265776,-0.97285944525458,8.74909327930345));
#49397=CARTESIAN_POINT('Ctrl Pts',(1.77640534738202,-1.0351158605092,8.74523449286404));
#49398=CARTESIAN_POINT('Ctrl Pts',(1.73839531770047,-1.09543565849258,8.74137570642464));
#49399=CARTESIAN_POINT('Ctrl Pts',(1.7004092315505,-1.15571745942624,8.73751935073774));
#49400=CARTESIAN_POINT('Ctrl Pts',(1.65925646224923,-1.21406465338534,8.73366299505084));
#49401=CARTESIAN_POINT('Ctrl Pts',(1.61516658621353,-1.27013167084335,8.72980663936394));
#49402=CARTESIAN_POINT('Ctrl Pts',(1.57108973476881,-1.32618212554286,8.72595142288314));
#49403=CARTESIAN_POINT('Ctrl Pts',(1.52407779923766,-1.37995335934943,8.72209620640234));
#49404=CARTESIAN_POINT('Ctrl Pts',(1.47440199708189,-1.43113113078465,8.71824098992154));
#49405=CARTESIAN_POINT('Ctrl Pts',(1.42472425275104,-1.48231090311744,8.71438562271332));
#49406=CARTESIAN_POINT('Ctrl Pts',(1.37238277494907,-1.53089666472608,8.71053025550509));
#49407=CARTESIAN_POINT('Ctrl Pts',(1.31768594539002,-1.57661070395377,8.70667488829687));
#49408=CARTESIAN_POINT('Ctrl Pts',(1.26293186316627,-1.6223725933143,8.70281548557055));
#49409=CARTESIAN_POINT('Ctrl Pts',(1.2058178811779,-1.66525644765854,8.69895608284422));
#49410=CARTESIAN_POINT('Ctrl Pts',(1.14668510504853,-1.70502517059422,8.69509668011789));
#49411=CARTESIAN_POINT('Ctrl Pts',(1.08751884747718,-1.74481641089297,8.69123509216745));
#49412=CARTESIAN_POINT('Ctrl Pts',(1.02633193716306,-1.78148875872548,8.687373504217));
#49413=CARTESIAN_POINT('Ctrl Pts',(0.963491712615178,-1.81485020930706,
8.68351191626656));
#49414=CARTESIAN_POINT('Ctrl Pts',(0.900541546843314,-1.84827002694154,
8.67964357232966));
#49415=CARTESIAN_POINT('Ctrl Pts',(0.835932732302552,-1.87836717717327,
8.67577522839276));
#49416=CARTESIAN_POINT('Ctrl Pts',(0.770053632803515,-1.90499736616776,
8.67190688445586));
#49417=CARTESIAN_POINT('Ctrl Pts',(0.730936519939146,-1.92080960580702,
8.6696099731816));
#49418=CARTESIAN_POINT('Ctrl Pts',(0.691371880962958,-1.93540046172162,
8.66731306190733));
#49419=CARTESIAN_POINT('Ctrl Pts',(0.651443173023543,-1.94874815069085,
8.66501615063306));
#49420=CARTESIAN_POINT('Ctrl Pts',(0.584184380516407,-1.97123195968846,
8.66114706779078));
#49421=CARTESIAN_POINT('Ctrl Pts',(0.515628483213545,-1.9902736788152,8.65727798494849));
#49422=CARTESIAN_POINT('Ctrl Pts',(0.446161188134982,-2.00572624171445,
8.6534089021062));
#49423=CARTESIAN_POINT('Ctrl Pts',(0.37679739586139,-2.02115578106568,8.64954558400438));
#49424=CARTESIAN_POINT('Ctrl Pts',(0.306525371609875,-2.0330066745322,8.64568226590255));
#49425=CARTESIAN_POINT('Ctrl Pts',(0.235747153476675,-2.04118123696247,
8.64181894780073));
#49426=CARTESIAN_POINT('Ctrl Pts',(0.165051958165386,-2.04934621063424,
8.63796016136951));
#49427=CARTESIAN_POINT('Ctrl Pts',(0.0938522286243621,-2.05384336356217,
8.63410137493829));
#49428=CARTESIAN_POINT('Ctrl Pts',(0.0225596791623202,-2.05462615173079,
8.63024258850707));
#49429=CARTESIAN_POINT('Ctrl Pts',(-0.0486879612217034,-2.05540844680028,
8.62638623282832));
#49430=CARTESIAN_POINT('Ctrl Pts',(-0.120027820918118,-2.0524810138713,
8.62252987714958));
#49431=CARTESIAN_POINT('Ctrl Pts',(-0.191045057807914,-2.04584929757477,
8.61867352147083));
#49432=CARTESIAN_POINT('Ctrl Pts',(-0.262041315495508,-2.03921954035357,
8.61481830499813));
#49433=CARTESIAN_POINT('Ctrl Pts',(-0.332714656170015,-2.02888771736128,
8.61096308852544));
#49434=CARTESIAN_POINT('Ctrl Pts',(-0.402653972158619,-2.0149112489648,
8.60710787205273));
#49435=CARTESIAN_POINT('Ctrl Pts',(-0.472596022566016,-2.00093423413006,
8.60325250485256));
#49436=CARTESIAN_POINT('Ctrl Pts',(-0.541803515378322,-1.98331238834194,
8.59939713765239));
#49437=CARTESIAN_POINT('Ctrl Pts',(-0.609875875675157,-1.96215416794131,
8.59554177045221));
#49438=CARTESIAN_POINT('Ctrl Pts',(-0.678019489172598,-1.94097380065293,
8.59168236773379));
#49439=CARTESIAN_POINT('Ctrl Pts',(-0.745025133450511,-1.91624981397103,
8.58782296501536));
#49440=CARTESIAN_POINT('Ctrl Pts',(-0.810508607011173,-1.88814018559555,
8.58396356229694));
#49441=CARTESIAN_POINT('Ctrl Pts',(-0.876029157829791,-1.86001464132732,
8.58010197435432));
#49442=CARTESIAN_POINT('Ctrl Pts',(-0.940025386211164,-1.82849985396889,
8.57624038641171));
#49443=CARTESIAN_POINT('Ctrl Pts',(-1.0021367454079,-1.79380029713546,8.5723787984691));
#49444=CARTESIAN_POINT('Ctrl Pts',(-1.06435677065593,-1.75904003218243,
8.56851045453984));
#49445=CARTESIAN_POINT('Ctrl Pts',(-1.12468493157216,-1.72108413213595,
8.56464211061058));
#49446=CARTESIAN_POINT('Ctrl Pts',(-1.18278936124687,-1.680180612143,8.56077376668132));
#49447=CARTESIAN_POINT('Ctrl Pts',(-1.21729010012848,-1.65589327862099,
8.55847685533471));
#49448=CARTESIAN_POINT('Ctrl Pts',(-1.25100744344955,-1.63056750904801,
8.55617994398811));
#49449=CARTESIAN_POINT('Ctrl Pts',(-1.28387782488486,-1.60426160375075,
8.55388303264151));
#49450=CARTESIAN_POINT('Ctrl Pts',(-1.33854910133951,-1.56050861525176,
8.55006272177992));
#49451=CARTESIAN_POINT('Ctrl Pts',(-1.39110142157108,-1.51386129057278,
8.54624241091833));
#49452=CARTESIAN_POINT('Ctrl Pts',(-1.44120640785681,-1.46455510393172,
8.54242210005673));
#49453=CARTESIAN_POINT('Ctrl Pts',(-1.49122604728079,-1.41533290350854,
8.53860829656232));
#49454=CARTESIAN_POINT('Ctrl Pts',(-1.53880627704515,-1.36346118031355,
8.5347944930679));
#49455=CARTESIAN_POINT('Ctrl Pts',(-1.58365108837674,-1.30921609858081,
8.53098068957349));
#49456=CARTESIAN_POINT('Ctrl Pts',(-1.62845321325744,-1.25502265113862,
8.52717051632593));
#49457=CARTESIAN_POINT('Ctrl Pts',(-1.67052476385377,-1.19846070522761,
8.52336034307837));
#49458=CARTESIAN_POINT('Ctrl Pts',(-1.70960699564656,-1.13984274482769,
8.51955016983081));
#49459=CARTESIAN_POINT('Ctrl Pts',(-1.74866589227533,-1.08125978395718,
8.51574227155614));
#49460=CARTESIAN_POINT('Ctrl Pts',(-1.78473873300152,-1.02062365730354,
8.51193437328147));
#49461=CARTESIAN_POINT('Ctrl Pts',(-1.81760863708442,-0.958277832831442,
8.5081264750068));
#49462=CARTESIAN_POINT('Ctrl Pts',(-1.85047057485056,-0.895947118430393,
8.50431949961052));
#49463=CARTESIAN_POINT('Ctrl Pts',(-1.88013088470096,-0.831907970450107,
8.50051252421422));
#49464=CARTESIAN_POINT('Ctrl Pts',(-1.90641836529415,-0.766528915938064,
8.49670554881793));
#49465=CARTESIAN_POINT('Ctrl Pts',(-1.93272464880456,-0.701103097075756,
8.49289585036711));
#49466=CARTESIAN_POINT('Ctrl Pts',(-1.95565309513118,-0.634335920452832,
8.48908615191628));
#49467=CARTESIAN_POINT('Ctrl Pts',(-1.97508093173989,-0.566615280042358,
8.48527645346546));
#49468=CARTESIAN_POINT('Ctrl Pts',(-1.99451568455286,-0.498870531451931,
8.48146539878269));
#49469=CARTESIAN_POINT('Ctrl Pts',(-2.01044723129373,-0.430172129688349,
8.47765434409992));
#49470=CARTESIAN_POINT('Ctrl Pts',(-2.02280361780844,-0.360919778179445,
8.47384328941715));
#49471=CARTESIAN_POINT('Ctrl Pts',(-2.0351795119928,-0.291558094383596,
8.47002621802426));
#49472=CARTESIAN_POINT('Ctrl Pts',(-2.04396891161403,-0.221641210370022,
8.46620914663137));
#49473=CARTESIAN_POINT('Ctrl Pts',(-2.04915169493153,-0.151574713126082,
8.46239207523848));
#49474=CARTESIAN_POINT('Ctrl Pts',(-2.05291610382554,-0.100683342748401,
8.45961962332987));
#49475=CARTESIAN_POINT('Ctrl Pts',(-2.05477892290776,-0.0497131519036452,
8.45684717142126));
#49476=CARTESIAN_POINT('Ctrl Pts',(-2.05474966036672,0.00118140715607104,
8.45407471951265));
#49477=CARTESIAN_POINT('Origin',(0.,0.,18.5459252805377));
#49478=CARTESIAN_POINT('',(1.25005255340789,1.62658210076147,9.60609423337355));
#49479=CARTESIAN_POINT('',(1.25206542099588,1.62921138715834,9.54788499192677));
#49480=CARTESIAN_POINT('',(1.25206542099588,1.62921138715835,18.5459252805377));
#49481=CARTESIAN_POINT('',(-2.0547494382537,-0.00151937358419461,9.09592528053767));
#49482=CARTESIAN_POINT('Ctrl Pts',(1.25206542099588,1.62921138715834,9.54788499192677));
#49483=CARTESIAN_POINT('Ctrl Pts',(1.30837948877059,1.58593345678534,9.54402021208199));
#49484=CARTESIAN_POINT('Ctrl Pts',(1.36254035296318,1.53966063449194,9.54015543223721));
#49485=CARTESIAN_POINT('Ctrl Pts',(1.41421380051509,1.49063640400088,9.53629065239243));
#49486=CARTESIAN_POINT('Ctrl Pts',(1.4658192534186,1.44167668217865,9.53243095802886));
#49487=CARTESIAN_POINT('Ctrl Pts',(1.51494344120504,1.38997307654059,9.5285712636653));
#49488=CARTESIAN_POINT('Ctrl Pts',(1.56128488797241,1.33580951527116,9.52471156930173));
#49489=CARTESIAN_POINT('Ctrl Pts',(1.60759282263362,1.28168512271877,9.52085466610021));
#49490=CARTESIAN_POINT('Ctrl Pts',(1.65112169351406,1.22510467151956,9.51699776289868));
#49491=CARTESIAN_POINT('Ctrl Pts',(1.69160760247761,1.16638813511625,9.51314085969715));
#49492=CARTESIAN_POINT('Ctrl Pts',(1.73207777713509,1.10769441810808,9.50928545542938));
#49493=CARTESIAN_POINT('Ctrl Pts',(1.76950706155502,1.0468666631196,9.50543005116161));
#49494=CARTESIAN_POINT('Ctrl Pts',(1.80367357484215,0.984255656786465,9.50157464689384));
#49495=CARTESIAN_POINT('Ctrl Pts',(1.83783823880112,0.921648039394291,9.49771945130723));
#49496=CARTESIAN_POINT('Ctrl Pts',(1.86874025100017,0.857257789492544,9.49386425572062));
#49497=CARTESIAN_POINT('Ctrl Pts',(1.8962034405214,0.791460722117526,9.49000906013401));
#49498=CARTESIAN_POINT('Ctrl Pts',(1.92369373512672,0.725598715634017,9.48615005962152));
#49499=CARTESIAN_POINT('Ctrl Pts',(1.94773824003505,0.658327567596629,9.48229105910902));
#49500=CARTESIAN_POINT('Ctrl Pts',(1.96820911877231,0.590042733436753,9.47843205859653));
#49501=CARTESIAN_POINT('Ctrl Pts',(1.98868987694765,0.521724944375491,9.4745711956942));
#49502=CARTESIAN_POINT('Ctrl Pts',(2.00559345799348,0.452392967291722,9.47071033279187));
#49503=CARTESIAN_POINT('Ctrl Pts',(2.01884279277754,0.382454364009832,9.46684946988954));
#49504=CARTESIAN_POINT('Ctrl Pts',(2.03211648364741,0.312387193471582,9.46298150961141));
#49505=CARTESIAN_POINT('Ctrl Pts',(2.0417224414168,0.241711651288871,9.45911354933328));
#49506=CARTESIAN_POINT('Ctrl Pts',(2.04763537173146,0.170841876992033,9.45524558905514));
#49507=CARTESIAN_POINT('Ctrl Pts',(2.05279162390166,0.109041313130481,9.45187261194954));
#49508=CARTESIAN_POINT('Ctrl Pts',(2.05514038457062,0.0470933095698247,
9.44849963484393));
#49509=CARTESIAN_POINT('Ctrl Pts',(2.05469720726044,-0.0147291878983883,
9.44512665773833));
#49510=CARTESIAN_POINT('Ctrl Pts',(2.05418884634507,-0.0856446898450993,
9.44125757489156));
#49511=CARTESIAN_POINT('Ctrl Pts',(2.05000382978784,-0.156672739017571,
9.43738849204479));
#49512=CARTESIAN_POINT('Ctrl Pts',(2.042127920654,-0.227400787565428,9.43351940919801));
#49513=CARTESIAN_POINT('Ctrl Pts',(2.03426374623198,-0.29802345484829,9.42965609109173));
#49514=CARTESIAN_POINT('Ctrl Pts',(2.02271964840836,-0.368346529895437,
9.42579277298544));
#49515=CARTESIAN_POINT('Ctrl Pts',(2.00753339905201,-0.437958005053798,
9.42192945487916));
#49516=CARTESIAN_POINT('Ctrl Pts',(1.99236496316031,-0.507487825978572,
9.41807066844352));
#49517=CARTESIAN_POINT('Ctrl Pts',(1.97356296489507,-0.576307232707317,
9.41421188200788));
#49518=CARTESIAN_POINT('Ctrl Pts',(1.9512166949604,-0.644011623969472,9.41035309557225));
#49519=CARTESIAN_POINT('Ctrl Pts',(1.92888450153722,-0.711673366429671,
9.40649673988912));
#49520=CARTESIAN_POINT('Ctrl Pts',(1.90301261784714,-0.778221026714865,
9.40264038420599));
#49521=CARTESIAN_POINT('Ctrl Pts',(1.87374053468269,-0.843263879925522,
9.39878402852285));
#49522=CARTESIAN_POINT('Ctrl Pts',(1.84447709878471,-0.908287518826033,
9.3949288120458));
#49523=CARTESIAN_POINT('Ctrl Pts',(1.81181565678583,-0.971806790429911,
9.39107359556876));
#49524=CARTESIAN_POINT('Ctrl Pts',(1.77594366512749,-1.03345133450662,9.38721837909171));
#49525=CARTESIAN_POINT('Ctrl Pts',(1.74007027098157,-1.09509828870065,9.38336301188723));
#49526=CARTESIAN_POINT('Ctrl Pts',(1.70098632419905,-1.15486995108761,9.37950764468274));
#49527=CARTESIAN_POINT('Ctrl Pts',(1.65892415623246,-1.21242245375464,9.37565227747826));
#49528=CARTESIAN_POINT('Ctrl Pts',(1.61681796064581,-1.27003519819815,9.37179287475562));
#49529=CARTESIAN_POINT('Ctrl Pts',(1.57172760810276,-1.3254237529768,9.36793347203299));
#49530=CARTESIAN_POINT('Ctrl Pts',(1.52392698066661,-1.37827577795459,9.36407406931035));
#49531=CARTESIAN_POINT('Ctrl Pts',(1.47609928813973,-1.43115772816408,9.36021248136357));
#49532=CARTESIAN_POINT('Ctrl Pts',(1.42555861018493,-1.48149994654887,9.3563508934168));
#49533=CARTESIAN_POINT('Ctrl Pts',(1.37261515912689,-1.52902752997945,9.35248930547002));
#49534=CARTESIAN_POINT('Ctrl Pts',(1.31957908160349,-1.57663826462085,9.34862096153672));
#49535=CARTESIAN_POINT('Ctrl Pts',(1.26413221611949,-1.62142422745431,9.34475261760341));
#49536=CARTESIAN_POINT('Ctrl Pts',(1.2066166827877,-1.66315174993697,9.34088427367011));
#49537=CARTESIAN_POINT('Ctrl Pts',(1.172465614227,-1.68792835198902,9.33858736236233));
#49538=CARTESIAN_POINT('Ctrl Pts',(1.13758575582091,-1.71162749254131,9.33629045105455));
#49539=CARTESIAN_POINT('Ctrl Pts',(1.10205285120755,-1.73420791015533,9.33399353974677));
#49540=CARTESIAN_POINT('Ctrl Pts',(1.04219866733299,-1.77224399199384,9.33012445689933));
#49541=CARTESIAN_POINT('Ctrl Pts',(0.98025578314655,-1.80725223721137,9.3262553740519));
#49542=CARTESIAN_POINT('Ctrl Pts',(0.916563071910391,-1.83899692705295,
9.32238629120446));
#49543=CARTESIAN_POINT('Ctrl Pts',(0.852965259637481,-1.87069431888984,
9.3185229730975));
#49544=CARTESIAN_POINT('Ctrl Pts',(0.787623226678478,-1.89913759241964,
9.31465965499054));
#49545=CARTESIAN_POINT('Ctrl Pts',(0.720903601009475,-1.924135016196,9.31079633688358));
#49546=CARTESIAN_POINT('Ctrl Pts',(0.65426223743565,-1.94910311800391,9.30693755044728));
#49547=CARTESIAN_POINT('Ctrl Pts',(0.586246943603025,-1.97063322919154,
9.30307876401097));
#49548=CARTESIAN_POINT('Ctrl Pts',(0.517246067943104,-1.9885809180663,9.29921997757466));
#49549=CARTESIAN_POINT('Ctrl Pts',(0.448288657775253,-2.0065173012131,9.29536362189086));
#49550=CARTESIAN_POINT('Ctrl Pts',(0.378347366553541,-2.02087561723382,
9.29150726620705));
#49551=CARTESIAN_POINT('Ctrl Pts',(0.307826112251187,-2.03156113546118,
9.28765091052325));
#49552=CARTESIAN_POINT('Ctrl Pts',(0.237325690633525,-2.04224349707946,
9.28379569404553));
#49553=CARTESIAN_POINT('Ctrl Pts',(0.166246126105861,-2.04925514215687,
9.27994047756781));
#49554=CARTESIAN_POINT('Ctrl Pts',(0.095000243233387,-2.05255268295009,
9.27608526109009));
#49555=CARTESIAN_POINT('Ctrl Pts',(0.0237515748600807,-2.05585035266728,
9.27222989388494));
#49556=CARTESIAN_POINT('Ctrl Pts',(-0.0476629394025676,-2.05543360954481,
9.2683745266798));
#49557=CARTESIAN_POINT('Ctrl Pts',(-0.118828392738864,-2.05131113573224,
9.26451915947465));
#49558=CARTESIAN_POINT('Ctrl Pts',(-0.190068336898829,-2.04718434681374,
9.26065975675135));
#49559=CARTESIAN_POINT('Ctrl Pts',(-0.261058213755417,-2.03934411222334,
9.25680035402806));
#49560=CARTESIAN_POINT('Ctrl Pts',(-0.331387067787583,-2.02785112219885,
9.25294095130476));
#49561=CARTESIAN_POINT('Ctrl Pts',(-0.401755742569288,-2.01635162475314,
9.24907936335732));
#49562=CARTESIAN_POINT('Ctrl Pts',(-0.47146217454117,-2.00119535794867,
9.24521777540989));
#49563=CARTESIAN_POINT('Ctrl Pts',(-0.54010715543086,-1.98249383937312,
9.24135618746246));
#49564=CARTESIAN_POINT('Ctrl Pts',(-0.60887223317487,-1.96375960182056,
9.23748784352851));
#49565=CARTESIAN_POINT('Ctrl Pts',(-0.676571690631472,-1.9414678809202,
9.23361949959456));
#49566=CARTESIAN_POINT('Ctrl Pts',(-0.742823655912128,-1.91577936587628,
9.22975115566061));
#49567=CARTESIAN_POINT('Ctrl Pts',(-0.78216216624574,-1.90052626492706,
9.22745424435881));
#49568=CARTESIAN_POINT('Ctrl Pts',(-0.820990746805723,-1.88407648961503,
9.22515733305701));
#49569=CARTESIAN_POINT('Ctrl Pts',(-0.859233650634652,-1.86647129528344,
9.22286042175521));
#49570=CARTESIAN_POINT('Ctrl Pts',(-0.923652752532163,-1.83681583782536,
9.21899133890884));
#49571=CARTESIAN_POINT('Ctrl Pts',(-0.986660938675525,-1.80376335515144,
9.21512225606246));
#49572=CARTESIAN_POINT('Ctrl Pts',(-1.04787637575334,-1.7674706966844,9.21125317321608));
#49573=CARTESIAN_POINT('Ctrl Pts',(-1.10900060488281,-1.73123211246852,
9.20738985511019));
#49574=CARTESIAN_POINT('Ctrl Pts',(-1.16833697255914,-1.69176318103148,
9.20352653700429));
#49575=CARTESIAN_POINT('Ctrl Pts',(-1.22552554705327,-1.6492679272998,9.1996632188984));
#49576=CARTESIAN_POINT('Ctrl Pts',(-1.28264703937168,-1.60682252048429,
9.19580443246315));
#49577=CARTESIAN_POINT('Ctrl Pts',(-1.33762535478415,-1.56135813095968,
9.19194564602789));
#49578=CARTESIAN_POINT('Ctrl Pts',(-1.39012851890175,-1.51312268618114,
9.18808685959264));
#49579=CARTESIAN_POINT('Ctrl Pts',(-1.44259860987588,-1.46491762619582,
9.18423050390989));
#49580=CARTESIAN_POINT('Ctrl Pts',(-1.49259628602557,-1.41394530200018,
9.18037414822714));
#49581=CARTESIAN_POINT('Ctrl Pts',(-1.53982288382424,-1.36049367839443,
9.17651779254438));
#49582=CARTESIAN_POINT('Ctrl Pts',(-1.58703553041312,-1.3070578449334,9.17266257606771));
#49583=CARTESIAN_POINT('Ctrl Pts',(-1.63147840233561,-1.25114452994511,
9.16880735959103));
#49584=CARTESIAN_POINT('Ctrl Pts',(-1.67289114019362,-1.19307702834381,
9.16495214311435));
#49585=CARTESIAN_POINT('Ctrl Pts',(-1.71430549716584,-1.13500725647684,
9.16109677591023));
#49586=CARTESIAN_POINT('Ctrl Pts',(-1.75268920459536,-1.07478352756789,
9.15724140870612));
#49587=CARTESIAN_POINT('Ctrl Pts',(-1.78782451935178,-1.01275912758393,
9.15338604150201));
#49588=CARTESIAN_POINT('Ctrl Pts',(-1.82299661120194,-0.950669804966202,
9.14952663877972));
#49589=CARTESIAN_POINT('Ctrl Pts',(-1.85491328292847,-0.886776472309764,
9.14566723605744));
#49590=CARTESIAN_POINT('Ctrl Pts',(-1.88340262822067,-0.821457304131785,
9.14180783333516));
#49591=CARTESIAN_POINT('Ctrl Pts',(-1.91190810440402,-0.756101151727558,
9.13794624538873));
#49592=CARTESIAN_POINT('Ctrl Pts',(-1.93698222022606,-0.689318011678123,
9.1340846574423));
#49593=CARTESIAN_POINT('Ctrl Pts',(-1.95850214259047,-0.621503757002758,
9.13022306949587));
#49594=CARTESIAN_POINT('Ctrl Pts',(-1.9800597148305,-0.553570858857855,
9.1263547255629));
#49595=CARTESIAN_POINT('Ctrl Pts',(-1.99805055616579,-0.484603714607712,
9.12248638162993));
#49596=CARTESIAN_POINT('Ctrl Pts',(-2.01240254711499,-0.415010302119222,
9.11861803769696));
#49597=CARTESIAN_POINT('Ctrl Pts',(-2.02092434634467,-0.373687736418489,
9.11632112638586));
#49598=CARTESIAN_POINT('Ctrl Pts',(-2.02816420397466,-0.332144526961971,
9.11402421507476));
#49599=CARTESIAN_POINT('Ctrl Pts',(-2.03411569632439,-0.290466687361487,
9.11172730376365));
#49600=CARTESIAN_POINT('Ctrl Pts',(-2.04776382455714,-0.194889903270089,
9.10645996268833));
#49601=CARTESIAN_POINT('Ctrl Pts',(-2.05467785275471,-0.0983291808467869,
9.101192621613));
#49602=CARTESIAN_POINT('Ctrl Pts',(-2.0547494382537,-0.00151937358419461,
9.09592528053767));
#49603=CARTESIAN_POINT('Ctrl Pts',(-2.05657619914637,-0.00150476774419542,
9.09592441312253));
#49604=CARTESIAN_POINT('Ctrl Pts',(-2.05172851349779,0.583051337434284,
9.06414767067239));
#49605=CARTESIAN_POINT('Ctrl Pts',(-1.48485246887974,1.85727103545833,8.99532655555841));
#49606=CARTESIAN_POINT('Ctrl Pts',(0.203568424281083,2.2283551924176,8.91263733706201));
#49607=CARTESIAN_POINT('Ctrl Pts',(1.0481375467077,1.78481282053903,8.86172486101579));
#49608=CARTESIAN_POINT('Ctrl Pts',(1.25051812704735,1.62722676461089,8.84785675763342));
#49609=CARTESIAN_POINT('',(-2.05468488894014,0.00105741319522436,9.15407467172219));
#49610=CARTESIAN_POINT('Ctrl Pts',(-2.05474972788973,0.00105746728722069,
9.15407467060216));
#49611=CARTESIAN_POINT('Ctrl Pts',(-2.05470909252753,0.0800154647999912,
9.14981306013524));
#49612=CARTESIAN_POINT('Ctrl Pts',(-2.05011312005515,0.158816114439893,
9.14555144966831));
#49613=CARTESIAN_POINT('Ctrl Pts',(-2.04104077392044,0.236960169003702,
9.14128983920139));
#49614=CARTESIAN_POINT('Ctrl Pts',(-2.03193556684571,0.315387269105138,
9.13701279275751));
#49615=CARTESIAN_POINT('Ctrl Pts',(-2.0183216354985,0.393152725894291,9.13273574631362));
#49616=CARTESIAN_POINT('Ctrl Pts',(-2.00032874250127,0.46976854345868,9.12845869986974));
#49617=CARTESIAN_POINT('Ctrl Pts',(-1.98224879419337,0.546755052595601,
9.12416095972158));
#49618=CARTESIAN_POINT('Ctrl Pts',(-1.95974754943351,0.622580496287309,
9.11986321957341));
#49619=CARTESIAN_POINT('Ctrl Pts',(-1.93300491868768,0.696770799351727,
9.11556547942525));
#49620=CARTESIAN_POINT('Ctrl Pts',(-1.92052498157348,0.731393059425061,
9.11355986048327));
#49621=CARTESIAN_POINT('Ctrl Pts',(-1.9071220283947,0.765659543230826,9.11155424154129));
#49622=CARTESIAN_POINT('Ctrl Pts',(-1.89281777540094,0.799523878083839,
9.10954862259931));
#49623=CARTESIAN_POINT('Ctrl Pts',(-1.86522313179983,0.864852298342182,
9.10567953975186));
#49624=CARTESIAN_POINT('Ctrl Pts',(-1.83418836795403,0.928878399016742,
9.10181045690442));
#49625=CARTESIAN_POINT('Ctrl Pts',(-1.7998581277094,0.991215558099463,9.09794137405698));
#49626=CARTESIAN_POINT('Ctrl Pts',(-1.76557903781057,1.0534598379241,9.09407805595001));
#49627=CARTESIAN_POINT('Ctrl Pts',(-1.72801445035035,1.11401974916303,9.09021473784305));
#49628=CARTESIAN_POINT('Ctrl Pts',(-1.68735685644335,1.17252906211898,9.08635141973609));
#49629=CARTESIAN_POINT('Ctrl Pts',(-1.64674695387837,1.23096974367333,9.08249263329978));
#49630=CARTESIAN_POINT('Ctrl Pts',(-1.60305152735594,1.28736420779808,9.07863384686347));
#49631=CARTESIAN_POINT('Ctrl Pts',(-1.55650783625712,1.34137277375463,9.07477506042716));
#49632=CARTESIAN_POINT('Ctrl Pts',(-1.50999346427081,1.39534731827487,9.07091870474335));
#49633=CARTESIAN_POINT('Ctrl Pts',(-1.46063470374567,1.4469385793191,9.06706234905955));
#49634=CARTESIAN_POINT('Ctrl Pts',(-1.40870988911519,1.49583889868163,9.06320599337574));
#49635=CARTESIAN_POINT('Ctrl Pts',(-1.35680041359492,1.54472477240014,9.05935077689802));
#49636=CARTESIAN_POINT('Ctrl Pts',(-1.3023267423383,1.59092094973071,9.0554955604203));
#49637=CARTESIAN_POINT('Ctrl Pts',(-1.24560373855348,1.63415693524264,9.05164034394258));
#49638=CARTESIAN_POINT('Ctrl Pts',(-1.18887851706889,1.67739461115225,9.04778497673743));
#49639=CARTESIAN_POINT('Ctrl Pts',(-1.12990417614052,1.71767157273418,9.04392960953228));
#49640=CARTESIAN_POINT('Ctrl Pts',(-1.06902690833012,1.75475896685731,9.04007424232713));
#49641=CARTESIAN_POINT('Ctrl Pts',(-1.00808591862087,1.79188518136878,9.03621483960383));
#49642=CARTESIAN_POINT('Ctrl Pts',(-0.945238441568808,1.82581491055631,
9.03235543688053));
#49643=CARTESIAN_POINT('Ctrl Pts',(-0.880857001440585,1.85636432456377,
9.02849603415723));
#49644=CARTESIAN_POINT('Ctrl Pts',(-0.816439108035306,1.88693103588938,
9.0246344462098));
#49645=CARTESIAN_POINT('Ctrl Pts',(-0.750485971899848,1.9141134367325,9.02077285826237));
#49646=CARTESIAN_POINT('Ctrl Pts',(-0.68338936536759,1.93777618361938,9.01691127031493));
#49647=CARTESIAN_POINT('Ctrl Pts',(-0.616175370917405,1.96148032933002,
9.01304292638098));
#49648=CARTESIAN_POINT('Ctrl Pts',(-0.54781437800007,1.98165238941271,9.00917458244703));
#49649=CARTESIAN_POINT('Ctrl Pts',(-0.478711868279485,1.99820732399528,
9.00530623851308));
#49650=CARTESIAN_POINT('Ctrl Pts',(-0.437680786692985,2.00803716771966,
9.0030093272113));
#49651=CARTESIAN_POINT('Ctrl Pts',(-0.3963884600947,2.01659272382017,9.00071241590952));
#49652=CARTESIAN_POINT('Ctrl Pts',(-0.3549206547011,2.02386484019229,8.99841550460774));
#49653=CARTESIAN_POINT('Ctrl Pts',(-0.285091861551083,2.03611055961465,
8.99454767165508));
#49654=CARTESIAN_POINT('Ctrl Pts',(-0.214491835897539,2.04476209373249,
8.99067983870242));
#49655=CARTESIAN_POINT('Ctrl Pts',(-0.143523450780166,2.04973134375609,
8.98681200574976));
#49656=CARTESIAN_POINT('Ctrl Pts',(-0.0726506121767563,2.05469390355396,
8.98294938015746));
#49657=CARTESIAN_POINT('Ctrl Pts',(-0.00141087773771996,2.05598397860889,
8.97908675456515));
#49658=CARTESIAN_POINT('Ctrl Pts',(0.0697838918775918,2.05356464980638,
8.97522412897285));
#49659=CARTESIAN_POINT('Ctrl Pts',(0.1409066324066,2.05114776868429,8.97136541127144));
#49660=CARTESIAN_POINT('Ctrl Pts',(0.21198401549772,2.04502894632438,8.96750669357003));
#49661=CARTESIAN_POINT('Ctrl Pts',(0.282602001321962,2.03522324852799,8.96364797586862));
#49662=CARTESIAN_POINT('Ctrl Pts',(0.353172167215793,2.02542419079334,8.95979187115044));
#49663=CARTESIAN_POINT('Ctrl Pts',(0.423283073477898,2.01194328047611,8.95593576643225));
#49664=CARTESIAN_POINT('Ctrl Pts',(0.49252535892379,1.99484744612639,8.95207966171406));
#49665=CARTESIAN_POINT('Ctrl Pts',(0.5617703014393,1.97775095574948,8.9482234090236));
#49666=CARTESIAN_POINT('Ctrl Pts',(0.630146080390361,1.95703936211572,8.94436715633313));
#49667=CARTESIAN_POINT('Ctrl Pts',(0.697254340464982,1.93283055315326,8.94051090364267));
#49668=CARTESIAN_POINT('Ctrl Pts',(0.76435907002111,1.90862301779927,8.93665485382695));
#49669=CARTESIAN_POINT('Ctrl Pts',(0.830195958385753,1.8809188049123,8.93279880401124));
#49670=CARTESIAN_POINT('Ctrl Pts',(0.894384763685532,1.84988471451255,8.92894275419552));
#49671=CARTESIAN_POINT('Ctrl Pts',(0.958639725066976,1.81881863888096,8.9250827301487));
#49672=CARTESIAN_POINT('Ctrl Pts',(1.0212427742253,1.78441604733185,8.92122270610188));
#49673=CARTESIAN_POINT('Ctrl Pts',(1.08183724595149,1.74689030444734,8.91736268205507));
#49674=CARTESIAN_POINT('Ctrl Pts',(1.14056599836375,1.71051998880353,8.91362150913791));
#49675=CARTESIAN_POINT('Ctrl Pts',(1.19740775918225,1.67121635280537,8.90988033622077));
#49676=CARTESIAN_POINT('Ctrl Pts',(1.25206542099588,1.62921138715834,8.90613916330362));
#49677=CARTESIAN_POINT('Ctrl Pts',(1.25005255340789,1.62658210076147,9.60609423337355));
#49678=CARTESIAN_POINT('Ctrl Pts',(1.50489202993141,1.43143452431908,9.58875652043754));
#49679=CARTESIAN_POINT('Ctrl Pts',(2.16745735673946,0.642365888481017,9.53437443483768));
#49680=CARTESIAN_POINT('Ctrl Pts',(2.07210355506776,-1.2666354657809,9.44294797657398));
#49681=CARTESIAN_POINT('Ctrl Pts',(0.0597258374687065,-2.4278408865574,
9.33181485858242));
#49682=CARTESIAN_POINT('Ctrl Pts',(-1.7312581697553,-1.50866925322773,9.23552377287854));
#49683=CARTESIAN_POINT('Ctrl Pts',(-2.05000971940957,-0.409738837837595,
9.1762770598385));
#49684=CARTESIAN_POINT('Ctrl Pts',(-2.0519211775981,0.00105510756466237,
9.15407471946233));
#49685=CARTESIAN_POINT('Origin',(0.,0.,18.5459252805377));
#49686=CARTESIAN_POINT('',(1.25206542099588,1.62921138715834,10.3060095422728));
#49687=CARTESIAN_POINT('',(1.25206542099587,1.62921138715835,10.2479916911084));
#49688=CARTESIAN_POINT('',(1.25206542099588,1.62921138715835,18.5459252805377));
#49689=CARTESIAN_POINT('',(-2.0547493654031,0.0016148918149348,9.79592528057681));
#49690=CARTESIAN_POINT('Ctrl Pts',(1.25206542099587,1.62921138715835,10.2479916911084));
#49691=CARTESIAN_POINT('Ctrl Pts',(1.30857145584848,1.58578592814536,10.2441287597561));
#49692=CARTESIAN_POINT('Ctrl Pts',(1.36275485896034,1.53946409868074,10.2402658284038));
#49693=CARTESIAN_POINT('Ctrl Pts',(1.41431998267322,1.49053565845008,10.2364028970515));
#49694=CARTESIAN_POINT('Ctrl Pts',(1.4659685929782,1.44152800055373,10.2325337114143));
#49695=CARTESIAN_POINT('Ctrl Pts',(1.51499013745528,1.38990566754411,10.2286645257772));
#49696=CARTESIAN_POINT('Ctrl Pts',(1.56112811870158,1.33599272434368,10.22479534014));
#49697=CARTESIAN_POINT('Ctrl Pts',(1.5680318152698,1.327925648349,10.2242163879864));
#49698=CARTESIAN_POINT('Ctrl Pts',(1.5748710286009,1.31980734010624,10.2236374358328));
#49699=CARTESIAN_POINT('Ctrl Pts',(1.58164498343667,1.31163893997915,10.2230584836792));
#49700=CARTESIAN_POINT('Ctrl Pts',(1.62691468715583,1.25705028939348,10.2191894008323));
#49701=CARTESIAN_POINT('Ctrl Pts',(1.66944364287453,1.2000083218721,10.2153203179854));
#49702=CARTESIAN_POINT('Ctrl Pts',(1.70895533975419,1.14081953403053,10.2114512351385));
#49703=CARTESIAN_POINT('Ctrl Pts',(1.74840816617605,1.08171893453096,10.207587917032));
#49704=CARTESIAN_POINT('Ctrl Pts',(1.78485238981659,1.0204782646924,10.2037245989256));
#49705=CARTESIAN_POINT('Ctrl Pts',(1.81805164243257,0.957437093467896,10.1998612808192));
#49706=CARTESIAN_POINT('Ctrl Pts',(1.851211952338,0.894469869512967,10.1960024943834));
#49707=CARTESIAN_POINT('Ctrl Pts',(1.88113462665997,0.829706767031211,10.1921437079476));
#49708=CARTESIAN_POINT('Ctrl Pts',(1.90762748561629,0.763514858153578,10.1882849215118));
#49709=CARTESIAN_POINT('Ctrl Pts',(1.9341036560141,0.697364645324893,10.1844285658285));
#49710=CARTESIAN_POINT('Ctrl Pts',(1.95715411742514,0.629787861706434,10.1805722101452));
#49711=CARTESIAN_POINT('Ctrl Pts',(1.97663403516038,0.561173282993416,10.176715854462));
#49712=CARTESIAN_POINT('Ctrl Pts',(1.99610819833286,0.492578973714011,10.1728606379848));
#49713=CARTESIAN_POINT('Ctrl Pts',(2.01201377924935,0.422947945037063,10.1690054215076));
#49714=CARTESIAN_POINT('Ctrl Pts',(2.02425575608784,0.352684273033582,10.1651502050304));
#49715=CARTESIAN_POINT('Ctrl Pts',(2.03649821155102,0.282417853930677,10.1612948378257));
#49716=CARTESIAN_POINT('Ctrl Pts',(2.04507669734875,0.211519221345956,10.1574394706211));
#49717=CARTESIAN_POINT('Ctrl Pts',(2.04994758497279,0.140401073230255,10.1535841034165));
#49718=CARTESIAN_POINT('Ctrl Pts',(2.05482357108796,0.0692084838064535,
10.1497247006937));
#49719=CARTESIAN_POINT('Ctrl Pts',(2.05598417873304,-0.00220359418590887,
10.1458652979709));
#49720=CARTESIAN_POINT('Ctrl Pts',(2.05343787109383,-0.073419834225099,
10.1420058952481));
#49721=CARTESIAN_POINT('Ctrl Pts',(2.05089012171523,-0.144676397458819,
10.1381443073012));
#49722=CARTESIAN_POINT('Ctrl Pts',(2.04463132146234,-0.215736417862735,
10.1342827193543));
#49723=CARTESIAN_POINT('Ctrl Pts',(2.03472183547422,-0.286189822922526,
10.1304211314073));
#49724=CARTESIAN_POINT('Ctrl Pts',(2.02479501248517,-0.356766488739775,
10.1265527874739));
#49725=CARTESIAN_POINT('Ctrl Pts',(2.0112048445784,-0.426733943285215,10.1226844435404));
#49726=CARTESIAN_POINT('Ctrl Pts',(1.99406266002678,-0.49569312118175,10.118816099607));
#49727=CARTESIAN_POINT('Ctrl Pts',(1.98388412414919,-0.536639096544201,
10.1165191883005));
#49728=CARTESIAN_POINT('Ctrl Pts',(1.97245423162198,-0.57722987554729,10.1142222769941));
#49729=CARTESIAN_POINT('Ctrl Pts',(1.95980437203989,-0.617385119543161,
10.1119253656877));
#49730=CARTESIAN_POINT('Ctrl Pts',(1.93849603741333,-0.685025504839332,
10.1080562828408));
#49731=CARTESIAN_POINT('Ctrl Pts',(1.91364006230091,-0.751693927907768,
10.1041871999939));
#49732=CARTESIAN_POINT('Ctrl Pts',(1.88534397061039,-0.816991845114166,
10.1003181171469));
#49733=CARTESIAN_POINT('Ctrl Pts',(1.85709003868528,-0.882192471680514,
10.0964547990405));
#49734=CARTESIAN_POINT('Ctrl Pts',(1.8254063559399,-0.946026203568283,10.0925914809341));
#49735=CARTESIAN_POINT('Ctrl Pts',(1.7904500040004,-1.00811028448031,10.0887281628276));
#49736=CARTESIAN_POINT('Ctrl Pts',(1.75553465584828,-1.0701215407893,10.0848693763919));
#49737=CARTESIAN_POINT('Ctrl Pts',(1.7173545009178,-1.13038680152145,10.0810105899561));
#49738=CARTESIAN_POINT('Ctrl Pts',(1.67611369411628,-1.18854551738496,10.0771518035203));
#49739=CARTESIAN_POINT('Ctrl Pts',(1.63489886599898,-1.24666759752208,10.073295447837));
#49740=CARTESIAN_POINT('Ctrl Pts',(1.59062749143636,-1.30268537014652,10.0694390921537));
#49741=CARTESIAN_POINT('Ctrl Pts',(1.54354763826478,-1.3562662905592,10.0655827364705));
#49742=CARTESIAN_POINT('Ctrl Pts',(1.49648169295327,-1.40983138263144,10.0617275199933));
#49743=CARTESIAN_POINT('Ctrl Pts',(1.44660923659695,-1.46096068690869,10.0578723035161));
#49744=CARTESIAN_POINT('Ctrl Pts',(1.39421820890273,-1.50935520950638,10.0540170870389));
#49745=CARTESIAN_POINT('Ctrl Pts',(1.34182513287606,-1.55775162418514,10.0501617198343));
#49746=CARTESIAN_POINT('Ctrl Pts',(1.28691364835081,-1.60341271690293,10.0463063526296));
#49747=CARTESIAN_POINT('Ctrl Pts',(1.22980681328235,-1.64607799466013,10.042450985425));
#49748=CARTESIAN_POINT('Ctrl Pts',(1.17264020292981,-1.68878793132891,10.0385915827022));
#49749=CARTESIAN_POINT('Ctrl Pts',(1.11327404480641,-1.72849550192885,10.0347321799794));
#49750=CARTESIAN_POINT('Ctrl Pts',(1.05206185872653,-1.76498255173044,10.0308727772566));
#49751=CARTESIAN_POINT('Ctrl Pts',(0.990815013826058,-1.80149026078623,
10.0270111893097));
#49752=CARTESIAN_POINT('Ctrl Pts',(0.927720490096649,-1.83477359228649,
10.0231496013628));
#49753=CARTESIAN_POINT('Ctrl Pts',(0.863155543885299,-1.86466084571969,
10.0192880134159));
#49754=CARTESIAN_POINT('Ctrl Pts',(0.798477638986301,-1.89460038797404,
10.0154196694824));
#49755=CARTESIAN_POINT('Ctrl Pts',(0.732324626438617,-1.92113180878327,
10.011551325549));
#49756=CARTESIAN_POINT('Ctrl Pts',(0.665092156530011,-1.94413219350492,
10.0076829816155));
#49757=CARTESIAN_POINT('Ctrl Pts',(0.625171450679649,-1.95778916005942,
10.0053860703091));
#49758=CARTESIAN_POINT('Ctrl Pts',(0.58487044581956,-1.97020216898538,10.0030891590026));
#49759=CARTESIAN_POINT('Ctrl Pts',(0.544273662203676,-1.9813540176181,10.0007922476961));
#49760=CARTESIAN_POINT('Ctrl Pts',(0.475889515769289,-2.00013899470224,
9.99692316484918));
#49761=CARTESIAN_POINT('Ctrl Pts',(0.406397776570062,-2.01541630848205,
9.99305408200225));
#49762=CARTESIAN_POINT('Ctrl Pts',(0.336191593147607,-2.02706013112509,
9.98918499915532));
#49763=CARTESIAN_POINT('Ctrl Pts',(0.266090013437113,-2.0386866050531,9.98532168104887));
#49764=CARTESIAN_POINT('Ctrl Pts',(0.195276577811771,-2.04669025509523,
9.98145836294242));
#49765=CARTESIAN_POINT('Ctrl Pts',(0.124158050480217,-2.05099545123848,
9.97759504483598));
#49766=CARTESIAN_POINT('Ctrl Pts',(0.0531229451538365,-2.05529559738832,
9.97373625840018));
#49767=CARTESIAN_POINT('Ctrl Pts',(-0.0182160584807071,-2.05590587773127,
9.96987747196439));
#49768=CARTESIAN_POINT('Ctrl Pts',(-0.0894453214332187,-2.05280225471761,
9.96601868552859));
#49769=CARTESIAN_POINT('Ctrl Pts',(-0.160629715173089,-2.04970058675887,
9.9621623298453));
#49770=CARTESIAN_POINT('Ctrl Pts',(-0.23170402120557,-2.04288967804532,
9.95830597416201));
#49771=CARTESIAN_POINT('Ctrl Pts',(-0.30225431061661,-2.03239757287143,
9.95444961847871));
#49772=CARTESIAN_POINT('Ctrl Pts',(-0.372783758765723,-2.02190856717046,
9.9505944020015));
#49773=CARTESIAN_POINT('Ctrl Pts',(-0.442789017377062,-2.00774059534358,
9.94673918552429));
#49774=CARTESIAN_POINT('Ctrl Pts',(-0.511862718967743,-1.98997339666412,
9.94288396904708));
#49775=CARTESIAN_POINT('Ctrl Pts',(-0.5809391211336,-1.97220550334033,9.93902860184243));
#49776=CARTESIAN_POINT('Ctrl Pts',(-0.649083424049654,-1.95083822693263,
9.93517323463779));
#49777=CARTESIAN_POINT('Ctrl Pts',(-0.715901558653159,-1.92600169283881,
9.93131786743315));
#49778=CARTESIAN_POINT('Ctrl Pts',(-0.78278963362311,-1.90113916166642,
9.92745846471035));
#49779=CARTESIAN_POINT('Ctrl Pts',(-0.848348312971446,-1.87280029338593,
9.92359906198755));
#49780=CARTESIAN_POINT('Ctrl Pts',(-0.912202575503724,-1.84116376885501,
9.91973965926475));
#49781=CARTESIAN_POINT('Ctrl Pts',(-0.976092992821027,-1.80950933147538,
9.91587807131782));
#49782=CARTESIAN_POINT('Ctrl Pts',(-1.03827664853373,-1.77455375906357,
9.91201648337088));
#49783=CARTESIAN_POINT('Ctrl Pts',(-1.09840467494435,-1.73652087017703,
9.90815489542395));
#49784=CARTESIAN_POINT('Ctrl Pts',(-1.15863789749239,-1.69842144138814,
9.90428655149049));
#49785=CARTESIAN_POINT('Ctrl Pts',(-1.21680791384032,-1.65723422786973,
9.90041820755702));
#49786=CARTESIAN_POINT('Ctrl Pts',(-1.27259686640149,-1.61322496203261,
9.89654986362356));
#49787=CARTESIAN_POINT('Ctrl Pts',(-1.30572274096442,-1.58709352645621,
9.89425295231723));
#49788=CARTESIAN_POINT('Ctrl Pts',(-1.33800979227511,-1.55996789096557,
9.8919560410109));
#49789=CARTESIAN_POINT('Ctrl Pts',(-1.36939772568353,-1.53190973343496,
9.88965912970457));
#49790=CARTESIAN_POINT('Ctrl Pts',(-1.42276852495404,-1.48420075323606,
9.88575355265758));
#49791=CARTESIAN_POINT('Ctrl Pts',(-1.47376547698587,-1.43358958402843,
9.88184797561058));
#49792=CARTESIAN_POINT('Ctrl Pts',(-1.52205085019631,-1.3803473374179,9.8779423985636));
#49793=CARTESIAN_POINT('Ctrl Pts',(-1.56909432278065,-1.32847448230223,
9.87413727302516));
#49794=CARTESIAN_POINT('Ctrl Pts',(-1.61356363799311,-1.27410464308286,
9.87033214748672));
#49795=CARTESIAN_POINT('Ctrl Pts',(-1.6551798379899,-1.2175291645015,9.86652702194828));
#49796=CARTESIAN_POINT('Ctrl Pts',(-1.69675650695488,-1.16100742670001,
9.86272551088062));
#49797=CARTESIAN_POINT('Ctrl Pts',(-1.73548513649758,-1.10228460370845,
9.85892399981296));
#49798=CARTESIAN_POINT('Ctrl Pts',(-1.77112604724776,-1.0416861750357,9.85512248874529));
#49799=CARTESIAN_POINT('Ctrl Pts',(-1.80674585565399,-0.981123625605609,
9.85132322848415));
#49800=CARTESIAN_POINT('Ctrl Pts',(-1.8392813171203,-0.918688104157346,
9.847523968223));
#49801=CARTESIAN_POINT('Ctrl Pts',(-1.86853633227469,-0.854733606142541,
9.84372470796185));
#49802=CARTESIAN_POINT('Ctrl Pts',(-1.89920837710276,-0.787681334259777,
9.83974142234643));
#49803=CARTESIAN_POINT('Ctrl Pts',(-1.92627380211056,-0.718959700575715,
9.83575813673102));
#49804=CARTESIAN_POINT('Ctrl Pts',(-1.94956209011008,-0.649003250612513,
9.8317748511156));
#49805=CARTESIAN_POINT('Ctrl Pts',(-1.9717826685226,-0.582254128397057,
9.82797418915372));
#49806=CARTESIAN_POINT('Ctrl Pts',(-1.99056476797815,-0.514381463802514,
9.82417352719185));
#49807=CARTESIAN_POINT('Ctrl Pts',(-2.00581132846463,-0.44577850677547,
9.82037286522998));
#49808=CARTESIAN_POINT('Ctrl Pts',(-2.02106384368285,-0.377148756019672,
9.81657071887282));
#49809=CARTESIAN_POINT('Ctrl Pts',(-2.03277798733833,-0.30778863949544,
9.81276857251567));
#49810=CARTESIAN_POINT('Ctrl Pts',(-2.04090813970047,-0.238099827392568,
9.80896642615852));
#49811=CARTESIAN_POINT('Ctrl Pts',(-2.04904829932559,-0.168325236544232,
9.80515959980561));
#49812=CARTESIAN_POINT('Ctrl Pts',(-2.05359564008046,-0.0982216428501038,
9.80135277345271));
#49813=CARTESIAN_POINT('Ctrl Pts',(-2.05455657900118,-0.0281926618634648,
9.7975459470998));
#49814=CARTESIAN_POINT('Ctrl Pts',(-2.05469294469403,-0.0182549329345308,
9.79700572492547));
#49815=CARTESIAN_POINT('Ctrl Pts',(-2.05475717252371,-0.0083187000115196,
9.79646550275115));
#49816=CARTESIAN_POINT('Ctrl Pts',(-2.0547493654031,0.00161489181494824,
9.79592528057682));
#49817=CARTESIAN_POINT('Ctrl Pts',(-2.05474936540253,0.00161489253451075,
9.79592528053768));
#49818=CARTESIAN_POINT('Ctrl Pts',(-2.05466554911524,0.108260665819365,
9.79012552426279));
#49819=CARTESIAN_POINT('Ctrl Pts',(-2.04627725539838,0.214587344483438,
9.7843257679879));
#49820=CARTESIAN_POINT('Ctrl Pts',(-2.02974241605634,0.319598634167586,
9.77852601171301));
#49821=CARTESIAN_POINT('Ctrl Pts',(-2.01871183817646,0.389652850308721,
9.77465692886612));
#49822=CARTESIAN_POINT('Ctrl Pts',(-2.00402863742738,0.45927254399467,9.77078784601923));
#49823=CARTESIAN_POINT('Ctrl Pts',(-1.98573997994474,0.528047625265998,
9.76691876317234));
#49824=CARTESIAN_POINT('Ctrl Pts',(-1.96747857164965,0.596720235096198,
9.76305544506593));
#49825=CARTESIAN_POINT('Ctrl Pts',(-1.9456224936184,0.664550264817994,9.75919212695952));
#49826=CARTESIAN_POINT('Ctrl Pts',(-1.92027026428373,0.731135879715741,
9.75532880885311));
#49827=CARTESIAN_POINT('Ctrl Pts',(-1.8949477731043,0.797643389712853,9.75147002241735));
#49828=CARTESIAN_POINT('Ctrl Pts',(-1.86613744858043,0.862908932554423,
9.7476112359816));
#49829=CARTESIAN_POINT('Ctrl Pts',(-1.83398765757475,0.926545646130553,
9.74375244954584));
#49830=CARTESIAN_POINT('Ctrl Pts',(-1.80185811857994,0.990142273243446,
9.73989609386258));
#49831=CARTESIAN_POINT('Ctrl Pts',(-1.76639350518624,1.05211167417853,9.73603973817932));
#49832=CARTESIAN_POINT('Ctrl Pts',(-1.7277897680421,1.11208816194986,9.73218338249606));
#49833=CARTESIAN_POINT('Ctrl Pts',(-1.6891974348285,1.17204693206609,9.72832816601889));
#49834=CARTESIAN_POINT('Ctrl Pts',(-1.64746808164534,1.23001354954329,9.72447294954172));
#49835=CARTESIAN_POINT('Ctrl Pts',(-1.60284207001888,1.28564958720391,9.72061773306455));
#49836=CARTESIAN_POINT('Ctrl Pts',(-1.55821431364881,1.34128780006724,9.71676236585994));
#49837=CARTESIAN_POINT('Ctrl Pts',(-1.51068997966217,1.39459487464493,9.71290699865533));
#49838=CARTESIAN_POINT('Ctrl Pts',(-1.46054987438482,1.44526524449129,9.70905163145072));
#49839=CARTESIAN_POINT('Ctrl Pts',(-1.41035728608979,1.49598865239775,9.70519222872796));
#49840=CARTESIAN_POINT('Ctrl Pts',(-1.35754380323296,1.54406950016236,9.7013328260052));
#49841=CARTESIAN_POINT('Ctrl Pts',(-1.3024266418318,1.58923956820447,9.69747342328243));
#49842=CARTESIAN_POINT('Ctrl Pts',(-1.2472782726609,1.63443521189393,9.69361183533553));
#49843=CARTESIAN_POINT('Ctrl Pts',(-1.18982401980682,1.6767165069229,9.68975024738863));
#49844=CARTESIAN_POINT('Ctrl Pts',(-1.13041146921395,1.71585764933154,9.68588865944173));
#49845=CARTESIAN_POINT('Ctrl Pts',(-1.07089497423428,1.75506727057177,9.6820203155083));
#49846=CARTESIAN_POINT('Ctrl Pts',(-1.00941376035066,1.79112552480892,9.67815197157487));
#49847=CARTESIAN_POINT('Ctrl Pts',(-0.94634084619215,1.82385212265916,9.67428362764144));
#49848=CARTESIAN_POINT('Ctrl Pts',(-0.908889964841267,1.84328423467522,
9.67198671633478));
#49849=CARTESIAN_POINT('Ctrl Pts',(-0.870878325287496,1.86154263115638,
9.66968980502811));
#49850=CARTESIAN_POINT('Ctrl Pts',(-0.832386957370501,1.87859775250038,
9.66739289372144));
#49851=CARTESIAN_POINT('Ctrl Pts',(-0.767549324792952,1.90732662733934,
9.66352381087445));
#49852=CARTESIAN_POINT('Ctrl Pts',(-0.701095638141634,1.9327511364569,9.65965472802746));
#49853=CARTESIAN_POINT('Ctrl Pts',(-0.633396009540079,1.95468848096025,
9.65578564518046));
#49854=CARTESIAN_POINT('Ctrl Pts',(-0.565797250008816,1.97659313991436,
9.65192232707395));
#49855=CARTESIAN_POINT('Ctrl Pts',(-0.496956691774747,1.9950207990505,9.64805900896744));
#49856=CARTESIAN_POINT('Ctrl Pts',(-0.427265363933371,2.00983627972103,
9.64419569086093));
#49857=CARTESIAN_POINT('Ctrl Pts',(-0.357655783992714,2.02463438183845,
9.64033690442507));
#49858=CARTESIAN_POINT('Ctrl Pts',(-0.287197889574732,2.03582862124997,
9.63647811798921));
#49859=CARTESIAN_POINT('Ctrl Pts',(-0.216297167600942,2.0433338194695,9.63261933155335));
#49860=CARTESIAN_POINT('Ctrl Pts',(-0.145441107883076,2.05083428996448,
9.62876297586999));
#49861=CARTESIAN_POINT('Ctrl Pts',(-0.0741432559817849,2.0546502786848,
9.62490662018664));
#49862=CARTESIAN_POINT('Ctrl Pts',(-0.00281711740553753,2.0547480688273,
9.62105026450328));
#49863=CARTESIAN_POINT('Ctrl Pts',(0.0684879507151712,2.05484583008161,
9.61719504802601));
#49864=CARTESIAN_POINT('Ctrl Pts',(0.139820803403486,2.05122757270765,9.61333983154874));
#49865=CARTESIAN_POINT('Ctrl Pts',(0.21076674943155,2.04391167613331,9.60948461507146));
#49866=CARTESIAN_POINT('Ctrl Pts',(0.281715469233902,2.03659549352929,9.60562924786676));
#49867=CARTESIAN_POINT('Ctrl Pts',(0.352276769348831,2.02558143672748,9.60177388066205));
#49868=CARTESIAN_POINT('Ctrl Pts',(0.422041629472952,2.01093968718403,9.59791851345734));
#49869=CARTESIAN_POINT('Ctrl Pts',(0.491879514381641,1.99628261172143,9.59405911073448));
#49870=CARTESIAN_POINT('Ctrl Pts',(0.560918818736848,1.97799036342823,9.59019970801162));
#49871=CARTESIAN_POINT('Ctrl Pts',(0.62876215067166,1.95618396895148,9.58634030528876));
#49872=CARTESIAN_POINT('Ctrl Pts',(0.696643896033928,1.93436522752288,9.58247871734177));
#49873=CARTESIAN_POINT('Ctrl Pts',(0.763327866616845,1.9090285515789,9.57861712939477));
#49874=CARTESIAN_POINT('Ctrl Pts',(0.828435833268841,1.88034348794473,9.57475554144777));
#49875=CARTESIAN_POINT('Ctrl Pts',(0.893657708642155,1.85160823876358,9.57088719751425));
#49876=CARTESIAN_POINT('Ctrl Pts',(0.957297641224268,1.8195131247985,9.56701885358073));
#49877=CARTESIAN_POINT('Ctrl Pts',(1.01900184597678,1.78427374592463,9.5631505096472));
#49878=CARTESIAN_POINT('Ctrl Pts',(1.05564002705512,1.76334961685681,9.56085359834143));
#49879=CARTESIAN_POINT('Ctrl Pts',(1.09159627510292,1.74131777606738,9.55855668703566));
#49880=CARTESIAN_POINT('Ctrl Pts',(1.12680180713025,1.71823026685832,9.55625977572989));
#49881=CARTESIAN_POINT('Ctrl Pts',(1.16958951638453,1.69017042584594,9.55346818112885));
#49882=CARTESIAN_POINT('Ctrl Pts',(1.21138883555603,1.66047175427513,9.55067658652781));
#49883=CARTESIAN_POINT('Ctrl Pts',(1.25206542099588,1.62921138715834,9.54788499192677));
#49884=CARTESIAN_POINT('',(-2.05474925034019,-0.0017551998270615,9.85407473953553));
#49885=CARTESIAN_POINT('Ctrl Pts',(-2.05341023593874,-0.00175368529942944,
9.85407471946233));
#49886=CARTESIAN_POINT('Ctrl Pts',(-2.04952255586939,0.476750142715482,
9.82816558982444));
#49887=CARTESIAN_POINT('Ctrl Pts',(-1.64442914339024,1.64534304864115,9.76521208752269));
#49888=CARTESIAN_POINT('Ctrl Pts',(-0.0359990651139381,2.27726163037769,
9.68255192549311));
#49889=CARTESIAN_POINT('Ctrl Pts',(0.960392961764501,1.84839376068804,9.6258008931014));
#49890=CARTESIAN_POINT('Ctrl Pts',(1.25005255340789,1.62658210076147,9.60609423337355));
#49891=CARTESIAN_POINT('Ctrl Pts',(1.25206542099588,1.62921138715834,10.3060095422728));
#49892=CARTESIAN_POINT('Ctrl Pts',(1.30851140146314,1.58583208054759,10.3021514635839));
#49893=CARTESIAN_POINT('Ctrl Pts',(1.36275851760942,1.53947116858342,10.2982933848949));
#49894=CARTESIAN_POINT('Ctrl Pts',(1.41448006564251,1.49038374467785,10.294435306206));
#49895=CARTESIAN_POINT('Ctrl Pts',(1.46617322566471,1.44132326301158,10.2905793450712));
#49896=CARTESIAN_POINT('Ctrl Pts',(1.51534321631979,1.38953957251344,10.2867233839364));
#49897=CARTESIAN_POINT('Ctrl Pts',(1.56169756025049,1.33532703590081,10.2828674228016));
#49898=CARTESIAN_POINT('Ctrl Pts',(1.60804196821539,1.28112611964272,10.2790122881848));
#49899=CARTESIAN_POINT('Ctrl Pts',(1.65157161248229,1.22449776034556,10.275157153568));
#49900=CARTESIAN_POINT('Ctrl Pts',(1.69203312206044,1.16577076492353,10.2713020189511));
#49901=CARTESIAN_POINT('Ctrl Pts',(1.73249949335545,1.10703671306623,10.2674464211145));
#49902=CARTESIAN_POINT('Ctrl Pts',(1.7698967246232,1.04620392594292,10.2635908232779));
#49903=CARTESIAN_POINT('Ctrl Pts',(1.80401473488021,0.983630214478525,10.2597352254412));
#49904=CARTESIAN_POINT('Ctrl Pts',(1.83817015564835,0.920987890732478,10.2558753999288));
#49905=CARTESIAN_POINT('Ctrl Pts',(1.86903894831024,0.856601261111506,10.2520155744164));
#49906=CARTESIAN_POINT('Ctrl Pts',(1.89645743256838,0.790851926062102,10.248155748904));
#49907=CARTESIAN_POINT('Ctrl Pts',(1.92389343440825,0.725060583973251,10.2442934573614));
#49908=CARTESIAN_POINT('Ctrl Pts',(1.94787457831404,0.657905261353421,10.2404311658188));
#49909=CARTESIAN_POINT('Ctrl Pts',(1.9682866322125,0.589784109614337,10.2365688742763));
#49910=CARTESIAN_POINT('Ctrl Pts',(1.98873291175794,0.52154873661644,10.2327001066864));
#49911=CARTESIAN_POINT('Ctrl Pts',(2.00559804624542,0.452344774535711,10.2288313390965));
#49912=CARTESIAN_POINT('Ctrl Pts',(2.01881877631864,0.38258111673645,10.2249625715066));
#49913=CARTESIAN_POINT('Ctrl Pts',(2.02346945516632,0.358040235418474,10.2236016485094));
#49914=CARTESIAN_POINT('Ctrl Pts',(2.02766963312196,0.33343014000644,10.2222407255122));
#49915=CARTESIAN_POINT('Ctrl Pts',(2.03141808692682,0.308768713775479,10.2208798025149));
#49916=CARTESIAN_POINT('Ctrl Pts',(2.04207488260764,0.23865666378834,10.217010719668));
#49917=CARTESIAN_POINT('Ctrl Pts',(2.04911853507526,0.167854932925696,10.2131416368211));
#49918=CARTESIAN_POINT('Ctrl Pts',(2.05247006878331,0.0967686894023167,
10.2092725539742));
#49919=CARTESIAN_POINT('Ctrl Pts',(2.05581660887328,0.0257883608366547,
10.2054092358677));
#49920=CARTESIAN_POINT('Ctrl Pts',(2.05548192698947,-0.0454751576497036,
10.2015459177613));
#49921=CARTESIAN_POINT('Ctrl Pts',(2.05143849348082,-0.116609047526893,
10.1976825996549));
#49922=CARTESIAN_POINT('Ctrl Pts',(2.04739980291812,-0.187659497378737,
10.1938238132191));
#49923=CARTESIAN_POINT('Ctrl Pts',(2.0396610294618,-0.258580138006337,10.1899650267833));
#49924=CARTESIAN_POINT('Ctrl Pts',(2.02824668591195,-0.328957358311389,
10.1861062403475));
#49925=CARTESIAN_POINT('Ctrl Pts',(2.01683953256154,-0.399290246128239,
10.1822498846642));
#49926=CARTESIAN_POINT('Ctrl Pts',(2.00176148030334,-0.469079914386366,
10.178393528981));
#49927=CARTESIAN_POINT('Ctrl Pts',(1.98308880014757,-0.53791855631617,10.1745371732977));
#49928=CARTESIAN_POINT('Ctrl Pts',(1.9644216360885,-0.606736862621825,10.1706819568205));
#49929=CARTESIAN_POINT('Ctrl Pts',(1.94216207938165,-0.674604231762789,
10.1668267403433));
#49930=CARTESIAN_POINT('Ctrl Pts',(1.91643697360225,-0.741125420364361,
10.1629715238661));
#49931=CARTESIAN_POINT('Ctrl Pts',(1.89071086204816,-0.807649209745421,
10.1591161566615));
#49932=CARTESIAN_POINT('Ctrl Pts',(1.86151910968989,-0.872826261805287,
10.1552607894568));
#49933=CARTESIAN_POINT('Ctrl Pts',(1.82903704474084,-0.936280434199973,
10.1514054222522));
#49934=CARTESIAN_POINT('Ctrl Pts',(1.79652097992722,-0.999801025810044,
10.1475460195294));
#49935=CARTESIAN_POINT('Ctrl Pts',(1.76070794921565,-1.06159470448789,10.1436866168066));
#49936=CARTESIAN_POINT('Ctrl Pts',(1.72181927482045,-1.12130992475621,10.1398272140838));
#49937=CARTESIAN_POINT('Ctrl Pts',(1.68290858135236,-1.18105895625128,10.1359656261369));
#49938=CARTESIAN_POINT('Ctrl Pts',(1.64091906358225,-1.23872679371579,10.13210403819));
#49939=CARTESIAN_POINT('Ctrl Pts',(1.59611381224928,-1.29399314559509,10.1282424502431));
#49940=CARTESIAN_POINT('Ctrl Pts',(1.55123017252307,-1.349356187938,10.1243741063096));
#49941=CARTESIAN_POINT('Ctrl Pts',(1.50352128915094,-1.40230899529215,10.1205057623762));
#49942=CARTESIAN_POINT('Ctrl Pts',(1.45328825158113,-1.45256697618948,10.1166374184427));
#49943=CARTESIAN_POINT('Ctrl Pts',(1.42346131945304,-1.48240871894766,10.1143405071363));
#49944=CARTESIAN_POINT('Ctrl Pts',(1.39274513387088,-1.51130110075618,10.1120435958298));
#49945=CARTESIAN_POINT('Ctrl Pts',(1.36120800223661,-1.53919145565034,10.1097466845234));
#49946=CARTESIAN_POINT('Ctrl Pts',(1.30808458614967,-1.58617197832557,10.1058776016765));
#49947=CARTESIAN_POINT('Ctrl Pts',(1.25242204857328,-1.63049104920695,10.1020085188295));
#49948=CARTESIAN_POINT('Ctrl Pts',(1.19451794994457,-1.6718625630596,10.0981394359826));
#49949=CARTESIAN_POINT('Ctrl Pts',(1.13670012553504,-1.71317243541989,10.0942761178762));
#49950=CARTESIAN_POINT('Ctrl Pts',(1.07664776155301,-1.75154318807345,10.0904127997698));
#49951=CARTESIAN_POINT('Ctrl Pts',(1.01469274895957,-1.78672778780341,10.0865494816633));
#49952=CARTESIAN_POINT('Ctrl Pts',(0.952810409571998,-1.82187111601146,
10.0826906952275));
#49953=CARTESIAN_POINT('Ctrl Pts',(0.88903027506293,-1.85383547622168,10.0788319087917));
#49954=CARTESIAN_POINT('Ctrl Pts',(0.823713129057717,-1.88241712792833,
10.074973122356));
#49955=CARTESIAN_POINT('Ctrl Pts',(0.758437128065021,-1.91098077529019,
10.0711167666727));
#49956=CARTESIAN_POINT('Ctrl Pts',(0.691626480467066,-1.93616574745647,
10.0672604109894));
#49957=CARTESIAN_POINT('Ctrl Pts',(0.623665166115261,-1.95781493585947,
10.0634040553061));
#49958=CARTESIAN_POINT('Ctrl Pts',(0.555723928216199,-1.97945772887545,
10.0595488388289));
#49959=CARTESIAN_POINT('Ctrl Pts',(0.486633161009463,-1.99756666439603,
10.0556936223517));
#49960=CARTESIAN_POINT('Ctrl Pts',(0.416793718986835,-2.01203393567632,
10.0518384058745));
#49961=CARTESIAN_POINT('Ctrl Pts',(0.346951546450887,-2.02650177258365,
10.0479830386699));
#49962=CARTESIAN_POINT('Ctrl Pts',(0.276361117116424,-2.03732756619642,
10.0441276714652));
#49963=CARTESIAN_POINT('Ctrl Pts',(0.205433535181078,-2.0444546033412,10.0402723042606));
#49964=CARTESIAN_POINT('Ctrl Pts',(0.134431711408507,-2.05158910055041,
10.0364129015378));
#49965=CARTESIAN_POINT('Ctrl Pts',(0.0630925148932319,-2.05501706406355,
10.032553498815));
#49966=CARTESIAN_POINT('Ctrl Pts',(-0.00816866856745738,-2.05473376264513,
10.0286940960922));
#49967=CARTESIAN_POINT('Ctrl Pts',(-0.0794702006701796,-2.05445030081923,
10.0248325081453));
#49968=CARTESIAN_POINT('Ctrl Pts',(-0.15069314653743,-2.05045141817204,
10.0209709201983));
#49969=CARTESIAN_POINT('Ctrl Pts',(-0.221425723400285,-2.04278442609999,
10.0171093322514));
#49970=CARTESIAN_POINT('Ctrl Pts',(-0.292282049441501,-2.03510402035051,
10.013240988318));
#49971=CARTESIAN_POINT('Ctrl Pts',(-0.362645813896895,-2.02374276993654,
10.0093726443845));
#49972=CARTESIAN_POINT('Ctrl Pts',(-0.432114617069166,-2.00879927325135,
10.005504300451));
#49973=CARTESIAN_POINT('Ctrl Pts',(-0.473363193254439,-1.99992625495615,
10.0032073891446));
#49974=CARTESIAN_POINT('Ctrl Pts',(-0.514296493476365,-1.9897912307239,
10.0009104778382));
#49975=CARTESIAN_POINT('Ctrl Pts',(-0.5548332227254,-1.97842302287962,9.99861356653179));
#49976=CARTESIAN_POINT('Ctrl Pts',(-0.623116209259948,-1.95927359475523,
9.99474448368487));
#49977=CARTESIAN_POINT('Ctrl Pts',(-0.690540391634209,-1.93654744760311,
9.99087540083796));
#49978=CARTESIAN_POINT('Ctrl Pts',(-0.756704012451471,-1.91033939394021,
9.98700631799105));
#49979=CARTESIAN_POINT('Ctrl Pts',(-0.822769052773433,-1.88417038897021,
9.98314299988462));
#49980=CARTESIAN_POINT('Ctrl Pts',(-0.887576811699232,-1.8545299527043,
9.97927968177818));
#49981=CARTESIAN_POINT('Ctrl Pts',(-0.950739737326332,-1.8215629317618,
9.97541636367175));
#49982=CARTESIAN_POINT('Ctrl Pts',(-1.0138285728661,-1.78863458112212,9.97155757723597));
#49983=CARTESIAN_POINT('Ctrl Pts',(-1.07527597896355,-1.7523876203456,9.96769879080019));
#49984=CARTESIAN_POINT('Ctrl Pts',(-1.13471510454231,-1.71301465084906,
9.96384000436441));
#49985=CARTESIAN_POINT('Ctrl Pts',(-1.19411678783038,-1.67366648343625,
9.95998364868113));
#49986=CARTESIAN_POINT('Ctrl Pts',(-1.25151229644495,-1.63119648171335,
9.95612729299785));
#49987=CARTESIAN_POINT('Ctrl Pts',(-1.30656137516673,-1.58584202725947,
9.95227093731457));
#49988=CARTESIAN_POINT('Ctrl Pts',(-1.36159419183955,-1.54050097096548,
9.94841572083736));
#49989=CARTESIAN_POINT('Ctrl Pts',(-1.41428158001253,-1.49227746231644,
9.94456050436016));
#49990=CARTESIAN_POINT('Ctrl Pts',(-1.46431555208567,-1.44144980017343,
9.94070528788295));
#49991=CARTESIAN_POINT('Ctrl Pts',(-1.51435148033746,-1.39062015082088,
9.93684992067832));
#49992=CARTESIAN_POINT('Ctrl Pts',(-1.56173344730898,-1.33718649357301,
9.93299455347368));
#49993=CARTESIAN_POINT('Ctrl Pts',(-1.60619083156095,-1.28146345055548,
9.92913918626905));
#49994=CARTESIAN_POINT('Ctrl Pts',(-1.65069475057122,-1.22568208070693,
9.92527978354626));
#49995=CARTESIAN_POINT('Ctrl Pts',(-1.69226767235597,-1.16760692192484,
9.92142038082348));
#49996=CARTESIAN_POINT('Ctrl Pts',(-1.73068032496605,-1.10758438742852,
9.91756097810069));
#49997=CARTESIAN_POINT('Ctrl Pts',(-1.76911472712186,-1.04752786770153,
9.91369939015376));
#49998=CARTESIAN_POINT('Ctrl Pts',(-1.80438505772054,-0.985522199735724,
9.90983780220683));
#49999=CARTESIAN_POINT('Ctrl Pts',(-1.8363077217611,-0.921938996626441,
9.9059762142599));
#50000=CARTESIAN_POINT('Ctrl Pts',(-1.86828623564657,-0.858244552424377,
9.90210787032644));
#50001=CARTESIAN_POINT('Ctrl Pts',(-1.89690519446484,-0.792967507795669,
9.89823952639299));
#50002=CARTESIAN_POINT('Ctrl Pts',(-1.92202918031085,-0.726499409864598,
9.89437118245954));
#50003=CARTESIAN_POINT('Ctrl Pts',(-1.93694708010085,-0.687032566098429,
9.8920742711531));
#50004=CARTESIAN_POINT('Ctrl Pts',(-1.95063372748089,-0.647146108913449,
9.88977735984666));
#50005=CARTESIAN_POINT('Ctrl Pts',(-1.96306924422631,-0.606923969598107,
9.88748044854022));
#50006=CARTESIAN_POINT('Ctrl Pts',(-1.98856453961245,-0.524460542954842,
9.88277132117284));
#50007=CARTESIAN_POINT('Ctrl Pts',(-2.00887960280738,-0.440324787035022,
9.87806219380546));
#50008=CARTESIAN_POINT('Ctrl Pts',(-2.02383211662245,-0.355107203851881,
9.87335306643807));
#50009=CARTESIAN_POINT('Ctrl Pts',(-2.03858220171866,-0.27104330535358,
9.86870769173674));
#50010=CARTESIAN_POINT('Ctrl Pts',(-2.04811390579993,-0.185926671662672,
9.86406231703542));
#50011=CARTESIAN_POINT('Ctrl Pts',(-2.05229833310357,-0.100344977155406,
9.85941694233409));
#50012=CARTESIAN_POINT('Ctrl Pts',(-2.05390237014321,-0.0675385264886835,
9.8576362080679));
#50013=CARTESIAN_POINT('Ctrl Pts',(-2.0547211391509,-0.0346639571255305,
9.85585547380171));
#50014=CARTESIAN_POINT('Ctrl Pts',(-2.05474925034019,-0.0017551998270615,
9.85407473953553));
#50015=CARTESIAN_POINT('Origin',(0.,0.,18.5459252805377));
#50016=CARTESIAN_POINT('',(1.25206542099588,1.62921138715834,11.006111809188));
#50017=CARTESIAN_POINT('',(1.2500265821584,1.62656556227503,10.9479122870705));
#50018=CARTESIAN_POINT('',(1.25206542099588,1.62921138715835,18.5459252805377));
#50019=CARTESIAN_POINT('',(-2.05447077626017,0.000498338557913886,10.4959252565846));
#50020=CARTESIAN_POINT('Ctrl Pts',(1.2500265821584,1.62656556227503,10.9479122870705));
#50021=CARTESIAN_POINT('Ctrl Pts',(1.53383714851955,1.40790651594786,10.9285605885899));
#50022=CARTESIAN_POINT('Ctrl Pts',(2.20363273241515,0.565166268200534,10.8721645174454));
#50023=CARTESIAN_POINT('Ctrl Pts',(1.99999618452663,-1.37767715104267,10.778724073637));
#50024=CARTESIAN_POINT('Ctrl Pts',(-0.0726735740554304,-2.42748792422539,
10.6675909556455));
#50025=CARTESIAN_POINT('Ctrl Pts',(-1.77435205970044,-1.43343066499739,
10.573324691279));
#50026=CARTESIAN_POINT('Ctrl Pts',(-2.05068411161783,-0.373027881039349,
10.5161027995764));
#50027=CARTESIAN_POINT('Ctrl Pts',(-2.05149284387169,0.000497172743597965,
10.4959252805377));
#50028=CARTESIAN_POINT('Ctrl Pts',(-2.05474993954246,0.000498447846006602,
10.4959252543392));
#50029=CARTESIAN_POINT('Ctrl Pts',(-2.05473097356229,0.0786818464106275,
10.4917085431161));
#50030=CARTESIAN_POINT('Ctrl Pts',(-2.05024504110033,0.156745944516384,
10.487491831893));
#50031=CARTESIAN_POINT('Ctrl Pts',(-2.04136052314416,0.234189617721592,
10.48327512067));
#50032=CARTESIAN_POINT('Ctrl Pts',(-2.03264332173962,0.310174842825331,
10.4791378201234));
#50033=CARTESIAN_POINT('Ctrl Pts',(-2.01969195736155,0.385562469206602,
10.4750005195768));
#50034=CARTESIAN_POINT('Ctrl Pts',(-2.00262219642564,0.459893358163985,
10.4708632190302));
#50035=CARTESIAN_POINT('Ctrl Pts',(-1.98506098415044,0.536364289683557,
10.4666068024689));
#50036=CARTESIAN_POINT('Ctrl Pts',(-1.96314076623114,0.611716290701171,
10.4623503859076));
#50037=CARTESIAN_POINT('Ctrl Pts',(-1.93704088653234,0.685470762616473,
10.4580939693463));
#50038=CARTESIAN_POINT('Ctrl Pts',(-1.91094100683353,0.759225234531785,
10.453837552785));
#50039=CARTESIAN_POINT('Ctrl Pts',(-1.88066170729429,0.831381822486739,
10.4495811362237));
#50040=CARTESIAN_POINT('Ctrl Pts',(-1.84643304563615,0.901489085060272,
10.4453247196624));
#50041=CARTESIAN_POINT('Ctrl Pts',(-1.8153191906393,0.965216589913511,10.4414556368155));
#50042=CARTESIAN_POINT('Ctrl Pts',(-1.78084130052563,1.02745623344192,10.4375865539685));
#50043=CARTESIAN_POINT('Ctrl Pts',(-1.74316487402478,1.08782985088026,10.4337174711216));
#50044=CARTESIAN_POINT('Ctrl Pts',(-1.70554458352043,1.14811351463955,10.4298541530152));
#50045=CARTESIAN_POINT('Ctrl Pts',(-1.66473547142074,1.20653626233826,10.4259908349087));
#50046=CARTESIAN_POINT('Ctrl Pts',(-1.62094970129442,1.26274289876187,10.4221275168023));
#50047=CARTESIAN_POINT('Ctrl Pts',(-1.57721529185957,1.31888360482263,10.4182687303665));
#50048=CARTESIAN_POINT('Ctrl Pts',(-1.53051145702339,1.37281298172646,10.4144099439307));
#50049=CARTESIAN_POINT('Ctrl Pts',(-1.48109361524659,1.42420478351106,10.4105511574949));
#50050=CARTESIAN_POINT('Ctrl Pts',(-1.43170690308646,1.47556421222893,10.4066948018117));
#50051=CARTESIAN_POINT('Ctrl Pts',(-1.37960991176963,1.52438888786751,10.4028384461284));
#50052=CARTESIAN_POINT('Ctrl Pts',(-1.32509732862853,1.57038677788675,10.3989820904451));
#50053=CARTESIAN_POINT('Ctrl Pts',(-1.27060084905034,1.6163710796687,10.3951268739679));
#50054=CARTESIAN_POINT('Ctrl Pts',(-1.21369056539008,1.65952994055047,10.3912716574907));
#50055=CARTESIAN_POINT('Ctrl Pts',(-1.15469561420114,1.69961042625792,10.3874164410135));
#50056=CARTESIAN_POINT('Ctrl Pts',(-1.09569835648608,1.73969247899248,10.3835610738089));
#50057=CARTESIAN_POINT('Ctrl Pts',(-1.03461667248542,1.77669564643269,10.3797057066042));
#50058=CARTESIAN_POINT('Ctrl Pts',(-0.971808712157427,1.81041028208385,
10.3758503393996));
#50059=CARTESIAN_POINT('Ctrl Pts',(-0.908935009021874,1.84416020776501,
10.3719909366768));
#50060=CARTESIAN_POINT('Ctrl Pts',(-0.84433185139397,1.87461450003715,10.368131533954));
#50061=CARTESIAN_POINT('Ctrl Pts',(-0.778381228161229,1.90160990377791,
10.3642721312312));
#50062=CARTESIAN_POINT('Ctrl Pts',(-0.712393263167531,1.92862059252832,
10.3604105432843));
#50063=CARTESIAN_POINT('Ctrl Pts',(-0.64505677254964,1.95216833364465,10.3565489553374));
#50064=CARTESIAN_POINT('Ctrl Pts',(-0.576770322283165,1.97213933529895,
10.3526873673904));
#50065=CARTESIAN_POINT('Ctrl Pts',(-0.508364402424352,1.99214527693647,
10.348819023457));
#50066=CARTESIAN_POINT('Ctrl Pts',(-0.439005677581511,2.00856187364456,
10.3449506795235));
#50067=CARTESIAN_POINT('Ctrl Pts',(-0.369103661279685,2.02132630956259,
10.3410823355901));
#50068=CARTESIAN_POINT('Ctrl Pts',(-0.327597855604687,2.02890546428221,
10.3387854242837));
#50069=CARTESIAN_POINT('Ctrl Pts',(-0.285900638318682,2.03519798793061,
10.3364885129772));
#50070=CARTESIAN_POINT('Ctrl Pts',(-0.244098146947801,2.04019941602694,
10.3341916016708));
#50071=CARTESIAN_POINT('Ctrl Pts',(-0.173703126748368,2.04862177604236,
10.3303236236506));
#50072=CARTESIAN_POINT('Ctrl Pts',(-0.102733850231292,2.05341298926354,
10.3264556456304));
#50073=CARTESIAN_POINT('Ctrl Pts',(-0.0315974388829441,2.0545070368232,
10.3225876676102));
#50074=CARTESIAN_POINT('Ctrl Pts',(0.0394421200313115,2.05559959483387,
10.3187249558535));
#50075=CARTESIAN_POINT('Ctrl Pts',(0.110647881218013,2.05300496468608,10.3148622440967));
#50076=CARTESIAN_POINT('Ctrl Pts',(0.181606556230323,2.04670872896809,10.31099953234));
#50077=CARTESIAN_POINT('Ctrl Pts',(0.252492365379201,2.04041895871259,10.3071407871149));
#50078=CARTESIAN_POINT('Ctrl Pts',(0.323131110541038,2.0304351683889,10.3032820418898));
#50079=CARTESIAN_POINT('Ctrl Pts',(0.393110179594325,2.01679496954929,10.2994232966647));
#50080=CARTESIAN_POINT('Ctrl Pts',(0.463040801360492,2.0031642139709,10.2955672228918));
#50081=CARTESIAN_POINT('Ctrl Pts',(0.532312178227357,1.98588216865933,10.2917111491189));
#50082=CARTESIAN_POINT('Ctrl Pts',(0.600519215173281,1.96503797284115,10.287855075346));
#50083=CARTESIAN_POINT('Ctrl Pts',(0.668720126930718,1.94419564889183,10.2839993478596));
#50084=CARTESIAN_POINT('Ctrl Pts',(0.735856420422147,1.91979193921891,10.2801436203733));
#50085=CARTESIAN_POINT('Ctrl Pts',(0.801536916561915,1.89196620844253,10.2762878928869));
#50086=CARTESIAN_POINT('Ctrl Pts',(0.86721356021688,1.8641421097824,10.2724323915579));
#50087=CARTESIAN_POINT('Ctrl Pts',(0.931434131880338,1.8328965857645,10.268576890229));
#50088=CARTESIAN_POINT('Ctrl Pts',(0.993828199404314,1.79841682392286,10.2647213889001));
#50089=CARTESIAN_POINT('Ctrl Pts',(1.05626662864416,1.76391254722814,10.2608631463385));
#50090=CARTESIAN_POINT('Ctrl Pts',(1.11687554065305,1.72616968602744,10.2570049037769));
#50091=CARTESIAN_POINT('Ctrl Pts',(1.17531089106955,1.68542038430574,10.2531466612153));
#50092=CARTESIAN_POINT('Ctrl Pts',(1.20133590805387,1.6672721014282,10.2514283378463));
#50093=CARTESIAN_POINT('Ctrl Pts',(1.22693019820243,1.64852805997119,10.2497100144773));
#50094=CARTESIAN_POINT('Ctrl Pts',(1.25206542099587,1.62921138715835,10.2479916911084));
#50095=CARTESIAN_POINT('',(-2.05474999986746,-2.33377752992841E-5,10.5540747194726));
#50096=CARTESIAN_POINT('Ctrl Pts',(-2.05474999986747,-2.33375873728629E-5,
10.5540747194623));
#50097=CARTESIAN_POINT('Ctrl Pts',(-2.05475080507059,0.0708704990450557,
10.5502069203748));
#50098=CARTESIAN_POINT('Ctrl Pts',(-2.05107828913696,0.141903688300347,
10.5463391212873));
#50099=CARTESIAN_POINT('Ctrl Pts',(-2.04371513948629,0.212664033476554,
10.5424713221998));
#50100=CARTESIAN_POINT('Ctrl Pts',(-2.03636296193386,0.283318936077959,
10.538609286661));
#50101=CARTESIAN_POINT('Ctrl Pts',(-2.02533111680999,0.353701322035903,
10.5347472511222));
#50102=CARTESIAN_POINT('Ctrl Pts',(-2.01065430302448,0.423399145286292,
10.5308852155834));
#50103=CARTESIAN_POINT('Ctrl Pts',(-1.99599469219053,0.493015274492245,
10.5270277068044));
#50104=CARTESIAN_POINT('Ctrl Pts',(-1.97769869852177,0.561947961368902,
10.5231701980254));
#50105=CARTESIAN_POINT('Ctrl Pts',(-1.95585259333795,0.629792184480901,
10.5193126892464));
#50106=CARTESIAN_POINT('Ctrl Pts',(-1.93402022515182,0.697593746627546,
10.5154576060983));
#50107=CARTESIAN_POINT('Ctrl Pts',(-1.90864232294593,0.764307741231233,
10.5116025229502));
#50108=CARTESIAN_POINT('Ctrl Pts',(-1.8798554581763,0.829542656446767,10.5077474398022));
#50109=CARTESIAN_POINT('Ctrl Pts',(-1.85107704745796,0.89475841364273,10.5038934888049));
#50110=CARTESIAN_POINT('Ctrl Pts',(-1.8188918578528,0.958495509261486,10.5000395378076));
#50111=CARTESIAN_POINT('Ctrl Pts',(-1.78348457188773,1.02038245003452,10.4961855868103));
#50112=CARTESIAN_POINT('Ctrl Pts',(-1.74807581851152,1.08227195563519,10.4923314760907));
#50113=CARTESIAN_POINT('Ctrl Pts',(-1.70944494702554,1.14231073330303,10.4884773653712));
#50114=CARTESIAN_POINT('Ctrl Pts',(-1.66782170192874,1.20015346230202,10.4846232546517));
#50115=CARTESIAN_POINT('Ctrl Pts',(-1.62615484911945,1.25805679179216,10.4807651060694));
#50116=CARTESIAN_POINT('Ctrl Pts',(-1.58148964919704,1.31375908455404,10.4769069574871));
#50117=CARTESIAN_POINT('Ctrl Pts',(-1.53409761489166,1.3669462573502,10.4730488089047));
#50118=CARTESIAN_POINT('Ctrl Pts',(-1.48667859361788,1.42016371710434,10.4691884633344));
#50119=CARTESIAN_POINT('Ctrl Pts',(-1.43652998905314,1.47086286017553,10.465328117764));
#50120=CARTESIAN_POINT('Ctrl Pts',(-1.383959901113,1.51876678743357,10.4614677721936));
#50121=CARTESIAN_POINT('Ctrl Pts',(-1.33129808653137,1.56675429960717,10.4576006909196));
#50122=CARTESIAN_POINT('Ctrl Pts',(-1.27620672940096,1.61193655060224,10.4537336096455));
#50123=CARTESIAN_POINT('Ctrl Pts',(-1.21902610721736,1.65407766214966,10.4498665283715));
#50124=CARTESIAN_POINT('Ctrl Pts',(-1.18590191827414,1.67848960605422,10.4476263650803));
#50125=CARTESIAN_POINT('Ctrl Pts',(-1.15207715688745,1.70188182604525,10.4453862017892));
#50126=CARTESIAN_POINT('Ctrl Pts',(-1.11762181697521,1.72421548442213,10.443146038498));
#50127=CARTESIAN_POINT('Ctrl Pts',(-1.05811251014641,1.76278891113464,10.4392769556511));
#50128=CARTESIAN_POINT('Ctrl Pts',(-0.996487327073619,1.79835342918964,
10.4354078728042));
#50129=CARTESIAN_POINT('Ctrl Pts',(-0.933083005032195,1.83067027840081,
10.4315387899573));
#50130=CARTESIAN_POINT('Ctrl Pts',(-0.869773152268525,1.86293897711835,
10.4276754718508));
#50131=CARTESIAN_POINT('Ctrl Pts',(-0.804689851637586,1.89196939320252,
10.4238121537444));
#50132=CARTESIAN_POINT('Ctrl Pts',(-0.73819799003566,1.91756650210816,10.419948835638));
#50133=CARTESIAN_POINT('Ctrl Pts',(-0.671784123361779,1.94313358561491,
10.4160900492022));
#50134=CARTESIAN_POINT('Ctrl Pts',(-0.603965428777979,1.96527518778353,
10.4122312627664));
#50135=CARTESIAN_POINT('Ctrl Pts',(-0.535128938610543,1.98384338634922,
10.4083724763306));
#50136=CARTESIAN_POINT('Ctrl Pts',(-0.466335810384357,2.00239988831137,
10.4045161206473));
#50137=CARTESIAN_POINT('Ctrl Pts',(-0.396526626490185,2.01738732636825,
10.4006597649641));
#50138=CARTESIAN_POINT('Ctrl Pts',(-0.326104435639335,2.02870733708841,
10.3968034092808));
#50139=CARTESIAN_POINT('Ctrl Pts',(-0.255703048208796,2.04002400376405,
10.3929481928036));
#50140=CARTESIAN_POINT('Ctrl Pts',(-0.184689492697166,2.04767531688683,
10.3890929763264));
#50141=CARTESIAN_POINT('Ctrl Pts',(-0.113476186303622,2.05161417367935,
10.3852377598492));
#50142=CARTESIAN_POINT('Ctrl Pts',(-0.0422600956828595,2.05555318446937,
10.3813823926445));
#50143=CARTESIAN_POINT('Ctrl Pts',(0.0291552761615211,2.05577942613248,
10.3775270254399));
#50144=CARTESIAN_POINT('Ctrl Pts',(0.100354961062196,2.05229784492656,10.3736716582353));
#50145=CARTESIAN_POINT('Ctrl Pts',(0.171629172617799,2.0488126194545,10.3698122555125));
#50146=CARTESIAN_POINT('Ctrl Pts',(0.242686760353929,2.04161184738354,10.3659528527897));
#50147=CARTESIAN_POINT('Ctrl Pts',(0.313116238992187,2.03075251652667,10.3620934500669));
#50148=CARTESIAN_POINT('Ctrl Pts',(0.383585595354432,2.01988703703137,10.35823186212));
#50149=CARTESIAN_POINT('Ctrl Pts',(0.453425658821506,2.00535897400424,10.3543702741731));
#50150=CARTESIAN_POINT('Ctrl Pts',(0.522236233272553,1.98727624631235,10.3505086862261));
#50151=CARTESIAN_POINT('Ctrl Pts',(0.591167194290042,1.9691618822402,10.3466403422927));
#50152=CARTESIAN_POINT('Ctrl Pts',(0.659064607380088,1.94748058488558,10.3427719983592));
#50153=CARTESIAN_POINT('Ctrl Pts',(0.725545169395101,1.92238959882419,10.3389036544258));
#50154=CARTESIAN_POINT('Ctrl Pts',(0.765019413975448,1.90749129335671,10.3366067431193));
#50155=CARTESIAN_POINT('Ctrl Pts',(0.803994523493019,1.89139177096154,10.3343098318129));
#50156=CARTESIAN_POINT('Ctrl Pts',(0.842394382624847,1.87413160333582,10.3320129205065));
#50157=CARTESIAN_POINT('Ctrl Pts',(0.907080692986367,1.84505606542574,10.3281436688738));
#50158=CARTESIAN_POINT('Ctrl Pts',(0.970386608737807,1.81257063920744,10.3242744172411));
#50159=CARTESIAN_POINT('Ctrl Pts',(1.03192885009436,1.7768287511302,10.3204051656084));
#50160=CARTESIAN_POINT('Ctrl Pts',(1.09337296593308,1.74114385141087,10.316542083272));
#50161=CARTESIAN_POINT('Ctrl Pts',(1.15305857523068,1.70221304314449,10.3126790009356));
#50162=CARTESIAN_POINT('Ctrl Pts',(1.21062399045595,1.66023706627472,10.3088159185992));
#50163=CARTESIAN_POINT('Ctrl Pts',(1.22456365524853,1.6500724380059,10.3078804598238));
#50164=CARTESIAN_POINT('Ctrl Pts',(1.23837910404261,1.63972946009415,10.3069450010483));
#50165=CARTESIAN_POINT('Ctrl Pts',(1.25206542099588,1.62921138715834,10.3060095422728));
#50166=CARTESIAN_POINT('Ctrl Pts',(1.25206542099588,1.62921138715834,11.006111809188));
#50167=CARTESIAN_POINT('Ctrl Pts',(1.28751164932299,1.60197060235723,11.0036784156106));
#50168=CARTESIAN_POINT('Ctrl Pts',(1.32203066489551,1.57360155165411,11.0012450220332));
#50169=CARTESIAN_POINT('Ctrl Pts',(1.3555499459167,1.54417677311415,10.9988116284558));
#50170=CARTESIAN_POINT('Ctrl Pts',(1.40884542448033,1.49739153172055,10.9949425456089));
#50171=CARTESIAN_POINT('Ctrl Pts',(1.45982033721477,1.44775226898479,10.991073462762));
#50172=CARTESIAN_POINT('Ctrl Pts',(1.50815338956561,1.39551815324694,10.9872043799151));
#50173=CARTESIAN_POINT('Ctrl Pts',(1.55641442807892,1.34336186373652,10.9833410618086));
#50174=CARTESIAN_POINT('Ctrl Pts',(1.60204109229655,1.28861874917948,10.9794777437022));
#50175=CARTESIAN_POINT('Ctrl Pts',(1.64474652611685,1.23158695483777,10.9756144255958));
#50176=CARTESIAN_POINT('Ctrl Pts',(1.68740186647972,1.17462205876885,10.97175563916));
#50177=CARTESIAN_POINT('Ctrl Pts',(1.72714249307915,1.11537420244368,10.9678968527242));
#50178=CARTESIAN_POINT('Ctrl Pts',(1.76372086005815,1.05417564489781,10.9640380662884));
#50179=CARTESIAN_POINT('Ctrl Pts',(1.80027618534813,0.993015637955712,10.9601817106051));
#50180=CARTESIAN_POINT('Ctrl Pts',(1.8336729544594,0.929907783702804,10.9563253549218));
#50181=CARTESIAN_POINT('Ctrl Pts',(1.86370696167862,0.865213224292507,10.9524689992386));
#50182=CARTESIAN_POINT('Ctrl Pts',(1.89373209655137,0.800537776302861,10.9486137827614));
#50183=CARTESIAN_POINT('Ctrl Pts',(1.92039623725209,0.734276994088983,10.9447585662842));
#50184=CARTESIAN_POINT('Ctrl Pts',(1.94354196280814,0.666814967816328,10.940903349807));
#50185=CARTESIAN_POINT('Ctrl Pts',(1.96668859329283,0.599350303980218,10.9370479826023));
#50186=CARTESIAN_POINT('Ctrl Pts',(1.98631637996209,0.530684763048594,10.9331926153977));
#50187=CARTESIAN_POINT('Ctrl Pts',(2.00231729822874,0.461219036591021,10.9293372481931));
#50188=CARTESIAN_POINT('Ctrl Pts',(2.01833496509358,0.39168059846024,10.9254778454703));
#50189=CARTESIAN_POINT('Ctrl Pts',(2.0307180759414,0.321340777170848,10.9216184427475));
#50190=CARTESIAN_POINT('Ctrl Pts',(2.03940963532042,0.250611056943251,10.9177590400247));
#50191=CARTESIAN_POINT('Ctrl Pts',(2.04810611592864,0.179841288992474,10.9138974520778));
#50192=CARTESIAN_POINT('Ctrl Pts',(2.053106850083,0.108681667448183,10.9100358641309));
#50193=CARTESIAN_POINT('Ctrl Pts',(2.05440692444374,0.0375466549457377,
10.9061742761839));
#50194=CARTESIAN_POINT('Ctrl Pts',(2.05570927333117,-0.0337128108108279,
10.9023059322505));
#50195=CARTESIAN_POINT('Ctrl Pts',(2.05329805246777,-0.104947095907617,
10.898437588317));
#50196=CARTESIAN_POINT('Ctrl Pts',(2.04722040877868,-0.175744588480139,
10.8945692443836));
#50197=CARTESIAN_POINT('Ctrl Pts',(2.04361167885547,-0.217782102195106,
10.8922723330771));
#50198=CARTESIAN_POINT('Ctrl Pts',(2.03871128981978,-0.259665750204335,
10.8899754217707));
#50199=CARTESIAN_POINT('Ctrl Pts',(2.03253759863262,-0.301311255423278,
10.8876785104643));
#50200=CARTESIAN_POINT('Ctrl Pts',(2.02213818851715,-0.371461944064481,
10.8838094276174));
#50201=CARTESIAN_POINT('Ctrl Pts',(2.00808239143017,-0.441211013602958,
10.8799403447704));
#50202=CARTESIAN_POINT('Ctrl Pts',(1.99041367942357,-0.510147966048595,
10.8760712619235));
#50203=CARTESIAN_POINT('Ctrl Pts',(1.97277129291668,-0.578982205873156,
10.8722079438171));
#50204=CARTESIAN_POINT('Ctrl Pts',(1.95152679634787,-0.647006263709907,
10.8683446257107));
#50205=CARTESIAN_POINT('Ctrl Pts',(1.92677508630939,-0.713817434136649,
10.8644813076042));
#50206=CARTESIAN_POINT('Ctrl Pts',(1.90205241001727,-0.780550235086181,
10.8606225211684));
#50207=CARTESIAN_POINT('Ctrl Pts',(1.87383085991449,-0.846072521305738,
10.8567637347326));
#50208=CARTESIAN_POINT('Ctrl Pts',(1.84225531380601,-0.90999611057054,10.8529049482969));
#50209=CARTESIAN_POINT('Ctrl Pts',(1.81069965797624,-0.973879432661422,
10.8490485926136));
#50210=CARTESIAN_POINT('Ctrl Pts',(1.77579441247878,-1.03616562127687,10.8451922369303));
#50211=CARTESIAN_POINT('Ctrl Pts',(1.73773222762227,-1.09648724004565,10.841335881247));
#50212=CARTESIAN_POINT('Ctrl Pts',(1.69968128671632,-1.15679103920421,10.8374806647698));
#50213=CARTESIAN_POINT('Ctrl Pts',(1.65847551699416,-1.21513101006899,10.8336254482926));
#50214=CARTESIAN_POINT('Ctrl Pts',(1.61435222327109,-1.27116657512683,10.8297702318154));
#50215=CARTESIAN_POINT('Ctrl Pts',(1.5702272044592,-1.32720433100768,10.8259148646108));
#50216=CARTESIAN_POINT('Ctrl Pts',(1.52318473744178,-1.38093712190746,10.8220594974061));
#50217=CARTESIAN_POINT('Ctrl Pts',(1.47350286605021,-1.43205686557546,10.8182041302015));
#50218=CARTESIAN_POINT('Ctrl Pts',(1.42376899128687,-1.48323011767541,10.8143447274787));
#50219=CARTESIAN_POINT('Ctrl Pts',(1.37139053636781,-1.53178451349683,10.8104853247559));
#50220=CARTESIAN_POINT('Ctrl Pts',(1.31668228958614,-1.57744898833218,10.8066259220331));
#50221=CARTESIAN_POINT('Ctrl Pts',(1.26194306656539,-1.62313931875188,10.8027643340862));
#50222=CARTESIAN_POINT('Ctrl Pts',(1.20487181450027,-1.66593617924574,10.7989027461393));
#50223=CARTESIAN_POINT('Ctrl Pts',(1.14581407226143,-1.70561064557761,10.7950411581924));
#50224=CARTESIAN_POINT('Ctrl Pts',(1.0866530063857,-1.74535452381041,10.7911728142589));
#50225=CARTESIAN_POINT('Ctrl Pts',(1.02549892846466,-1.78196485176482,10.7873044703255));
#50226=CARTESIAN_POINT('Ctrl Pts',(0.962723218805193,-1.81525798895732,
10.783436126392));
#50227=CARTESIAN_POINT('Ctrl Pts',(0.925448808937162,-1.83502649572909,
10.7811392150856));
#50228=CARTESIAN_POINT('Ctrl Pts',(0.887603096255043,-1.85362638322459,
10.7788423037791));
#50229=CARTESIAN_POINT('Ctrl Pts',(0.849266841179643,-1.87102736350187,
10.7765453924727));
#50230=CARTESIAN_POINT('Ctrl Pts',(0.784690491839525,-1.90033882804205,
10.7726763096258));
#50231=CARTESIAN_POINT('Ctrl Pts',(0.718468403655894,-1.92636061064501,
10.7688072267789));
#50232=CARTESIAN_POINT('Ctrl Pts',(0.650969027954004,-1.94890658758818,
10.7649381439319));
#50233=CARTESIAN_POINT('Ctrl Pts',(0.583570222955575,-1.97141897215013,
10.7610748258255));
#50234=CARTESIAN_POINT('Ctrl Pts',(0.514898365035326,-1.99046567813353,
10.7572115077191));
#50235=CARTESIAN_POINT('Ctrl Pts',(0.445343250383112,-2.00590801180867,
10.7533481896126));
#50236=CARTESIAN_POINT('Ctrl Pts',(0.375869723853611,-2.02133223163235,
10.7494894031768));
#50237=CARTESIAN_POINT('Ctrl Pts',(0.305515470492084,-2.03316037246611,
10.7456306167411));
#50238=CARTESIAN_POINT('Ctrl Pts',(0.234685193895992,-2.04130360854675,
10.7417718303053));
#50239=CARTESIAN_POINT('Ctrl Pts',(0.163899535180383,-2.04944171498578,
10.737915474622));
#50240=CARTESIAN_POINT('Ctrl Pts',(0.092638929610532,-2.05389946658242,
10.7340591189387));
#50241=CARTESIAN_POINT('Ctrl Pts',(0.0213165623719672,-2.05463942497671,
10.7302027632554));
#50242=CARTESIAN_POINT('Ctrl Pts',(-0.0499847355251396,-2.05537916477989,
10.7263475467782));
#50243=CARTESIAN_POINT('Ctrl Pts',(-0.121347273377171,-2.05240328672127,
10.722492330301));
#50244=CARTESIAN_POINT('Ctrl Pts',(-0.192356211288108,-2.04572643588503,
10.7186371138238));
#50245=CARTESIAN_POINT('Ctrl Pts',(-0.263367925436155,-2.0390493240039,
10.7147817466192));
#50246=CARTESIAN_POINT('Ctrl Pts',(-0.334025528752484,-2.02867099973832,
10.7109263794145));
#50247=CARTESIAN_POINT('Ctrl Pts',(-0.403919385645346,-2.0146579591583,
10.7070710122099));
#50248=CARTESIAN_POINT('Ctrl Pts',(-0.473886402347216,-2.00063025074597,
10.7032116094871));
#50249=CARTESIAN_POINT('Ctrl Pts',(-0.543087599495356,-1.98296032696125,
10.6993522067643));
#50250=CARTESIAN_POINT('Ctrl Pts',(-0.611124511687531,-1.96176563169882,
10.6954928040415));
#50251=CARTESIAN_POINT('Ctrl Pts',(-0.679199946913825,-1.94055893583344,
10.6916312160946));
#50252=CARTESIAN_POINT('Ctrl Pts',(-0.746109329005823,-1.91582366408486,
10.6877696281477));
#50253=CARTESIAN_POINT('Ctrl Pts',(-0.811472917657158,-1.88772595108744,
10.6839080402008));
#50254=CARTESIAN_POINT('Ctrl Pts',(-0.876950862249698,-1.85957908013401,
10.6800396962673));
#50255=CARTESIAN_POINT('Ctrl Pts',(-0.940877178113974,-1.8280582378337,
10.6761713523339));
#50256=CARTESIAN_POINT('Ctrl Pts',(-1.0028961534356,-1.7933758300825,10.6723030084004));
#50257=CARTESIAN_POINT('Ctrl Pts',(-1.0397212362307,-1.77278241443272,10.670006097094));
#50258=CARTESIAN_POINT('Ctrl Pts',(-1.07587438671979,-1.75107519229419,
10.6677091857875));
#50259=CARTESIAN_POINT('Ctrl Pts',(-1.11128635613807,-1.72830558558415,
10.6654122744811));
#50260=CARTESIAN_POINT('Ctrl Pts',(-1.17093682808642,-1.68995081998811,
10.6615431916342));
#50261=CARTESIAN_POINT('Ctrl Pts',(-1.22871614578505,-1.64842915600993,
10.6576741087873));
#50262=CARTESIAN_POINT('Ctrl Pts',(-1.28426809979031,-1.60394919195122,
10.6538050259404));
#50263=CARTESIAN_POINT('Ctrl Pts',(-1.33973728415463,-1.55953550082063,
10.6499417078339));
#50264=CARTESIAN_POINT('Ctrl Pts',(-1.39298531615975,-1.51217255996362,
10.6460783897275));
#50265=CARTESIAN_POINT('Ctrl Pts',(-1.4436842568334,-1.46211262530333,10.6422150716211));
#50266=CARTESIAN_POINT('Ctrl Pts',(-1.49432372766912,-1.41211141092715,
10.6383562851853));
#50267=CARTESIAN_POINT('Ctrl Pts',(-1.5424197024965,-1.35941982633297,10.6344974987495));
#50268=CARTESIAN_POINT('Ctrl Pts',(-1.58767805258693,-1.3043296990538,10.6306387123137));
#50269=CARTESIAN_POINT('Ctrl Pts',(-1.63290789323544,-1.24927427451525,
10.6267823566304));
#50270=CARTESIAN_POINT('Ctrl Pts',(-1.67530334787002,-1.19182367937645,
10.6229260009471));
#50271=CARTESIAN_POINT('Ctrl Pts',(-1.71460885977287,-1.13230473834935,
10.6190696452639));
#50272=CARTESIAN_POINT('Ctrl Pts',(-1.75390276043392,-1.0728033798134,10.6152144287867));
#50273=CARTESIAN_POINT('Ctrl Pts',(-1.79010826297151,-1.01123529356004,
10.6113592123095));
#50274=CARTESIAN_POINT('Ctrl Pts',(-1.82301267020963,-0.947956943513336,
10.6075039958323));
#50275=CARTESIAN_POINT('Ctrl Pts',(-1.85591836391165,-0.884676119472439,
10.6036486286276));
#50276=CARTESIAN_POINT('Ctrl Pts',(-1.88552248391556,-0.819685330896271,
10.599793261423));
#50277=CARTESIAN_POINT('Ctrl Pts',(-1.91165871748591,-0.753364792355016,
10.5959378942184));
#50278=CARTESIAN_POINT('Ctrl Pts',(-1.93782230856582,-0.686974834294604,
10.5920784914956));
#50279=CARTESIAN_POINT('Ctrl Pts',(-1.96051058858047,-0.619252800632963,
10.5882190887728));
#50280=CARTESIAN_POINT('Ctrl Pts',(-1.9796061062381,-0.550597154592022,
10.58435968605));
#50281=CARTESIAN_POINT('Ctrl Pts',(-1.99871243592782,-0.481902635184988,
10.5804980981031));
#50282=CARTESIAN_POINT('Ctrl Pts',(-2.01422184802851,-0.41227392546909,
10.5766365101562));
#50283=CARTESIAN_POINT('Ctrl Pts',(-2.02606795407287,-0.342120165992837,
10.5727749222093));
#50284=CARTESIAN_POINT('Ctrl Pts',(-2.03793478530437,-0.271843669999794,
10.5689065782758));
#50285=CARTESIAN_POINT('Ctrl Pts',(-2.04612545871765,-0.201040772966261,
10.5650382343423));
#50286=CARTESIAN_POINT('Ctrl Pts',(-2.05062549244402,-0.130125524931508,
10.5611698904089));
#50287=CARTESIAN_POINT('Ctrl Pts',(-2.05329748297105,-0.0880180914117523,
10.5588729791025));
#50288=CARTESIAN_POINT('Ctrl Pts',(-2.05466928496541,-0.0458710637282637,
10.556576067796));
#50289=CARTESIAN_POINT('Ctrl Pts',(-2.05474654051348,-0.00377051029486843,
10.5542791564896));
#50290=CARTESIAN_POINT('Ctrl Pts',(-2.05474883256118,-0.00252145467031257,
10.5542110108299));
#50291=CARTESIAN_POINT('Ctrl Pts',(-2.05474998568027,-0.00127239695515452,
10.5541428651703));
#50292=CARTESIAN_POINT('Ctrl Pts',(-2.05474999986746,-2.33384712630955E-5,
10.5540747195105));
#50293=CARTESIAN_POINT('Origin',(0.,0.,18.5459252805377));
#50294=CARTESIAN_POINT('',(1.25062491733535,1.62730785058777,11.7061482541083));
#50295=CARTESIAN_POINT('',(1.25206542099587,1.62921138715835,11.6478607732374));
#50296=CARTESIAN_POINT('',(1.25206542099588,1.62921138715835,18.5459252805377));
#50297=CARTESIAN_POINT('',(-2.05474914153225,-0.00187826315611485,11.1959252893731));
#50298=CARTESIAN_POINT('Ctrl Pts',(1.25206542099587,1.62921138715835,11.6478607732374));
#50299=CARTESIAN_POINT('Ctrl Pts',(1.30846798771459,1.58586544445223,11.644001066733));
#50300=CARTESIAN_POINT('Ctrl Pts',(1.36268721289643,1.53953314852563,11.6401413602286));
#50301=CARTESIAN_POINT('Ctrl Pts',(1.41439379402388,1.49046561782777,11.6362816537241));
#50302=CARTESIAN_POINT('Ctrl Pts',(1.46606292217753,1.44143362854267,11.6324247429467));
#50303=CARTESIAN_POINT('Ctrl Pts',(1.51522266547132,1.38967066815831,11.6285678321693));
#50304=CARTESIAN_POINT('Ctrl Pts',(1.56157735598458,1.33546760491455,11.6247109213919));
#50305=CARTESIAN_POINT('Ctrl Pts',(1.60791397665069,1.28128567094718,11.620855514104));
#50306=CARTESIAN_POINT('Ctrl Pts',(1.65144739933588,1.22466589084389,11.617000106816));
#50307=CARTESIAN_POINT('Ctrl Pts',(1.69192054918418,1.16593413954146,11.6131446995281));
#50308=CARTESIAN_POINT('Ctrl Pts',(1.73239146057176,1.10720563653375,11.6092895054723));
#50309=CARTESIAN_POINT('Ctrl Pts',(1.7698021608593,1.0463657951568,11.6054343114166));
#50310=CARTESIAN_POINT('Ctrl Pts',(1.80393844138186,0.983770126708874,11.6015791173608));
#50311=CARTESIAN_POINT('Ctrl Pts',(1.83810838664273,0.921112727259046,11.5977201213648));
#50312=CARTESIAN_POINT('Ctrl Pts',(1.86899722866235,0.856696469425504,11.5938611253687));
#50313=CARTESIAN_POINT('Ctrl Pts',(1.89643679424826,0.790901414792889,11.5900021293727));
#50314=CARTESIAN_POINT('Ctrl Pts',(1.92388957338067,0.725074676494898,11.5861412750738));
#50315=CARTESIAN_POINT('Ctrl Pts',(1.94788960352915,0.657868276882644,11.582280420775));
#50316=CARTESIAN_POINT('Ctrl Pts',(1.96831794880335,0.589679586655826,11.5784195664761));
#50317=CARTESIAN_POINT('Ctrl Pts',(1.98878387090947,0.521365467035805,11.5745516103454));
#50318=CARTESIAN_POINT('Ctrl Pts',(2.0056648664798,0.452065919930567,11.5706836542146));
#50319=CARTESIAN_POINT('Ctrl Pts',(2.01889281237227,0.382190233590036,11.5668156980839));
#50320=CARTESIAN_POINT('Ctrl Pts',(2.03047457634721,0.321010386517599,11.5634290985819));
#50321=CARTESIAN_POINT('Ctrl Pts',(2.03925671420953,0.259389223890336,11.56004249908));
#50322=CARTESIAN_POINT('Ctrl Pts',(2.04522628418895,0.197603160305332,11.556655899578));
#50323=CARTESIAN_POINT('Ctrl Pts',(2.05204632913298,0.127014536331309,11.5527868167311));
#50324=CARTESIAN_POINT('Ctrl Pts',(2.05522101457037,0.0559341627700564,
11.5489177338841));
#50325=CARTESIAN_POINT('Ctrl Pts',(2.05469356287205,-0.0152290903256963,
11.5450486510372));
#50326=CARTESIAN_POINT('Ctrl Pts',(2.05416689705046,-0.0862863137234158,
11.5411853329308));
#50327=CARTESIAN_POINT('Ctrl Pts',(2.04994904677113,-0.157425689726149,
11.5373220148244));
#50328=CARTESIAN_POINT('Ctrl Pts',(2.04203502076875,-0.228233512994843,
11.5334586967179));
#50329=CARTESIAN_POINT('Ctrl Pts',(2.03413027791583,-0.298958278714105,
11.5295999102821));
#50330=CARTESIAN_POINT('Ctrl Pts',(2.02253802503167,-0.36935178377467,11.5257411238463));
#50331=CARTESIAN_POINT('Ctrl Pts',(2.00730527915571,-0.439002367617327,
11.5218823374106));
#50332=CARTESIAN_POINT('Ctrl Pts',(1.99208212879268,-0.508609076699419,
11.5180259817273));
#50333=CARTESIAN_POINT('Ctrl Pts',(1.97322313874075,-0.577473319595851,
11.514169626044));
#50334=CARTESIAN_POINT('Ctrl Pts',(1.95082669101271,-0.64519205213052,11.5103132703607));
#50335=CARTESIAN_POINT('Ctrl Pts',(1.9284368594196,-0.712890779873512,11.5064580538835));
#50336=CARTESIAN_POINT('Ctrl Pts',(1.90251179721924,-0.779444208100835,
11.5026028374063));
#50337=CARTESIAN_POINT('Ctrl Pts',(1.87319969916412,-0.844464593426782,
11.4987476209291));
#50338=CARTESIAN_POINT('Ctrl Pts',(1.84388645509363,-0.909487520855325,
11.4948922537245));
#50339=CARTESIAN_POINT('Ctrl Pts',(1.81118611391614,-0.972976844428992,
11.4910368865198));
#50340=CARTESIAN_POINT('Ctrl Pts',(1.77529424201665,-1.03456653568657,11.4871815193152));
#50341=CARTESIAN_POINT('Ctrl Pts',(1.73936480111453,-1.0962206945562,11.4833221165924));
#50342=CARTESIAN_POINT('Ctrl Pts',(1.70023740587255,-1.15597083124951,11.4794627138696));
#50343=CARTESIAN_POINT('Ctrl Pts',(1.65815220786431,-1.21347798416564,11.4756033111468));
#50344=CARTESIAN_POINT('Ctrl Pts',(1.61604318088636,-1.2710176980835,11.4717417231999));
#50345=CARTESIAN_POINT('Ctrl Pts',(1.57097332433423,-1.32631152333354,11.467880135253));
#50346=CARTESIAN_POINT('Ctrl Pts',(1.52322279298218,-1.37905398206146,11.4640185473061));
#50347=CARTESIAN_POINT('Ctrl Pts',(1.47538872036398,-1.4318887156114,11.4601502033726));
#50348=CARTESIAN_POINT('Ctrl Pts',(1.42486495381398,-1.48216282796461,11.4562818594392));
#50349=CARTESIAN_POINT('Ctrl Pts',(1.37196764478991,-1.52960855912538,11.4524135155057));
#50350=CARTESIAN_POINT('Ctrl Pts',(1.34055874494356,-1.55778046891927,11.4501166041993));
#50351=CARTESIAN_POINT('Ctrl Pts',(1.30831365070504,-1.58495596672168,11.4478196928928));
#50352=CARTESIAN_POINT('Ctrl Pts',(1.2753034381163,-1.61108618739928,11.4455227815864));
#50353=CARTESIAN_POINT('Ctrl Pts',(1.2196986583659,-1.65510181322117,11.4416536987395));
#50354=CARTESIAN_POINT('Ctrl Pts',(1.16170357226489,-1.69632156723997,11.4377846158926));
#50355=CARTESIAN_POINT('Ctrl Pts',(1.10163089000041,-1.73447598562128,11.4339155330457));
#50356=CARTESIAN_POINT('Ctrl Pts',(1.04164771303652,-1.77257355582206,11.4300522149392));
#50357=CARTESIAN_POINT('Ctrl Pts',(0.979593491143668,-1.80761459782017,
11.4261888968328));
#50358=CARTESIAN_POINT('Ctrl Pts',(0.91581308469753,-1.83937053265425,11.4223255787264));
#50359=CARTESIAN_POINT('Ctrl Pts',(0.852107492643623,-1.87108921778899,
11.4184667922906));
#50360=CARTESIAN_POINT('Ctrl Pts',(0.786680170754984,-1.89953023450996,
11.4146080058548));
#50361=CARTESIAN_POINT('Ctrl Pts',(0.719902469801093,-1.92450980680128,
11.410749219419));
#50362=CARTESIAN_POINT('Ctrl Pts',(0.653166833902216,-1.94947364379372,
11.4068928637357));
#50363=CARTESIAN_POINT('Ctrl Pts',(0.58508296051036,-1.97098019255074,11.4030365080524));
#50364=CARTESIAN_POINT('Ctrl Pts',(0.516042820837258,-1.98889350382627,
11.3991801523692));
#50365=CARTESIAN_POINT('Ctrl Pts',(0.44702307631272,-2.00680152333027,11.395324935892));
#50366=CARTESIAN_POINT('Ctrl Pts',(0.377048096286477,-2.02111829074576,
11.3914697194148));
#50367=CARTESIAN_POINT('Ctrl Pts',(0.306524014719824,-2.03175800500454,
11.3876145029376));
#50368=CARTESIAN_POINT('Ctrl Pts',(0.23599717587256,-2.04239813524432,11.3837591357329));
#50369=CARTESIAN_POINT('Ctrl Pts',(0.164921673538474,-2.04936085661723,
11.3799037685283));
#50370=CARTESIAN_POINT('Ctrl Pts',(0.0937110916937221,-2.05261194427821,
11.3760484013237));
#50371=CARTESIAN_POINT('Ctrl Pts',(0.0224259717879226,-2.05586643494144,
11.3721889986009));
#50372=CARTESIAN_POINT('Ctrl Pts',(-0.0489940236056687,-2.0554015142251,
11.3683295958781));
#50373=CARTESIAN_POINT('Ctrl Pts',(-0.120133868146701,-2.05123509530822,
11.3644701931553));
#50374=CARTESIAN_POINT('Ctrl Pts',(-0.191313992626522,-2.04706631733221,
11.3606086052084));
#50375=CARTESIAN_POINT('Ctrl Pts',(-0.262213167440128,-2.03919192267871,
11.3567470172615));
#50376=CARTESIAN_POINT('Ctrl Pts',(-0.332422800101435,-2.027681593464,11.3528854293145));
#50377=CARTESIAN_POINT('Ctrl Pts',(-0.402755267031661,-2.01615112651577,
11.3490170853811));
#50378=CARTESIAN_POINT('Ctrl Pts',(-0.472395308450975,-2.00097212818192,
11.3451487414476));
#50379=CARTESIAN_POINT('Ctrl Pts',(-0.540946496001207,-1.98226498000747,
11.3412803975142));
#50380=CARTESIAN_POINT('Ctrl Pts',(-0.581650218436983,-1.97115721376637,
11.3389834862077));
#50381=CARTESIAN_POINT('Ctrl Pts',(-0.621970357581862,-1.95880649870203,
11.3366865749013));
#50382=CARTESIAN_POINT('Ctrl Pts',(-0.661827309974577,-1.94524604466166,
11.3343896635949));
#50383=CARTESIAN_POINT('Ctrl Pts',(-0.72896523140905,-1.92240383914107,
11.330520580748));
#50384=CARTESIAN_POINT('Ctrl Pts',(-0.795050703584486,-1.8960370323457,
11.326651497901));
#50385=CARTESIAN_POINT('Ctrl Pts',(-0.859687733168942,-1.86626219056671,
11.3227824150541));
#50386=CARTESIAN_POINT('Ctrl Pts',(-0.924228456802882,-1.83653171181704,
11.3189190969477));
#50387=CARTESIAN_POINT('Ctrl Pts',(-0.987324584002499,-1.80340347897189,
11.3150557788412));
#50388=CARTESIAN_POINT('Ctrl Pts',(-1.0485970325405,-1.7670432439098,11.3111924607348));
#50389=CARTESIAN_POINT('Ctrl Pts',(-1.10979760851999,-1.73072565938941,
11.307333674299));
#50390=CARTESIAN_POINT('Ctrl Pts',(-1.16917833922634,-1.69118384984025,
11.3034748878632));
#50391=CARTESIAN_POINT('Ctrl Pts',(-1.22638341500047,-1.64863012283283,
11.2996161014274));
#50392=CARTESIAN_POINT('Ctrl Pts',(-1.28355245577151,-1.60610320155311,
11.2957597457442));
#50393=CARTESIAN_POINT('Ctrl Pts',(-1.33854817181992,-1.56056841625879,
11.2919033900609));
#50394=CARTESIAN_POINT('Ctrl Pts',(-1.39104375021585,-1.51228133873476,
11.2880470343776));
#50395=CARTESIAN_POINT('Ctrl Pts',(-1.44352382089228,-1.46400852569694,
11.2841918179004));
#50396=CARTESIAN_POINT('Ctrl Pts',(-1.49350486283601,-1.41298536325948,
11.2803366014232));
#50397=CARTESIAN_POINT('Ctrl Pts',(-1.54069451266359,-1.35950652118639,
11.276481384946));
#50398=CARTESIAN_POINT('Ctrl Pts',(-1.58788600746534,-1.30602558825051,
11.2726260177414));
#50399=CARTESIAN_POINT('Ctrl Pts',(-1.63228557371542,-1.25008915077213,
11.2687706505367));
#50400=CARTESIAN_POINT('Ctrl Pts',(-1.67364013817998,-1.1920261114476,11.2649152833321));
#50401=CARTESIAN_POINT('Ctrl Pts',(-1.71503798959668,-1.13390229595394,
11.2610558806093));
#50402=CARTESIAN_POINT('Ctrl Pts',(-1.75338419429404,-1.07364783156664,
11.2571964778865));
#50403=CARTESIAN_POINT('Ctrl Pts',(-1.78846869960691,-1.01162111139813,
11.2533370751637));
#50404=CARTESIAN_POINT('Ctrl Pts',(-1.82357307004229,-0.949559271213391,
11.2494754872168));
#50405=CARTESIAN_POINT('Ctrl Pts',(-1.85541184776366,-0.885723612576363,
11.2456138992699));
#50406=CARTESIAN_POINT('Ctrl Pts',(-1.88382196249841,-0.820495201758459,
11.2417523113229));
#50407=CARTESIAN_POINT('Ctrl Pts',(-1.9122817817472,-0.755152671497825,
11.2378839673895));
#50408=CARTESIAN_POINT('Ctrl Pts',(-1.93730079112354,-0.688412979191603,
11.234015623456));
#50409=CARTESIAN_POINT('Ctrl Pts',(-1.95876511220552,-0.620674469997365,
11.2301472795226));
#50410=CARTESIAN_POINT('Ctrl Pts',(-1.97151000837456,-0.580453292582558,
11.2278503682161));
#50411=CARTESIAN_POINT('Ctrl Pts',(-1.98300261409516,-0.539880225197758,
11.2255534569097));
#50412=CARTESIAN_POINT('Ctrl Pts',(-1.99322765470765,-0.499040157711441,
11.2232565456033));
#50413=CARTESIAN_POINT('Ctrl Pts',(-2.01567775412989,-0.409371704526085,
11.2182134470819));
#50414=CARTESIAN_POINT('Ctrl Pts',(-2.03208632056842,-0.318134497274714,
11.2131703485606));
#50415=CARTESIAN_POINT('Ctrl Pts',(-2.0422798960547,-0.226031831100864,
11.2081272500393));
#50416=CARTESIAN_POINT('Ctrl Pts',(-2.05050113851806,-0.151749911949275,
11.2040599298172));
#50417=CARTESIAN_POINT('Ctrl Pts',(-2.05468055872562,-0.0769052702050597,
11.1999926095951));
#50418=CARTESIAN_POINT('Ctrl Pts',(-2.05474914153225,-0.00187826315611485,
11.1959252893731));
#50419=CARTESIAN_POINT('Ctrl Pts',(-2.05448230159788,-0.00187785627648217,
11.1959252805377));
#50420=CARTESIAN_POINT('Ctrl Pts',(-2.04980379711585,0.513337962037447,
11.1679913295624));
#50421=CARTESIAN_POINT('Ctrl Pts',(-1.59250349515915,1.71920574835467,11.1030130059232));
#50422=CARTESIAN_POINT('Ctrl Pts',(0.0481892737830568,2.26260148112704,
11.0203420081008));
#50423=CARTESIAN_POINT('Ctrl Pts',(0.990547142386969,1.82647893255362,10.9656049612537));
#50424=CARTESIAN_POINT('Ctrl Pts',(1.2500265821584,1.62656556227503,10.9479122870705));
#50425=CARTESIAN_POINT('',(-2.05474923773585,0.00176989376130956,11.2540747002055));
#50426=CARTESIAN_POINT('Ctrl Pts',(-2.05474923773585,0.00176989376130957,
11.2540747002055));
#50427=CARTESIAN_POINT('Ctrl Pts',(-2.05467509737831,0.0878427680056098,
11.2494166422338));
#50428=CARTESIAN_POINT('Ctrl Pts',(-2.04918878694341,0.173679370728022,
11.2447585842621));
#50429=CARTESIAN_POINT('Ctrl Pts',(-2.03840174561635,0.258681050655506,
11.2401005262904));
#50430=CARTESIAN_POINT('Ctrl Pts',(-2.02745814788226,0.344916392084481,
11.2353748641632));
#50431=CARTESIAN_POINT('Ctrl Pts',(-2.01105891234539,0.430292414196941,
11.2306492020359));
#50432=CARTESIAN_POINT('Ctrl Pts',(-1.98936916430093,0.514206077977125,
11.2259235399086));
#50433=CARTESIAN_POINT('Ctrl Pts',(-1.98195563668563,0.542887658900054,
11.2243083147521));
#50434=CARTESIAN_POINT('Ctrl Pts',(-1.9739244479774,0.571398584098788,11.2226930895955));
#50435=CARTESIAN_POINT('Ctrl Pts',(-1.96528345696356,0.599715346047911,
11.2210778644389));
#50436=CARTESIAN_POINT('Ctrl Pts',(-1.94458497416931,0.667544835634683,
11.217208781592));
#50437=CARTESIAN_POINT('Ctrl Pts',(-1.92033024378843,0.734434342938788,
11.2133396987451));
#50438=CARTESIAN_POINT('Ctrl Pts',(-1.89262319715387,0.799984372406787,
11.2094706158982));
#50439=CARTESIAN_POINT('Ctrl Pts',(-1.86495743263698,0.865436735599987,
11.2056072977917));
#50440=CARTESIAN_POINT('Ctrl Pts',(-1.83384974971676,0.929553138667919,
11.2017439796853));
#50441=CARTESIAN_POINT('Ctrl Pts',(-1.79945377757442,0.991949426570303,
11.1978806615789));
#50442=CARTESIAN_POINT('Ctrl Pts',(-1.76509815189415,1.05427252365101,11.1940218751431));
#50443=CARTESIAN_POINT('Ctrl Pts',(-1.72746213199957,1.11487909002906,11.1901630887073));
#50444=CARTESIAN_POINT('Ctrl Pts',(-1.68674661838198,1.17340675295353,11.1863043022715));
#50445=CARTESIAN_POINT('Ctrl Pts',(-1.64605675255243,1.231897547742,11.1824479465882));
#50446=CARTESIAN_POINT('Ctrl Pts',(-1.60229151840284,1.28831163937972,11.1785915909049));
#50447=CARTESIAN_POINT('Ctrl Pts',(-1.55569597970807,1.34231426321117,11.1747352352217));
#50448=CARTESIAN_POINT('Ctrl Pts',(-1.509114205802,1.39630093412681,11.1708800187445));
#50449=CARTESIAN_POINT('Ctrl Pts',(-1.45970410441845,1.44787718389519,11.1670248022673));
#50450=CARTESIAN_POINT('Ctrl Pts',(-1.40775091165561,1.49674143833622,11.1631695857901));
#50451=CARTESIAN_POINT('Ctrl Pts',(-1.35579568767834,1.54560760322345,11.1593142185854));
#50452=CARTESIAN_POINT('Ctrl Pts',(-1.30129753029019,1.5917612310577,11.1554588513808));
#50453=CARTESIAN_POINT('Ctrl Pts',(-1.24457713905028,1.63493893080244,11.1516034841762));
#50454=CARTESIAN_POINT('Ctrl Pts',(-1.18779737702768,1.6781618258248,11.1477440814534));
#50455=CARTESIAN_POINT('Ctrl Pts',(-1.12879112511406,1.71840227970392,11.1438846787306));
#50456=CARTESIAN_POINT('Ctrl Pts',(-1.06790992467806,1.75543896369942,11.1400252760078));
#50457=CARTESIAN_POINT('Ctrl Pts',(-1.00699425282815,1.79249661815632,11.1361636880609));
#50458=CARTESIAN_POINT('Ctrl Pts',(-0.944201946926682,1.82634666099208,
11.132302100114));
#50459=CARTESIAN_POINT('Ctrl Pts',(-0.879908702155135,1.85681400209382,
11.128440512167));
#50460=CARTESIAN_POINT('Ctrl Pts',(-0.815502974047321,1.88733464690089,
11.1245721682336));
#50461=CARTESIAN_POINT('Ctrl Pts',(-0.749591513662162,1.91446058926608,
11.1207038243001));
#50462=CARTESIAN_POINT('Ctrl Pts',(-0.682568848611284,1.93806535736168,
11.1168354803667));
#50463=CARTESIAN_POINT('Ctrl Pts',(-0.64277271884858,1.95208118937072,11.1145385690602));
#50464=CARTESIAN_POINT('Ctrl Pts',(-0.602585105738489,1.96485653812434,
11.1122416577538));
#50465=CARTESIAN_POINT('Ctrl Pts',(-0.562090371228137,1.97637344069197,
11.1099447464474));
#50466=CARTESIAN_POINT('Ctrl Pts',(-0.493875070548586,1.9957742092375,11.1060754904244));
#50467=CARTESIAN_POINT('Ctrl Pts',(-0.424520539258813,2.01167711519797,
11.1022062344015));
#50468=CARTESIAN_POINT('Ctrl Pts',(-0.354418830153114,2.02395277991679,
11.0983369783785));
#50469=CARTESIAN_POINT('Ctrl Pts',(-0.284439025878964,2.03620709761199,
11.0944744508791));
#50470=CARTESIAN_POINT('Ctrl Pts',(-0.21371510006283,2.04484662432041,11.0906119233798));
#50471=CARTESIAN_POINT('Ctrl Pts',(-0.142652869620053,2.04979211660333,
11.0867493958804));
#50472=CARTESIAN_POINT('Ctrl Pts',(-0.0716604748457906,2.05473274875511,
11.0828906642398));
#50473=CARTESIAN_POINT('Ctrl Pts',(-0.000330916901744124,2.05598651416958,
11.0790319325992));
#50474=CARTESIAN_POINT('Ctrl Pts',(0.0709224168760033,2.053525644662,11.0751732009586));
#50475=CARTESIAN_POINT('Ctrl Pts',(0.142129564120466,2.05106637029425,11.0713169705544));
#50476=CARTESIAN_POINT('Ctrl Pts',(0.213260100960262,2.04489725599101,11.0674607401503));
#50477=CARTESIAN_POINT('Ctrl Pts',(0.28389990271725,2.03504260587761,11.0636045097462));
#50478=CARTESIAN_POINT('Ctrl Pts',(0.35451754588503,2.02519104701218,11.0597494889806));
#50479=CARTESIAN_POINT('Ctrl Pts',(0.424644278966299,2.01165631567822,11.0558944682149));
#50480=CARTESIAN_POINT('Ctrl Pts',(0.493872093027739,1.99451445676094,11.0520394474493));
#50481=CARTESIAN_POINT('Ctrl Pts',(0.563141981578827,1.97736217956057,11.0481820837233));
#50482=CARTESIAN_POINT('Ctrl Pts',(0.631511385573021,1.95659850524197,11.0443247199972));
#50483=CARTESIAN_POINT('Ctrl Pts',(0.698584466233787,1.93235020274195,11.0404673562711));
#50484=CARTESIAN_POINT('Ctrl Pts',(0.765674913431462,1.90809562188054,11.0366089937979));
#50485=CARTESIAN_POINT('Ctrl Pts',(0.831467917351197,1.88035479749049,11.0327506313246));
#50486=CARTESIAN_POINT('Ctrl Pts',(0.895587170542185,1.84930289094573,11.0288922688514));
#50487=CARTESIAN_POINT('Ctrl Pts',(0.95980545125286,1.8182030269914,11.0250279474181));
#50488=CARTESIAN_POINT('Ctrl Pts',(1.02234438568784,1.78378209158101,11.0211636259849));
#50489=CARTESIAN_POINT('Ctrl Pts',(1.08285236991923,1.74626123688877,11.0172993045516));
#50490=CARTESIAN_POINT('Ctrl Pts',(1.14124406125458,1.71005269030342,11.0135701394304));
#50491=CARTESIAN_POINT('Ctrl Pts',(1.19774422955969,1.67095777191887,11.0098409743092));
#50492=CARTESIAN_POINT('Ctrl Pts',(1.25206542099588,1.62921138715834,11.006111809188));
#50493=CARTESIAN_POINT('Ctrl Pts',(1.25062491733525,1.62730785058785,11.7061482541084));
#50494=CARTESIAN_POINT('Ctrl Pts',(1.44978277724123,1.47638255877163,11.6926356148739));
#50495=CARTESIAN_POINT('Ctrl Pts',(2.09378666756174,0.782978067453363,11.6420786029757));
#50496=CARTESIAN_POINT('Ctrl Pts',(2.19186345478925,-1.04580741136612,11.5544772184136));
#50497=CARTESIAN_POINT('Ctrl Pts',(0.310206203218445,-2.40868234883592,
11.443344100422));
#50498=CARTESIAN_POINT('Ctrl Pts',(-1.64103540980871,-1.65033490605083,
11.343209934105));
#50499=CARTESIAN_POINT('Ctrl Pts',(-2.04952780599468,-0.479212094141424,
11.2801201404517));
#50500=CARTESIAN_POINT('Ctrl Pts',(-2.05347838646333,0.0017684434794585,
11.2540747194623));
#50501=CARTESIAN_POINT('Origin',(0.,0.,18.5459252805377));
#50502=CARTESIAN_POINT('',(1.25206542099587,1.62921138715835,12.4060251712286));
#50503=CARTESIAN_POINT('',(1.25206542099587,1.62921138715835,12.3479810351515));
#50504=CARTESIAN_POINT('',(1.25206542099588,1.62921138715835,18.5459252805377));
#50505=CARTESIAN_POINT('',(-2.0547498960994,0.000653436693597364,11.8959252805748));
#50506=CARTESIAN_POINT('Ctrl Pts',(1.25206542099587,1.62921138715835,12.3479810351515));
#50507=CARTESIAN_POINT('Ctrl Pts',(1.30851985569991,1.58582558338117,12.3441118588283));
#50508=CARTESIAN_POINT('Ctrl Pts',(1.36263268936519,1.53956655303378,12.340242682505));
#50509=CARTESIAN_POINT('Ctrl Pts',(1.41411515648718,1.49072998450197,12.3363735061818));
#50510=CARTESIAN_POINT('Ctrl Pts',(1.42203556698149,1.48321663691921,12.3357782459608));
#50511=CARTESIAN_POINT('Ctrl Pts',(1.42989379641613,1.47564234693037,12.3351829857399));
#50512=CARTESIAN_POINT('Ctrl Pts',(1.43768887830515,1.46800826009178,12.3345877255189));
#50513=CARTESIAN_POINT('Ctrl Pts',(1.48835548857877,1.41838808827663,12.330718642672));
#50514=CARTESIAN_POINT('Ctrl Pts',(1.53654944525446,1.3660446008768,12.326849559825));
#50515=CARTESIAN_POINT('Ctrl Pts',(1.58196405520874,1.31125409075721,12.3229804769781));
#50516=CARTESIAN_POINT('Ctrl Pts',(1.62731099965912,1.25654521576516,12.3191171588717));
#50517=CARTESIAN_POINT('Ctrl Pts',(1.66988650985259,1.19939692610743,12.3152538407653));
#50518=CARTESIAN_POINT('Ctrl Pts',(1.70942040407517,1.14012255684706,12.3113905226588));
#50519=CARTESIAN_POINT('Ctrl Pts',(1.74890792505505,1.080917716399,12.307531736223));
#50520=CARTESIAN_POINT('Ctrl Pts',(1.78536064871228,1.01959215223843,12.3036729497872));
#50521=CARTESIAN_POINT('Ctrl Pts',(1.81854950426628,0.956491120205974,12.2998141633515));
#50522=CARTESIAN_POINT('Ctrl Pts',(1.8517174532749,0.893429837196706,12.2959578076682));
#50523=CARTESIAN_POINT('Ctrl Pts',(1.88162538764864,0.828595734156922,12.2921014519849));
#50524=CARTESIAN_POINT('Ctrl Pts',(1.90808908639414,0.762360545203895,12.2882450963016));
#50525=CARTESIAN_POINT('Ctrl Pts',(1.93454496749805,0.696144922788906,12.2843898798244));
#50526=CARTESIAN_POINT('Ctrl Pts',(1.95755845277884,0.628529487020637,12.2805346633472));
#50527=CARTESIAN_POINT('Ctrl Pts',(1.9769932870616,0.559906336286134,12.27667944687));
#50528=CARTESIAN_POINT('Ctrl Pts',(1.99642888118825,0.491280502591688,12.2728240796654));
#50529=CARTESIAN_POINT('Ctrl Pts',(2.01228541628162,0.421647343710315,12.2689687124607));
#50530=CARTESIAN_POINT('Ctrl Pts',(2.02447686487614,0.351412842795018,12.2651133452561));
#50531=CARTESIAN_POINT('Ctrl Pts',(2.03668107459289,0.28110482550929,12.2612539425333));
#50532=CARTESIAN_POINT('Ctrl Pts',(2.04521245635311,0.210194689290596,12.2573945398105));
#50533=CARTESIAN_POINT('Ctrl Pts',(2.05003652416308,0.139096412956515,12.2535351370877));
#50534=CARTESIAN_POINT('Ctrl Pts',(2.05486332339813,0.0679578802198854,
12.2496735491408));
#50535=CARTESIAN_POINT('Ctrl Pts',(2.0559786224031,-0.00336851873967881,
12.2458119611939));
#50536=CARTESIAN_POINT('Ctrl Pts',(2.05340010221357,-0.0744686694476668,
12.241950373247));
#50537=CARTESIAN_POINT('Ctrl Pts',(2.05081707081054,-0.145693212417816,
12.2380820293135));
#50538=CARTESIAN_POINT('Ctrl Pts',(2.04452736059261,-0.216690232810768,
12.23421368538));
#50539=CARTESIAN_POINT('Ctrl Pts',(2.03460048013541,-0.287051299827666,
12.2303453414466));
#50540=CARTESIAN_POINT('Ctrl Pts',(2.0287061841907,-0.328829676606923,12.2280484301402));
#50541=CARTESIAN_POINT('Ctrl Pts',(2.02153053389919,-0.370384024467946,
12.2257515188337));
#50542=CARTESIAN_POINT('Ctrl Pts',(2.01309645181131,-0.411631191972505,
12.2234546075273));
#50543=CARTESIAN_POINT('Ctrl Pts',(1.99888947645081,-0.481110891876079,
12.2195855246804));
#50544=CARTESIAN_POINT('Ctrl Pts',(1.9810534349364,-0.549990306481095,12.2157164418335));
#50545=CARTESIAN_POINT('Ctrl Pts',(1.9596541057285,-0.617861916937283,12.2118473589865));
#50546=CARTESIAN_POINT('Ctrl Pts',(1.9382866604539,-0.685632402078804,12.2079840408801));
#50547=CARTESIAN_POINT('Ctrl Pts',(1.91336661082874,-0.752397604135835,
12.2041207227737));
#50548=CARTESIAN_POINT('Ctrl Pts',(1.88501065875936,-0.81776058774166,12.2002574046672));
#50549=CARTESIAN_POINT('Ctrl Pts',(1.85668796821084,-0.88304690059289,12.1963986182314));
#50550=CARTESIAN_POINT('Ctrl Pts',(1.82493757317916,-0.946933818635436,
12.1925398317957));
#50551=CARTESIAN_POINT('Ctrl Pts',(1.789925291033,-1.00904163195601,12.1886810453599));
#50552=CARTESIAN_POINT('Ctrl Pts',(1.75493506405724,-1.07111032190835,12.1848246896766));
#50553=CARTESIAN_POINT('Ctrl Pts',(1.71668726455152,-1.1314017084279,12.1809683339933));
#50554=CARTESIAN_POINT('Ctrl Pts',(1.6753942808025,-1.18955940009496,12.17711197831));
#50555=CARTESIAN_POINT('Ctrl Pts',(1.63411349541436,-1.24769991139755,12.1732567618328));
#50556=CARTESIAN_POINT('Ctrl Pts',(1.58978959277674,-1.30370758331733,12.1694015453556));
#50557=CARTESIAN_POINT('Ctrl Pts',(1.5426780855889,-1.3572552769261,12.1655463288784));
#50558=CARTESIAN_POINT('Ctrl Pts',(1.49556473648206,-1.41080506408953,12.1616909616738));
#50559=CARTESIAN_POINT('Ctrl Pts',(1.4456638889812,-1.46189431872944,12.1578355944691));
#50560=CARTESIAN_POINT('Ctrl Pts',(1.39326996335785,-1.51023056905388,12.1539802272645));
#50561=CARTESIAN_POINT('Ctrl Pts',(1.34082119558151,-1.55861741425176,12.1501208245417));
#50562=CARTESIAN_POINT('Ctrl Pts',(1.28587449816979,-1.60424517265427,12.1462614218189));
#50563=CARTESIAN_POINT('Ctrl Pts',(1.22875896389649,-1.64686033747371,12.1424020190961));
#50564=CARTESIAN_POINT('Ctrl Pts',(1.17161109035904,-1.68949963133423,12.1385404311492));
#50565=CARTESIAN_POINT('Ctrl Pts',(1.11229233951033,-1.72912266602566,12.1346788432023));
#50566=CARTESIAN_POINT('Ctrl Pts',(1.0511602124641,-1.76551968842956,12.1308172552554));
#50567=CARTESIAN_POINT('Ctrl Pts',(0.989921132570398,-1.80198038872877,
12.1269489113219));
#50568=CARTESIAN_POINT('Ctrl Pts',(0.926862772277252,-1.83520358177884,
12.1230805673885));
#50569=CARTESIAN_POINT('Ctrl Pts',(0.862365967892246,-1.8650261392059,12.119212223455));
#50570=CARTESIAN_POINT('Ctrl Pts',(0.824069621505006,-1.88273391558754,
12.1169153121486));
#50571=CARTESIAN_POINT('Ctrl Pts',(0.785266507841448,-1.89924367492176,
12.1146184008421));
#50572=CARTESIAN_POINT('Ctrl Pts',(0.746038917915524,-1.91452957549771,
12.1123214895357));
#50573=CARTESIAN_POINT('Ctrl Pts',(0.679961139951928,-1.94027824744361,
12.1084524066888));
#50574=CARTESIAN_POINT('Ctrl Pts',(0.612419347461162,-1.96265243793997,
12.1045833238419));
#50575=CARTESIAN_POINT('Ctrl Pts',(0.54379158745156,-1.98148637944269,12.100714240995));
#50576=CARTESIAN_POINT('Ctrl Pts',(0.475266079381733,-2.00029225931187,
12.0968509228885));
#50577=CARTESIAN_POINT('Ctrl Pts',(0.405658280198486,-2.01556823299288,
12.0929876047821));
#50578=CARTESIAN_POINT('Ctrl Pts',(0.335364965250433,-2.02719705568615,
12.0891242866757));
#50579=CARTESIAN_POINT('Ctrl Pts',(0.265154104333754,-2.03881223777487,
12.0852655002399));
#50580=CARTESIAN_POINT('Ctrl Pts',(0.194259801829534,-2.04678868774226,
12.0814067138041));
#50581=CARTESIAN_POINT('Ctrl Pts',(0.12309100067338,-2.05105976706025,12.0775479273683));
#50582=CARTESIAN_POINT('Ctrl Pts',(0.0519670306433579,-2.05532815591144,
12.073691571685));
#50583=CARTESIAN_POINT('Ctrl Pts',(-0.019430611215484,-2.0558957759222,
12.0698352160017));
#50584=CARTESIAN_POINT('Ctrl Pts',(-0.0906873134559301,-2.05274776182515,
12.0659788603185));
#50585=CARTESIAN_POINT('Ctrl Pts',(-0.161922965752997,-2.04960067768298,
12.0621236438413));
#50586=CARTESIAN_POINT('Ctrl Pts',(-0.233017276043263,-2.0427401599728,
12.0582684273641));
#50587=CARTESIAN_POINT('Ctrl Pts',(-0.303556819032513,-2.03220343964842,
12.0544132108869));
#50588=CARTESIAN_POINT('Ctrl Pts',(-0.374099119906884,-2.02166630736979,
12.0505578436822));
#50589=CARTESIAN_POINT('Ctrl Pts',(-0.444086130290927,-2.00745276106833,
12.0467024764776));
#50590=CARTESIAN_POINT('Ctrl Pts',(-0.513112447196806,-1.98965152200874,
12.042847109273));
#50591=CARTESIAN_POINT('Ctrl Pts',(-0.582211015833957,-1.97183164990601,
12.0389877065502));
#50592=CARTESIAN_POINT('Ctrl Pts',(-0.650346412265481,-1.95041671011129,
12.0351283038274));
#50593=CARTESIAN_POINT('Ctrl Pts',(-0.717127163609594,-1.9255456872568,
12.0312689011046));
#50594=CARTESIAN_POINT('Ctrl Pts',(-0.783945726739678,-1.90066058223381,
12.0274073131577));
#50595=CARTESIAN_POINT('Ctrl Pts',(-0.849407671902037,-1.87231569176008,
12.0235457252108));
#50596=CARTESIAN_POINT('Ctrl Pts',(-0.913142876995169,-1.84069759838301,
12.0196841372638));
#50597=CARTESIAN_POINT('Ctrl Pts',(-0.97698958911414,-1.80902418801826,
12.0158157933304));
#50598=CARTESIAN_POINT('Ctrl Pts',(-1.03910310618935,-1.7740663797939,12.0119474493969));
#50599=CARTESIAN_POINT('Ctrl Pts',(-1.09913982055953,-1.73605564926945,
12.0080791054635));
#50600=CARTESIAN_POINT('Ctrl Pts',(-1.13478789384623,-1.71348597133768,
12.005782194157));
#50601=CARTESIAN_POINT('Ctrl Pts',(-1.16970433398133,-1.68984076058459,
12.0034852828506));
#50602=CARTESIAN_POINT('Ctrl Pts',(-1.20382279746224,-1.66517513637761,
12.0011883715442));
#50603=CARTESIAN_POINT('Ctrl Pts',(-1.26083681927375,-1.62395738232141,
11.9973500934401));
#50604=CARTESIAN_POINT('Ctrl Pts',(-1.31585191288247,-1.5797208791892,11.993511815336));
#50605=CARTESIAN_POINT('Ctrl Pts',(-1.36852678994371,-1.53268783113404,
11.9896735372319));
#50606=CARTESIAN_POINT('Ctrl Pts',(-1.42213348718528,-1.48482276702558,
11.9857673598712));
#50607=CARTESIAN_POINT('Ctrl Pts',(-1.4733158971113,-1.43406148037154,11.9818611825105));
#50608=CARTESIAN_POINT('Ctrl Pts',(-1.5217450967034,-1.38068440389509,11.9779550051498));
#50609=CARTESIAN_POINT('Ctrl Pts',(-1.5692056384388,-1.32837495035961,11.974126957294));
#50610=CARTESIAN_POINT('Ctrl Pts',(-1.6140217352881,-1.27355376028476,11.9702989094383));
#50611=CARTESIAN_POINT('Ctrl Pts',(-1.6559188631244,-1.21652385149195,11.9664708615825));
#50612=CARTESIAN_POINT('Ctrl Pts',(-1.69779086095982,-1.15952814937945,
11.9626451097993));
#50613=CARTESIAN_POINT('Ctrl Pts',(-1.73674706992695,-1.10032675344736,
11.9588193580162));
#50614=CARTESIAN_POINT('Ctrl Pts',(-1.77255338645319,-1.03925552905593,
11.954993606233));
#50615=CARTESIAN_POINT('Ctrl Pts',(-1.80835068587627,-0.978199684228333,
11.9511688178887));
#50616=CARTESIAN_POINT('Ctrl Pts',(-1.84099941769869,-0.915275372082998,
11.9473440295444));
#50617=CARTESIAN_POINT('Ctrl Pts',(-1.87030994639299,-0.850845618736703,
11.9435192412002));
#50618=CARTESIAN_POINT('Ctrl Pts',(-1.90070387548185,-0.784034358699591,
11.9395530778147));
#50619=CARTESIAN_POINT('Ctrl Pts',(-1.92750771800191,-0.715604685579293,
11.9355869144293));
#50620=CARTESIAN_POINT('Ctrl Pts',(-1.95056426599362,-0.64598498955375,
11.9316207510438));
#50621=CARTESIAN_POINT('Ctrl Pts',(-1.97282450374,-0.578769767833822,11.9277915681179));
#50622=CARTESIAN_POINT('Ctrl Pts',(-1.99159199666899,-0.510445894525309,
11.9239623851919));
#50623=CARTESIAN_POINT('Ctrl Pts',(-2.00677657951126,-0.441412870706191,
11.920133202266));
#50624=CARTESIAN_POINT('Ctrl Pts',(-2.02197110779225,-0.37233463236159,
11.916301511342));
#50625=CARTESIAN_POINT('Ctrl Pts',(-2.03357797952057,-0.302546806993616,
11.912469820418));
#50626=CARTESIAN_POINT('Ctrl Pts',(-2.0415586573881,-0.232456040884489,
11.908638129494));
#50627=CARTESIAN_POINT('Ctrl Pts',(-2.04955171545767,-0.162256544933185,
11.9048004945752));
#50628=CARTESIAN_POINT('Ctrl Pts',(-2.05390733765599,-0.091753662965547,
11.9009628596564));
#50629=CARTESIAN_POINT('Ctrl Pts',(-2.0546390270676,-0.0213548811910643,
11.8971252247376));
#50630=CARTESIAN_POINT('Ctrl Pts',(-2.05471528813786,-0.0140174968341446,
11.89672524335));
#50631=CARTESIAN_POINT('Ctrl Pts',(-2.05475222861971,-0.0066812384315459,
11.8963252619624));
#50632=CARTESIAN_POINT('Ctrl Pts',(-2.0547498960994,0.000653436693603956,
11.8959252805748));
#50633=CARTESIAN_POINT('Ctrl Pts',(-2.05474989609918,0.000653437373812688,
11.8959252805377));
#50634=CARTESIAN_POINT('Ctrl Pts',(-2.05473848559207,0.0365340576922297,
11.893968604876));
#50635=CARTESIAN_POINT('Ctrl Pts',(-2.05378729851884,0.0723985335872527,
11.8920119292143));
#50636=CARTESIAN_POINT('Ctrl Pts',(-2.05189850659895,0.108213128210028,
11.8900552535526));
#50637=CARTESIAN_POINT('Ctrl Pts',(-2.04816365541142,0.179032036237403,
11.8861861707057));
#50638=CARTESIAN_POINT('Ctrl Pts',(-2.04075083573292,0.249796068327482,
11.8823170878588));
#50639=CARTESIAN_POINT('Ctrl Pts',(-2.02966459840712,0.320092456132394,
11.8784480050119));
#50640=CARTESIAN_POINT('Ctrl Pts',(-2.01859487902203,0.390284105825381,
11.8745846869055));
#50641=CARTESIAN_POINT('Ctrl Pts',(-2.00386268121796,0.460009018352436,
11.870721368799));
#50642=CARTESIAN_POINT('Ctrl Pts',(-1.9855244861849,0.528857331669124,11.8668580506926));
#50643=CARTESIAN_POINT('Ctrl Pts',(-1.96720780184756,0.597624885940748,
11.8629992642568));
#50644=CARTESIAN_POINT('Ctrl Pts',(-1.94529364658789,0.665517416317043,
11.859140477821));
#50645=CARTESIAN_POINT('Ctrl Pts',(-1.91988963003493,0.732134803833518,
11.8552816913852));
#50646=CARTESIAN_POINT('Ctrl Pts',(-1.89450161614958,0.798710227280726,
11.8514253357019));
#50647=CARTESIAN_POINT('Ctrl Pts',(-1.86562827515809,0.864011648670079,
11.8475689800187));
#50648=CARTESIAN_POINT('Ctrl Pts',(-1.83342673333031,0.927655095393628,
11.8437126243354));
#50649=CARTESIAN_POINT('Ctrl Pts',(-1.80123470416043,0.991279741205714,
11.8398574078582));
#50650=CARTESIAN_POINT('Ctrl Pts',(-1.7657166452435,1.05324695148401,11.836002191381));
#50651=CARTESIAN_POINT('Ctrl Pts',(-1.72707667211473,1.11319527987551,11.8321469749038));
#50652=CARTESIAN_POINT('Ctrl Pts',(-1.68843518827859,1.17314595206732,11.8282916076992));
#50653=CARTESIAN_POINT('Ctrl Pts',(-1.64667181293418,1.2310771785415,11.8244362404945));
#50654=CARTESIAN_POINT('Ctrl Pts',(-1.60203428460654,1.28665601986125,11.8205808732899));
#50655=CARTESIAN_POINT('Ctrl Pts',(-1.55735003295878,1.34229303707229,11.8167214705671));
#50656=CARTESIAN_POINT('Ctrl Pts',(-1.50978592759242,1.39557237428656,11.8128620678443));
#50657=CARTESIAN_POINT('Ctrl Pts',(-1.45962977992668,1.44619447794935,11.8090026651215));
#50658=CARTESIAN_POINT('Ctrl Pts',(-1.40944523345615,1.49684524424488,11.8051410771746));
#50659=CARTESIAN_POINT('Ctrl Pts',(-1.35666608266766,1.54483545493889,11.8012794892277));
#50660=CARTESIAN_POINT('Ctrl Pts',(-1.30161472803287,1.58990460791455,11.7974179012807));
#50661=CARTESIAN_POINT('Ctrl Pts',(-1.24646705907993,1.63505261098876,11.7935495573473));
#50662=CARTESIAN_POINT('Ctrl Pts',(-1.1890396410044,1.67726906527471,11.7896812134138));
#50663=CARTESIAN_POINT('Ctrl Pts',(-1.1296848726291,1.71633611249457,11.7858128694804));
#50664=CARTESIAN_POINT('Ctrl Pts',(-1.0944417192495,1.7395330008819,11.783515958174));
#50665=CARTESIAN_POINT('Ctrl Pts',(-1.05851956096535,1.76162038025266,11.7812190468675));
#50666=CARTESIAN_POINT('Ctrl Pts',(-1.02199594055809,1.78256047863257,11.7789221355611));
#50667=CARTESIAN_POINT('Ctrl Pts',(-0.960472923613762,1.81783348862112,
11.7750530527142));
#50668=CARTESIAN_POINT('Ctrl Pts',(-0.897001152031734,1.84998675199316,
11.7711839698673));
#50669=CARTESIAN_POINT('Ctrl Pts',(-0.831929874442541,1.87880021463433,
11.7673148870203));
#50670=CARTESIAN_POINT('Ctrl Pts',(-0.766955549811701,1.90757074665316,
11.7634515689139));
#50671=CARTESIAN_POINT('Ctrl Pts',(-0.700386890294981,1.9330111603523,11.7595882508075));
#50672=CARTESIAN_POINT('Ctrl Pts',(-0.632598868839114,1.95494660634082,
11.755724932701));
#50673=CARTESIAN_POINT('Ctrl Pts',(-0.564890362706312,1.97685632205963,
11.7518661462652));
#50674=CARTESIAN_POINT('Ctrl Pts',(-0.495965795661029,1.99526908771997,
11.7480073598295));
#50675=CARTESIAN_POINT('Ctrl Pts',(-0.426219686225407,2.01005829307857,
11.7441485733937));
#50676=CARTESIAN_POINT('Ctrl Pts',(-0.356517511724471,2.02483818232223,
11.7402922177104));
#50677=CARTESIAN_POINT('Ctrl Pts',(-0.285995295661607,2.03599893933331,
11.7364358620271));
#50678=CARTESIAN_POINT('Ctrl Pts',(-0.215060848322245,2.04346431190244,
11.7325795063438));
#50679=CARTESIAN_POINT('Ctrl Pts',(-0.144147355728934,2.05092747912576,
11.7287242898666));
#50680=CARTESIAN_POINT('Ctrl Pts',(-0.0728223564725586,2.0546973783256,
11.7248690733894));
#50681=CARTESIAN_POINT('Ctrl Pts',(-0.00150022183944837,2.05474945232611,
11.7210138569122));
#50682=CARTESIAN_POINT('Ctrl Pts',(0.0698247012758174,2.05480152836255,
11.7171584897076));
#50683=CARTESIAN_POINT('Ctrl Pts',(0.141146273760915,2.05113549246291,11.7133031225029));
#50684=CARTESIAN_POINT('Ctrl Pts',(0.212050413681591,2.04377889815838,11.7094477552983));
#50685=CARTESIAN_POINT('Ctrl Pts',(0.283028770902149,2.03641460350565,11.7055883525755));
#50686=CARTESIAN_POINT('Ctrl Pts',(0.353588339152754,2.0253520892534,11.7017289498527));
#50687=CARTESIAN_POINT('Ctrl Pts',(0.423321350333843,2.01067068334214,11.69786954713));
#50688=CARTESIAN_POINT('Ctrl Pts',(0.493093844893627,1.99598096470352,11.694007959183));
#50689=CARTESIAN_POINT('Ctrl Pts',(0.562038381008229,1.97766840015477,11.6901463712361));
#50690=CARTESIAN_POINT('Ctrl Pts',(0.629761238561418,1.95586255777485,11.6862847832892));
#50691=CARTESIAN_POINT('Ctrl Pts',(0.69760257968133,1.93401856529209,11.6824164393557));
#50692=CARTESIAN_POINT('Ctrl Pts',(0.764217520754356,1.90866926579212,11.6785480954223));
#50693=CARTESIAN_POINT('Ctrl Pts',(0.829231897648688,1.87999255914005,11.6746797514888));
#50694=CARTESIAN_POINT('Ctrl Pts',(0.867835563697562,1.86296515597387,11.6723828401824));
#50695=CARTESIAN_POINT('Ctrl Pts',(0.905875373419138,1.84476552247177,11.6700859288759));
#50696=CARTESIAN_POINT('Ctrl Pts',(0.943277535649769,1.8254383181139,11.6677890175695));
#50697=CARTESIAN_POINT('Ctrl Pts',(1.00626540384789,1.79288994849758,11.6639208576022));
#50698=CARTESIAN_POINT('Ctrl Pts',(1.06768998270875,1.75701386646393,11.6600526976348));
#50699=CARTESIAN_POINT('Ctrl Pts',(1.12717723733065,1.71798400404184,11.6561845376675));
#50700=CARTESIAN_POINT('Ctrl Pts',(1.16984678376852,1.68998831761005,11.6534099495242));
#50701=CARTESIAN_POINT('Ctrl Pts',(1.21151987881709,1.66037104620426,11.6506353613808));
#50702=CARTESIAN_POINT('Ctrl Pts',(1.25206542099587,1.62921138715835,11.6478607732374));
#50703=CARTESIAN_POINT('',(-2.05466569125301,-0.00102264302692682,11.9540747659024));
#50704=CARTESIAN_POINT('Ctrl Pts',(-2.05188276458647,-0.00102039859364231,
11.9540747194623));
#50705=CARTESIAN_POINT('Ctrl Pts',(-2.05004756599998,0.40727097526418,11.9320086704376));
#50706=CARTESIAN_POINT('Ctrl Pts',(-1.7342531973136,1.50361561120492,11.8728982487491));
#50707=CARTESIAN_POINT('Ctrl Pts',(-0.200040598667229,2.29813379067046,
11.7902560936311));
#50708=CARTESIAN_POINT('Ctrl Pts',(0.90379928332058,1.89013835121545,11.7296799875378));
#50709=CARTESIAN_POINT('Ctrl Pts',(1.25062491733525,1.62730785058785,11.7061482541084));
#50710=CARTESIAN_POINT('Ctrl Pts',(1.25206542099587,1.62921138715835,12.4060251712286));
#50711=CARTESIAN_POINT('Ctrl Pts',(1.30857348607413,1.58578436789642,12.402169202365));
#50712=CARTESIAN_POINT('Ctrl Pts',(1.36285495219622,1.5393867813656,12.3983132335015));
#50713=CARTESIAN_POINT('Ctrl Pts',(1.41458832701998,1.49028098946434,12.394457264638));
#50714=CARTESIAN_POINT('Ctrl Pts',(1.46631052222186,1.44118580936228,12.3906021290523));
#50715=CARTESIAN_POINT('Ctrl Pts',(1.51548536748826,1.3893839205327,12.3867469934665));
#50716=CARTESIAN_POINT('Ctrl Pts',(1.56182668300009,1.33517600891004,12.3828918578808));
#50717=CARTESIAN_POINT('Ctrl Pts',(1.60817348550792,1.28096167885511,12.3790362658318));
#50718=CARTESIAN_POINT('Ctrl Pts',(1.65168577852569,1.2243411313406,12.3751806737827));
#50719=CARTESIAN_POINT('Ctrl Pts',(1.69211742153164,1.16564840078349,12.3713250817336));
#50720=CARTESIAN_POINT('Ctrl Pts',(1.73259335532627,1.10689137535402,12.3674652660814));
#50721=CARTESIAN_POINT('Ctrl Pts',(1.76998162974679,1.0460580384509,12.3636054504292));
#50722=CARTESIAN_POINT('Ctrl Pts',(1.80407977935618,0.983510911082403,12.359745634777));
#50723=CARTESIAN_POINT('Ctrl Pts',(1.83819966057492,0.920923920854698,12.3558833591671));
#50724=CARTESIAN_POINT('Ctrl Pts',(1.86902503473518,0.856621404660003,12.3520210835572));
#50725=CARTESIAN_POINT('Ctrl Pts',(1.89640089579593,0.790987487211018,12.3481588079473));
#50726=CARTESIAN_POINT('Ctrl Pts',(1.92382270088975,0.72524341845512,12.3442900504037));
#50727=CARTESIAN_POINT('Ctrl Pts',(1.94778327885194,0.658163946893732,12.34042129286));
#50728=CARTESIAN_POINT('Ctrl Pts',(1.96817720266579,0.590149185720579,12.3365525353163));
#50729=CARTESIAN_POINT('Ctrl Pts',(1.97545792419331,0.565867613406076,12.3351713716624));
#50730=CARTESIAN_POINT('Ctrl Pts',(1.9822845424209,0.541466932141748,12.3337902080085));
#50731=CARTESIAN_POINT('Ctrl Pts',(1.98865384835457,0.516965602264348,12.3324090443545));
#50732=CARTESIAN_POINT('Ctrl Pts',(2.00649631927715,0.448329510599995,12.3285399615076));
#50733=CARTESIAN_POINT('Ctrl Pts',(2.0208162221759,0.378634184255975,12.3246708786607));
#50734=CARTESIAN_POINT('Ctrl Pts',(2.03149314948497,0.308274465526457,12.3208017958138));
#50735=CARTESIAN_POINT('Ctrl Pts',(2.04215416870484,0.23801957926887,12.3169384777073));
#50736=CARTESIAN_POINT('Ctrl Pts',(2.04918291418265,0.16710274194488,12.3130751596009));
#50737=CARTESIAN_POINT('Ctrl Pts',(2.05250935872637,0.0959317196794512,
12.3092118414945));
#50738=CARTESIAN_POINT('Ctrl Pts',(2.05583190135193,0.0248441809956648,
12.3053530550587));
#50739=CARTESIAN_POINT('Ctrl Pts',(2.05546074673972,-0.0464964674867899,
12.3014942686229));
#50740=CARTESIAN_POINT('Ctrl Pts',(2.05137754985214,-0.11767629524525,12.2976354821871));
#50741=CARTESIAN_POINT('Ctrl Pts',(2.04729692507919,-0.188811284931504,
12.2937791265038));
#50742=CARTESIAN_POINT('Ctrl Pts',(2.03950892496536,-0.259785171042465,
12.2899227708206));
#50743=CARTESIAN_POINT('Ctrl Pts',(2.02804728537728,-0.330184449624538,
12.2860664151373));
#50744=CARTESIAN_POINT('Ctrl Pts',(2.01658903167228,-0.400562931554911,
12.2822111986601));
#50745=CARTESIAN_POINT('Ctrl Pts',(2.00145937099513,-0.470366663738085,
12.2783559821829));
#50746=CARTESIAN_POINT('Ctrl Pts',(1.98274363903717,-0.53918941417433,12.2745007657057));
#50747=CARTESIAN_POINT('Ctrl Pts',(1.96402717535011,-0.608014855374075,
12.2706453985011));
#50748=CARTESIAN_POINT('Ctrl Pts',(1.94172449162492,-0.675858770499862,
12.2667900312964));
#50749=CARTESIAN_POINT('Ctrl Pts',(1.9159711219694,-0.742328917852,12.2629346640918));
#50750=CARTESIAN_POINT('Ctrl Pts',(1.89019079555839,-0.808868641323056,
12.259075261369));
#50751=CARTESIAN_POINT('Ctrl Pts',(1.86095274886154,-0.874031272628489,
12.2552158586462));
#50752=CARTESIAN_POINT('Ctrl Pts',(1.82844080481938,-0.937444284089179,
12.2513564559235));
#50753=CARTESIAN_POINT('Ctrl Pts',(1.79591045225908,-1.00089320049512,12.2474948679765));
#50754=CARTESIAN_POINT('Ctrl Pts',(1.76010275615705,-1.06259010463368,12.2436332800296));
#50755=CARTESIAN_POINT('Ctrl Pts',(1.72124631310105,-1.12218924078608,12.2397716920827));
#50756=CARTESIAN_POINT('Ctrl Pts',(1.6823218893052,-1.18189264776338,12.2359033481492));
#50757=CARTESIAN_POINT('Ctrl Pts',(1.64033835552297,-1.23949056656658,12.2320350042158));
#50758=CARTESIAN_POINT('Ctrl Pts',(1.59556579163784,-1.29466882524262,12.2281666602823));
#50759=CARTESIAN_POINT('Ctrl Pts',(1.56898113164501,-1.32743208735248,12.2258697489759));
#50760=CARTESIAN_POINT('Ctrl Pts',(1.54141390511254,-1.3593429288423,12.2235728376694));
#50761=CARTESIAN_POINT('Ctrl Pts',(1.5129266135236,-1.39034190924103,12.221275926363));
#50762=CARTESIAN_POINT('Ctrl Pts',(1.46494056768335,-1.4425588246249,12.2174068435161));
#50763=CARTESIAN_POINT('Ctrl Pts',(1.41415405217899,-1.49239082213816,12.2135377606691));
#50764=CARTESIAN_POINT('Ctrl Pts',(1.3608334803882,-1.53952258871201,12.2096686778222));
#50765=CARTESIAN_POINT('Ctrl Pts',(1.30759235359024,-1.58658413130417,12.2058053597158));
#50766=CARTESIAN_POINT('Ctrl Pts',(1.25182502601033,-1.63095310980967,12.2019420416094));
#50767=CARTESIAN_POINT('Ctrl Pts',(1.19383609408718,-1.67234952774672,12.1980787235029));
#50768=CARTESIAN_POINT('Ctrl Pts',(1.13591518315877,-1.71369738770151,12.1942199370671));
#50769=CARTESIAN_POINT('Ctrl Pts',(1.0757782376257,-1.75207933220145,12.1903611506314));
#50770=CARTESIAN_POINT('Ctrl Pts',(1.01376306422456,-1.7872554412042,12.1865023641956));
#50771=CARTESIAN_POINT('Ctrl Pts',(0.951786955835391,-1.82240939183757,
12.1826460085123));
#50772=CARTESIAN_POINT('Ctrl Pts',(0.887935388464297,-1.85436127440682,
12.178789652829));
#50773=CARTESIAN_POINT('Ctrl Pts',(0.822574058130612,-1.88291515512265,
12.1749332971457));
#50774=CARTESIAN_POINT('Ctrl Pts',(0.757232036188336,-1.91146060073621,
12.1710780806685));
#50775=CARTESIAN_POINT('Ctrl Pts',(0.690381581630985,-1.93660984295883,
12.1672228641913));
#50776=CARTESIAN_POINT('Ctrl Pts',(0.622410267798343,-1.95821424288539,
12.1633676477141));
#50777=CARTESIAN_POINT('Ctrl Pts',(0.55443629649076,-1.97981948747932,12.1595122805095));
#50778=CARTESIAN_POINT('Ctrl Pts',(0.485341842531987,-1.99787946956899,
12.1556569133049));
#50779=CARTESIAN_POINT('Ctrl Pts',(0.415529952181181,-2.01229531166285,
12.1518015461003));
#50780=CARTESIAN_POINT('Ctrl Pts',(0.345644987817769,-2.02672624321242,
12.1479421433775));
#50781=CARTESIAN_POINT('Ctrl Pts',(0.275041564697992,-2.03750532188664,
12.1440827406547));
#50782=CARTESIAN_POINT('Ctrl Pts',(0.204132357592777,-2.04458493173642,
12.1402233379319));
#50783=CARTESIAN_POINT('Ctrl Pts',(0.133183001137418,-2.05166855011691,
12.136361749985));
#50784=CARTESIAN_POINT('Ctrl Pts',(0.061928001500897,-2.05504850680639,
12.132500162038));
#50785=CARTESIAN_POINT('Ctrl Pts',(-0.00921817421015008,-2.05472932226224,
12.1286385740911));
#50786=CARTESIAN_POINT('Ctrl Pts',(-0.0804888227056832,-2.05440957929328,
12.1247702301576));
#50787=CARTESIAN_POINT('Ctrl Pts',(-0.151649781995328,-2.05037780148638,
12.1209018862242));
#50788=CARTESIAN_POINT('Ctrl Pts',(-0.222290619815562,-2.04269049120076,
12.1170335422907));
#50789=CARTESIAN_POINT('Ctrl Pts',(-0.264235116446928,-2.03812598757469,
12.1147366309843));
#50790=CARTESIAN_POINT('Ctrl Pts',(-0.305996391073655,-2.03227366112877,
12.1124397196778));
#50791=CARTESIAN_POINT('Ctrl Pts',(-0.347490606215405,-2.02515378208472,
12.1101428083714));
#50792=CARTESIAN_POINT('Ctrl Pts',(-0.41738645095297,-2.013160544991,12.1062737255245));
#50793=CARTESIAN_POINT('Ctrl Pts',(-0.486797566932928,-1.99752100818105,
12.1024046426776));
#50794=CARTESIAN_POINT('Ctrl Pts',(-0.555314551843232,-1.97828797474259,
12.0985355598307));
#50795=CARTESIAN_POINT('Ctrl Pts',(-0.623729449863567,-1.95908359756464,
12.0946722417242));
#50796=CARTESIAN_POINT('Ctrl Pts',(-0.691252397319804,-1.93629648177733,
12.0908089236178));
#50797=CARTESIAN_POINT('Ctrl Pts',(-0.757482952791989,-1.91003066434273,
12.0869456055113));
#50798=CARTESIAN_POINT('Ctrl Pts',(-0.823635819847797,-1.88379565670198,
12.0830868190755));
#50799=CARTESIAN_POINT('Ctrl Pts',(-0.888498856782718,-1.85409023091444,
12.0792280326397));
#50800=CARTESIAN_POINT('Ctrl Pts',(-0.951687279107213,-1.821068061684,12.0753692462039));
#50801=CARTESIAN_POINT('Ctrl Pts',(-1.01483589735908,-1.78806669399875,
12.0715128905207));
#50802=CARTESIAN_POINT('Ctrl Pts',(-1.0763115643563,-1.75175295248498,12.0676565348374));
#50803=CARTESIAN_POINT('Ctrl Pts',(-1.13575132331738,-1.71232779983355,
12.0638001791541));
#50804=CARTESIAN_POINT('Ctrl Pts',(-1.19517352317843,-1.67291429376703,
12.0599449626769));
#50805=CARTESIAN_POINT('Ctrl Pts',(-1.25256060439685,-1.63039146968246,
12.0560897461997));
#50806=CARTESIAN_POINT('Ctrl Pts',(-1.30757747835969,-1.58500432194569,
12.0522345297225));
#50807=CARTESIAN_POINT('Ctrl Pts',(-1.36259650331782,-1.53961539970714,
12.0483791625179));
#50808=CARTESIAN_POINT('Ctrl Pts',(-1.41524476371604,-1.49136224231808,
12.0445237953132));
#50809=CARTESIAN_POINT('Ctrl Pts',(-1.46522058494397,-1.44052983306714,
12.0406684281086));
#50810=CARTESIAN_POINT('Ctrl Pts',(-1.51524871722895,-1.38964421614508,
12.0368090253858));
#50811=CARTESIAN_POINT('Ctrl Pts',(-1.56259848500875,-1.336174305125,12.032949622663));
#50812=CARTESIAN_POINT('Ctrl Pts',(-1.60700605787508,-1.28044097577858,
12.0290902199402));
#50813=CARTESIAN_POINT('Ctrl Pts',(-1.65143877465797,-1.22467608978332,
12.0252286319933));
#50814=CARTESIAN_POINT('Ctrl Pts',(-1.69292569759206,-1.16664562962774,
12.0213670440464));
#50815=CARTESIAN_POINT('Ctrl Pts',(-1.73124582566109,-1.10670025464488,
12.0175054560994));
#50816=CARTESIAN_POINT('Ctrl Pts',(-1.76963299616775,-1.04665000307977,
12.013637112166));
#50817=CARTESIAN_POINT('Ctrl Pts',(-1.80484207015481,-0.984678570400846,
12.0097687682325));
#50818=CARTESIAN_POINT('Ctrl Pts',(-1.83669790674073,-0.921161420096516,
12.0059004242991));
#50819=CARTESIAN_POINT('Ctrl Pts',(-1.85561298577411,-0.88344676411059,
12.0036035129927));
#50820=CARTESIAN_POINT('Ctrl Pts',(-1.87334674624879,-0.845187549237961,
12.0013066016863));
#50821=CARTESIAN_POINT('Ctrl Pts',(-1.88987074604909,-0.806465204288353,
11.9990096903798));
#50822=CARTESIAN_POINT('Ctrl Pts',(-1.92069469607791,-0.734232352669482,
11.9947250207971));
#50823=CARTESIAN_POINT('Ctrl Pts',(-1.94740950840208,-0.660146193744584,
11.9904403512143));
#50824=CARTESIAN_POINT('Ctrl Pts',(-1.96981308826176,-0.584665682089075,
11.9861556816316));
#50825=CARTESIAN_POINT('Ctrl Pts',(-1.99214571435029,-0.509424222718199,
11.9818845819099));
#50826=CARTESIAN_POINT('Ctrl Pts',(-2.01019421233967,-0.432797493083545,
11.9776134821881));
#50827=CARTESIAN_POINT('Ctrl Pts',(-2.02380481117486,-0.355262788320802,
11.9733423824664));
#50828=CARTESIAN_POINT('Ctrl Pts',(-2.03734384291512,-0.278135775654815,
11.9690937409923));
#50829=CARTESIAN_POINT('Ctrl Pts',(-2.04649139620821,-0.200110594467843,
11.9648450995182));
#50830=CARTESIAN_POINT('Ctrl Pts',(-2.05114422938467,-0.121675440257956,
11.9605964580442));
#50831=CARTESIAN_POINT('Ctrl Pts',(-2.05352493854566,-0.08154262588682,
11.9584225611311));
#50832=CARTESIAN_POINT('Ctrl Pts',(-2.05472969689495,-0.0413027495048298,
11.9562486642181));
#50833=CARTESIAN_POINT('Ctrl Pts',(-2.05474974548303,-0.00102271081675177,
11.9540747673051));
#50834=CARTESIAN_POINT('Origin',(0.,0.,18.5459252805377));
#50835=CARTESIAN_POINT('',(1.25206542099588,1.62921138715834,13.1060515834985));
#50836=CARTESIAN_POINT('',(1.2502432481766,1.62681756561327,13.047972482772));
#50837=CARTESIAN_POINT('',(1.25206542099588,1.62921138715835,18.5459252805377));
#50838=CARTESIAN_POINT('',(-2.0547494773391,0.00146556292173476,12.5959252537175));
#50839=CARTESIAN_POINT('Ctrl Pts',(1.25024324817659,1.62681756561327,13.047972482772));
#50840=CARTESIAN_POINT('Ctrl Pts',(1.47885177013841,1.452673658258,13.0324437996707));
#50841=CARTESIAN_POINT('Ctrl Pts',(2.13338525759955,0.709856746996147,12.9798707439056));
#50842=CARTESIAN_POINT('Ctrl Pts',(2.1316126390019,-1.16370384027608,12.8902533154766));
#50843=CARTESIAN_POINT('Ctrl Pts',(0.178478656788241,-2.42200834839547,
12.7791201974851));
#50844=CARTESIAN_POINT('Ctrl Pts',(-1.68997359897976,-1.57591260505555,
12.6810108525054));
#50845=CARTESIAN_POINT('Ctrl Pts',(-2.04962979387723,-0.442629241759327,
12.6199458801896));
#50846=CARTESIAN_POINT('Ctrl Pts',(-2.05255322210627,0.00146350058043466,
12.5959252805377));
#50847=CARTESIAN_POINT('Ctrl Pts',(-2.0547494773391,0.00146556292173476,
12.5959252537175));
#50848=CARTESIAN_POINT('Ctrl Pts',(-2.05469114092328,0.0832544224373133,
12.5915060692206));
#50849=CARTESIAN_POINT('Ctrl Pts',(-2.04974540773188,0.164848037177314,
12.5870868847237));
#50850=CARTESIAN_POINT('Ctrl Pts',(-2.04000589565819,0.245710211793937,
12.5826677002268));
#50851=CARTESIAN_POINT('Ctrl Pts',(-2.03017754638782,0.327309956101516,
12.5782082069382));
#50852=CARTESIAN_POINT('Ctrl Pts',(-2.01546767759796,0.408164668537392,
12.5737487136497));
#50853=CARTESIAN_POINT('Ctrl Pts',(-1.99602219393391,0.487742722983417,
12.5692892203612));
#50854=CARTESIAN_POINT('Ctrl Pts',(-1.97794767235628,0.561710297513277,
12.5651441340748));
#50855=CARTESIAN_POINT('Ctrl Pts',(-1.95578233527752,0.634574984482566,
12.5609990477884));
#50856=CARTESIAN_POINT('Ctrl Pts',(-1.92968005290243,0.705926664697185,
12.556853961502));
#50857=CARTESIAN_POINT('Ctrl Pts',(-1.90531580906655,0.772527343897062,
12.5529848786551));
#50858=CARTESIAN_POINT('Ctrl Pts',(-1.87745182895922,0.837995631989894,
12.5491157958081));
#50859=CARTESIAN_POINT('Ctrl Pts',(-1.84621366087208,0.901938291076125,
12.5452467129612));
#50860=CARTESIAN_POINT('Ctrl Pts',(-1.81502203609748,0.965785678789267,
12.5413833948548));
#50861=CARTESIAN_POINT('Ctrl Pts',(-1.78046641403582,1.0281115166333,12.5375200767484));
#50862=CARTESIAN_POINT('Ctrl Pts',(-1.74272113095632,1.08854059282064,12.5336567586419));
#50863=CARTESIAN_POINT('Ctrl Pts',(-1.70502012307931,1.14889878572493,12.5297979722061));
#50864=CARTESIAN_POINT('Ctrl Pts',(-1.6641371421163,1.20736422636482,12.5259391857703));
#50865=CARTESIAN_POINT('Ctrl Pts',(-1.62029253832278,1.26358602902831,12.5220803993346));
#50866=CARTESIAN_POINT('Ctrl Pts',(-1.57647555341467,1.31977241607866,12.5182240436513));
#50867=CARTESIAN_POINT('Ctrl Pts',(-1.52970094503791,1.37371758700872,12.514367687968));
#50868=CARTESIAN_POINT('Ctrl Pts',(-1.48023165653616,1.42510062995152,12.5105113322847));
#50869=CARTESIAN_POINT('Ctrl Pts',(-1.43077698175754,1.47646849382896,12.5066561158075));
#50870=CARTESIAN_POINT('Ctrl Pts',(-1.37862954394352,1.5252753825675,12.5028008993303));
#50871=CARTESIAN_POINT('Ctrl Pts',(-1.32409059027219,1.57123571473304,12.4989456828531));
#50872=CARTESIAN_POINT('Ctrl Pts',(-1.26954950429088,1.61719784381012,12.4950903156485));
#50873=CARTESIAN_POINT('Ctrl Pts',(-1.21261708970847,1.66031288400247,12.4912349484438));
#50874=CARTESIAN_POINT('Ctrl Pts',(-1.1536279235862,1.70033531293748,12.4873795812392));
#50875=CARTESIAN_POINT('Ctrl Pts',(-1.09457701189259,1.74039963444197,12.4835201785164));
#50876=CARTESIAN_POINT('Ctrl Pts',(-1.03346545388818,1.77736460937187,12.4796607757936));
#50877=CARTESIAN_POINT('Ctrl Pts',(-0.970656330330856,1.81102839593658,
12.4758013730708));
#50878=CARTESIAN_POINT('Ctrl Pts',(-0.907811643754378,1.8447112432017,12.4719397851239));
#50879=CARTESIAN_POINT('Ctrl Pts',(-0.84326791796477,1.87508897421654,12.468078197177));
#50880=CARTESIAN_POINT('Ctrl Pts',(-0.777409831760266,1.90200723342012,
12.4642166092301));
#50881=CARTESIAN_POINT('Ctrl Pts',(-0.711436524473381,1.92897258708302,
12.4603482652966));
#50882=CARTESIAN_POINT('Ctrl Pts',(-0.644144724493293,1.95246622483331,
12.4564799213632));
#50883=CARTESIAN_POINT('Ctrl Pts',(-0.575935265499068,1.97238336346019,
12.4526115774297));
#50884=CARTESIAN_POINT('Ctrl Pts',(-0.535434451645713,1.98420958721146,
12.4503146661233));
#50885=CARTESIAN_POINT('Ctrl Pts',(-0.494610339145961,1.9947758363981,12.4480177548168));
#50886=CARTESIAN_POINT('Ctrl Pts',(-0.453548143508707,2.00406877227799,
12.4457208435104));
#50887=CARTESIAN_POINT('Ctrl Pts',(-0.380743650195929,2.02054542379707,
12.4416483514955));
#50888=CARTESIAN_POINT('Ctrl Pts',(-0.306889998070348,2.03308359131829,
12.4375758594805));
#50889=CARTESIAN_POINT('Ctrl Pts',(-0.23245234744894,2.04155907792684,12.4335033674655));
#50890=CARTESIAN_POINT('Ctrl Pts',(-0.16185603027104,2.04959718949886,12.4296410352238));
#50891=CARTESIAN_POINT('Ctrl Pts',(-0.0907350550844751,2.05398142394467,
12.4257787029821));
#50892=CARTESIAN_POINT('Ctrl Pts',(-0.0194993857400896,2.05465747424133,
12.4219163707404));
#50893=CARTESIAN_POINT('Ctrl Pts',(0.0516664469702679,2.05533286176501,
12.4180578249765));
#50894=CARTESIAN_POINT('Ctrl Pts',(0.122946267557767,2.05230727293557,12.4141992792127));
#50895=CARTESIAN_POINT('Ctrl Pts',(0.193925736297766,2.04557824863811,12.4103407334488));
#50896=CARTESIAN_POINT('Ctrl Pts',(0.264859365375091,2.0388535700509,12.4064846795948));
#50897=CARTESIAN_POINT('Ctrl Pts',(0.335492545182316,2.02843024911777,12.4026286257407));
#50898=CARTESIAN_POINT('Ctrl Pts',(0.405413417056765,2.01435784402135,12.3987725718867));
#50899=CARTESIAN_POINT('Ctrl Pts',(0.475312522755492,2.00028981962607,12.3949177184117));
#50900=CARTESIAN_POINT('Ctrl Pts',(0.544499285330755,1.98257506415181,12.3910628649366));
#50901=CARTESIAN_POINT('Ctrl Pts',(0.612571145518115,1.96131439452695,12.3872080114616));
#50902=CARTESIAN_POINT('Ctrl Pts',(0.680674715449567,1.94004382109762,12.3833513622898));
#50903=CARTESIAN_POINT('Ctrl Pts',(0.747661880423524,1.91522417591916,12.379494713118));
#50904=CARTESIAN_POINT('Ctrl Pts',(0.813145524332736,1.88700607279299,12.3756380639462));
#50905=CARTESIAN_POINT('Ctrl Pts',(0.878646757697546,1.85878039004782,12.3717803788462));
#50906=CARTESIAN_POINT('Ctrl Pts',(0.942643226698747,1.82715464010088,12.3679226937461));
#50907=CARTESIAN_POINT('Ctrl Pts',(1.00477027017304,1.79232649555721,12.364065008646));
#50908=CARTESIAN_POINT('Ctrl Pts',(1.06696943851605,1.75745791813258,12.360202845061));
#50909=CARTESIAN_POINT('Ctrl Pts',(1.12729443571184,1.71937978027434,12.3563406814759));
#50910=CARTESIAN_POINT('Ctrl Pts',(1.18540845321352,1.67833380516211,12.3524785178908));
#50911=CARTESIAN_POINT('Ctrl Pts',(1.20796634379055,1.66240114975445,12.3509793569777));
#50912=CARTESIAN_POINT('Ctrl Pts',(1.23019144193433,1.64602176119478,12.3494801960646));
#50913=CARTESIAN_POINT('Ctrl Pts',(1.25206542099587,1.62921138715835,12.3479810351515));
#50914=CARTESIAN_POINT('',(-2.05474964003203,-0.00121625993429837,12.6540747194125));
#50915=CARTESIAN_POINT('Ctrl Pts',(-2.05474964003203,-0.00121625993429152,
12.6540747194125));
#50916=CARTESIAN_POINT('Ctrl Pts',(-2.05479111887721,0.0688581047612897,
12.6502578388075));
#50917=CARTESIAN_POINT('Ctrl Pts',(-2.05124368555208,0.139075573134476,
12.6464409582024));
#50918=CARTESIAN_POINT('Ctrl Pts',(-2.044089796226,0.209032216332157,12.6426240775974));
#50919=CARTESIAN_POINT('Ctrl Pts',(-2.0369463642195,0.278886599215084,12.6388127763825));
#50920=CARTESIAN_POINT('Ctrl Pts',(-2.02620699185267,0.348480420599989,
12.6350014751677));
#50921=CARTESIAN_POINT('Ctrl Pts',(-2.01190615332121,0.41741010137304,12.6311901739529));
#50922=CARTESIAN_POINT('Ctrl Pts',(-1.99761679316685,0.486284456658215,
12.6273819318281));
#50923=CARTESIAN_POINT('Ctrl Pts',(-1.9797717334666,0.554495240735824,12.6235736897033));
#50924=CARTESIAN_POINT('Ctrl Pts',(-1.95845703300675,0.62164588984919,12.6197654475785));
#50925=CARTESIAN_POINT('Ctrl Pts',(-1.93715187206696,0.688766485292987,
12.615958909855));
#50926=CARTESIAN_POINT('Ctrl Pts',(-1.91238030076588,0.754827411188127,
12.6121523721315));
#50927=CARTESIAN_POINT('Ctrl Pts',(-1.88427857892226,0.819446032094063,
12.6083458344079));
#50928=CARTESIAN_POINT('Ctrl Pts',(-1.85617945689729,0.884058674836218,
12.6045396488446));
#50929=CARTESIAN_POINT('Ctrl Pts',(-1.82475099666655,0.947228820103455,
12.6007334632813));
#50930=CARTESIAN_POINT('Ctrl Pts',(-1.79017732801765,1.00859441637934,12.5969272777179));
#50931=CARTESIAN_POINT('Ctrl Pts',(-1.75557129150574,1.07001746311657,12.5931175288043));
#50932=CARTESIAN_POINT('Ctrl Pts',(-1.71781441294439,1.12963215146144,12.5893077798906));
#50933=CARTESIAN_POINT('Ctrl Pts',(-1.67713593618041,1.18710261311828,12.585498030977));
#50934=CARTESIAN_POINT('Ctrl Pts',(-1.63643771004458,1.24460097664382,12.5816864324329));
#50935=CARTESIAN_POINT('Ctrl Pts',(-1.59281537301402,1.2999526496942,12.5778748338888));
#50936=CARTESIAN_POINT('Ctrl Pts',(-1.54653873298482,1.35285457824472,12.5740632353447));
#50937=CARTESIAN_POINT('Ctrl Pts',(-1.50018078791144,1.40584945204009,12.5702449400701));
#50938=CARTESIAN_POINT('Ctrl Pts',(-1.45115957837219,1.45638563068069,12.5664266447955));
#50939=CARTESIAN_POINT('Ctrl Pts',(-1.39978145601897,1.50419727359326,12.5626083495209));
#50940=CARTESIAN_POINT('Ctrl Pts',(-1.3641995911793,1.53730917683064,12.5599639931265));
#50941=CARTESIAN_POINT('Ctrl Pts',(-1.32748803416161,1.56911514178964,12.5573196367321));
#50942=CARTESIAN_POINT('Ctrl Pts',(-1.28975687735514,1.59953892100665,12.5546752803376));
#50943=CARTESIAN_POINT('Ctrl Pts',(-1.23455063817286,1.64405339059733,12.5508061974907));
#50944=CARTESIAN_POINT('Ctrl Pts',(-1.17692901738585,1.68579362240212,12.5469371146438));
#50945=CARTESIAN_POINT('Ctrl Pts',(-1.11720228643712,1.72448734807759,12.5430680317969));
#50946=CARTESIAN_POINT('Ctrl Pts',(-1.05756454533888,1.7631234220315,12.5392047136905));
#50947=CARTESIAN_POINT('Ctrl Pts',(-0.995828324344066,1.79872173795106,
12.535341395584));
#50948=CARTESIAN_POINT('Ctrl Pts',(-0.932336411880873,1.8310506212503,12.5314780774776));
#50949=CARTESIAN_POINT('Ctrl Pts',(-0.868918975406488,1.8633415827819,12.5276192910418));
#50950=CARTESIAN_POINT('Ctrl Pts',(-0.803750368975177,1.89237051003465,
12.523760504606));
#50951=CARTESIAN_POINT('Ctrl Pts',(-0.737200273710599,1.91795029105058,
12.5199017181702));
#50952=CARTESIAN_POINT('Ctrl Pts',(-0.670692100126142,1.94351395868015,
12.5160453624869));
#50953=CARTESIAN_POINT('Ctrl Pts',(-0.602804616613449,1.96563261681741,
12.5121890068037));
#50954=CARTESIAN_POINT('Ctrl Pts',(-0.533928554502491,1.98416679268324,
12.5083326511204));
#50955=CARTESIAN_POINT('Ctrl Pts',(-0.465072839069948,2.00269549336793,
12.5044774346432));
#50956=CARTESIAN_POINT('Ctrl Pts',(-0.395229593652036,2.01764168781327,
12.500622218166));
#50957=CARTESIAN_POINT('Ctrl Pts',(-0.324804163254478,2.02891592187369,
12.4967670016888));
#50958=CARTESIAN_POINT('Ctrl Pts',(-0.254375979433294,2.04019059672293,
12.4929116344842));
#50959=CARTESIAN_POINT('Ctrl Pts',(-0.18336604546572,2.04779295154757,12.4890562672795));
#50960=CARTESIAN_POINT('Ctrl Pts',(-0.112187620427746,2.05168503925987,
12.4852009000749));
#50961=CARTESIAN_POINT('Ctrl Pts',(-0.0409346909881128,2.05558120092668,
12.4813414973521));
#50962=CARTESIAN_POINT('Ctrl Pts',(0.0304865955321654,2.05575931629186,
12.4774820946293));
#50963=CARTESIAN_POINT('Ctrl Pts',(0.101661068335935,2.05223356119249,12.4736226919065));
#50964=CARTESIAN_POINT('Ctrl Pts',(0.172875840685214,2.04870580978289,12.4697611039596));
#50965=CARTESIAN_POINT('Ctrl Pts',(0.243843037616678,2.04147006240673,12.4658995160127));
#50966=CARTESIAN_POINT('Ctrl Pts',(0.314153455834246,2.03059231966621,12.4620379280658));
#50967=CARTESIAN_POINT('Ctrl Pts',(0.384586884648705,2.01969554592486,12.4581695841323));
#50968=CARTESIAN_POINT('Ctrl Pts',(0.454360764920788,2.00514415454549,12.4543012401989));
#50969=CARTESIAN_POINT('Ctrl Pts',(0.523077600526005,1.98705495302167,12.4504328962654));
#50970=CARTESIAN_POINT('Ctrl Pts',(0.563879680009971,1.97631410571874,12.448135984959));
#50971=CARTESIAN_POINT('Ctrl Pts',(0.604309382418821,1.96432690644618,12.4458390736525));
#50972=CARTESIAN_POINT('Ctrl Pts',(0.644286808518715,1.95112584700956,12.4435421623461));
#50973=CARTESIAN_POINT('Ctrl Pts',(0.711614188174318,1.92889348171609,12.4396738537867));
#50974=CARTESIAN_POINT('Ctrl Pts',(0.777921303223199,1.90312859844738,12.4358055452274));
#50975=CARTESIAN_POINT('Ctrl Pts',(0.842811364020459,1.87394412061245,12.431937236668));
#50976=CARTESIAN_POINT('Ctrl Pts',(0.907616620856139,1.84479778358532,12.4280739835499));
#50977=CARTESIAN_POINT('Ctrl Pts',(0.971008056576276,1.8122409112598,12.4242107304318));
#50978=CARTESIAN_POINT('Ctrl Pts',(1.0326051273996,1.77643581740744,12.4203474773137));
#50979=CARTESIAN_POINT('Ctrl Pts',(1.09413108355865,1.74067206102771,12.4164886843744));
#50980=CARTESIAN_POINT('Ctrl Pts',(1.15386637137547,1.7016677742289,12.412629891435));
#50981=CARTESIAN_POINT('Ctrl Pts',(1.21145327695171,1.65963204363587,12.4087710984957));
#50982=CARTESIAN_POINT('Ctrl Pts',(1.22511294175184,1.64966113125946,12.4078557894067));
#50983=CARTESIAN_POINT('Ctrl Pts',(1.23865184132203,1.63951985873777,12.4069404803176));
#50984=CARTESIAN_POINT('Ctrl Pts',(1.25206542099587,1.62921138715835,12.4060251712286));
#50985=CARTESIAN_POINT('Ctrl Pts',(1.25206542099588,1.62921138715834,13.1060515834985));
#50986=CARTESIAN_POINT('Ctrl Pts',(1.30834031581923,1.58596356159447,13.1021847974854));
#50987=CARTESIAN_POINT('Ctrl Pts',(1.36247333019475,1.53971860876087,13.0983180114722));
#50988=CARTESIAN_POINT('Ctrl Pts',(1.41412862706877,1.49071720611409,13.0944512254591));
#50989=CARTESIAN_POINT('Ctrl Pts',(1.46714239897573,1.44042712280717,13.090482747411));
#50990=CARTESIAN_POINT('Ctrl Pts',(1.51754582996521,1.38723380459452,13.0865142693628));
#50991=CARTESIAN_POINT('Ctrl Pts',(1.56500993085928,1.33144338175223,13.0825457913147));
#50992=CARTESIAN_POINT('Ctrl Pts',(1.61114869445704,1.27721079160406,13.0786881248456));
#50993=CARTESIAN_POINT('Ctrl Pts',(1.65450979289494,1.22052463414179,13.0748304583765));
#50994=CARTESIAN_POINT('Ctrl Pts',(1.69482808368481,1.16170363228031,13.0709727919073));
#50995=CARTESIAN_POINT('Ctrl Pts',(1.73512633244712,1.10291187005467,13.0671170430656));
#50996=CARTESIAN_POINT('Ctrl Pts',(1.77238450077215,1.04198776935196,13.0632612942238));
#50997=CARTESIAN_POINT('Ctrl Pts',(1.80637926427822,0.979281122091948,13.0594055453821));
#50998=CARTESIAN_POINT('Ctrl Pts',(1.84036850083389,0.916584669829447,13.0555504234173));
#50999=CARTESIAN_POINT('Ctrl Pts',(1.87109515527224,0.852106673817415,13.0516953014524));
#51000=CARTESIAN_POINT('Ctrl Pts',(1.89838145671275,0.786222237862287,13.0478401794876));
#51001=CARTESIAN_POINT('Ctrl Pts',(1.92706621861358,0.716961133990656,13.0437874772223));
#51002=CARTESIAN_POINT('Ctrl Pts',(1.95194827002454,0.646146091395115,13.039734774957));
#51003=CARTESIAN_POINT('Ctrl Pts',(1.97287896198443,0.574235286149538,13.0356820726917));
#51004=CARTESIAN_POINT('Ctrl Pts',(1.99281564784182,0.505739550954497,13.0318218347171));
#51005=CARTESIAN_POINT('Ctrl Pts',(2.00916769123172,0.436250271976713,13.0279615967426));
#51006=CARTESIAN_POINT('Ctrl Pts',(2.02185882763527,0.366175427375082,13.024101358768));
#51007=CARTESIAN_POINT('Ctrl Pts',(2.0345588558355,0.296051486203185,13.0202384161932));
#51008=CARTESIAN_POINT('Ctrl Pts',(2.04359281349571,0.225341644505659,13.0163754736184));
#51009=CARTESIAN_POINT('Ctrl Pts',(2.04893629360516,0.154459144266526,13.0125125310435));
#51010=CARTESIAN_POINT('Ctrl Pts',(2.05428842000437,0.0834619489927554,
13.008643337838));
#51011=CARTESIAN_POINT('Ctrl Pts',(2.05593815011108,0.0122920220530018,
13.0047741446325));
#51012=CARTESIAN_POINT('Ctrl Pts',(2.05391312248099,-0.0586382793097567,
13.0009049514269));
#51013=CARTESIAN_POINT('Ctrl Pts',(2.05361703361221,-0.0690093341934075,
13.0003392183859));
#51014=CARTESIAN_POINT('Ctrl Pts',(2.05324247306339,-0.0793752786927251,
12.9997734853449));
#51015=CARTESIAN_POINT('Ctrl Pts',(2.05278961933086,-0.0897348386495988,
12.9992077523039));
#51016=CARTESIAN_POINT('Ctrl Pts',(2.04969252497423,-0.16058450240405,12.995338669457));
#51017=CARTESIAN_POINT('Ctrl Pts',(2.04291711713161,-0.231412406381142,
12.9914695866101));
#51018=CARTESIAN_POINT('Ctrl Pts',(2.03246423017578,-0.301805757990093,
12.9876005037631));
#51019=CARTESIAN_POINT('Ctrl Pts',(2.0220269175002,-0.37209422701583,12.9837371856567));
#51020=CARTESIAN_POINT('Ctrl Pts',(2.00792307266343,-0.441948952266497,
12.9798738675503));
#51021=CARTESIAN_POINT('Ctrl Pts',(1.99020548444614,-0.510959579791311,
12.9760105494438));
#51022=CARTESIAN_POINT('Ctrl Pts',(1.972508678953,-0.579889257876603,12.9721517630081));
#51023=CARTESIAN_POINT('Ctrl Pts',(1.9512066702235,-0.647976336722143,12.9682929765723));
#51024=CARTESIAN_POINT('Ctrl Pts',(1.92640346112517,-0.71481974473638,12.9644341901365));
#51025=CARTESIAN_POINT('Ctrl Pts',(1.90161587622982,-0.781621046304986,
12.9605778344532));
#51026=CARTESIAN_POINT('Ctrl Pts',(1.87333163524002,-0.847179776975268,
12.9567214787699));
#51027=CARTESIAN_POINT('Ctrl Pts',(1.84170440102805,-0.911110565043517,
12.9528651230867));
#51028=CARTESIAN_POINT('Ctrl Pts',(1.81008650981775,-0.975022467316813,
12.9490099066095));
#51029=CARTESIAN_POINT('Ctrl Pts',(1.77512780124049,-1.03730694655122,12.9451546901323));
#51030=CARTESIAN_POINT('Ctrl Pts',(1.73702912834051,-1.09760073332547,12.9412994736551));
#51031=CARTESIAN_POINT('Ctrl Pts',(1.69892896589637,-1.15789687740644,12.9374441064504));
#51032=CARTESIAN_POINT('Ctrl Pts',(1.65768885675581,-1.21620176501485,12.9335887392458));
#51033=CARTESIAN_POINT('Ctrl Pts',(1.61355353184179,-1.27218023973842,12.9297333720412));
#51034=CARTESIAN_POINT('Ctrl Pts',(1.5693720092777,-1.32821730866042,12.9258739693184));
#51035=CARTESIAN_POINT('Ctrl Pts',(1.52228952276467,-1.38192272139538,12.9220145665956));
#51036=CARTESIAN_POINT('Ctrl Pts',(1.47259117507951,-1.43299434527075,12.9181551638728));
#51037=CARTESIAN_POINT('Ctrl Pts',(1.42286468779949,-1.48409488630074,12.9142935759259));
#51038=CARTESIAN_POINT('Ctrl Pts',(1.37051974752311,-1.53255833962242,12.910431987979));
#51039=CARTESIAN_POINT('Ctrl Pts',(1.31587639627039,-1.57812131100193,12.9065704000321));
#51040=CARTESIAN_POINT('Ctrl Pts',(1.26113744451604,-1.623763996433,12.9027020560986));
#51041=CARTESIAN_POINT('Ctrl Pts',(1.20409244236039,-1.66649577720976,12.8988337121652));
#51042=CARTESIAN_POINT('Ctrl Pts',(1.14509181289497,-1.70609563112415,12.8949653682317));
#51043=CARTESIAN_POINT('Ctrl Pts',(1.1100589370082,-1.72960888479427,12.8926684569253));
#51044=CARTESIAN_POINT('Ctrl Pts',(1.07433709447014,-1.752018787717,12.8903715456188));
#51045=CARTESIAN_POINT('Ctrl Pts',(1.03800348484611,-1.77328687130632,12.8880746343123));
#51046=CARTESIAN_POINT('Ctrl Pts',(0.976800535752212,-1.80911236320516,
12.8842055514654));
#51047=CARTESIAN_POINT('Ctrl Pts',(0.913620822920747,-1.84183578019922,
12.8803364686185));
#51048=CARTESIAN_POINT('Ctrl Pts',(0.848811599608828,-1.87123393269508,
12.8764673857716));
#51049=CARTESIAN_POINT('Ctrl Pts',(0.784098938807428,-1.90058828340989,
12.8726040676651));
#51050=CARTESIAN_POINT('Ctrl Pts',(0.717762025611132,-1.92662700508797,
12.8687407495587));
#51051=CARTESIAN_POINT('Ctrl Pts',(0.650174243543331,-1.94917187942286,
12.8648774314523));
#51052=CARTESIAN_POINT('Ctrl Pts',(0.582665741917904,-1.97169030862884,
12.8610186450165));
#51053=CARTESIAN_POINT('Ctrl Pts',(0.513909744499352,-1.9907228780986,12.8571598585807));
#51054=CARTESIAN_POINT('Ctrl Pts',(0.444299613906862,-2.00613943074309,
12.8533010721449));
#51055=CARTESIAN_POINT('Ctrl Pts',(0.374733332592358,-2.02154627208987,
12.8494447164616));
#51056=CARTESIAN_POINT('Ctrl Pts',(0.304314458738831,-2.03334151098861,
12.8455883607783));
#51057=CARTESIAN_POINT('Ctrl Pts',(0.23345009957965,-2.04144522667307,12.8417320050951));
#51058=CARTESIAN_POINT('Ctrl Pts',(0.162606674461754,-2.04954654843877,
12.8378767886179));
#51059=CARTESIAN_POINT('Ctrl Pts',(0.0913185076770635,-2.05395845679896,
12.8340215721407));
#51060=CARTESIAN_POINT('Ctrl Pts',(0.0199997326209688,-2.05465266485484,
12.8301663556635));
#51061=CARTESIAN_POINT('Ctrl Pts',(-0.0513218307859419,-2.05534690005218,
12.8263109884588));
#51062=CARTESIAN_POINT('Ctrl Pts',(-0.122673519058635,-2.05232314384442,
12.8224556212542));
#51063=CARTESIAN_POINT('Ctrl Pts',(-0.193641018972577,-2.04560522053285,
12.8186002540496));
#51064=CARTESIAN_POINT('Ctrl Pts',(-0.264682802507017,-2.03888026538747,
12.8147408513268));
#51065=CARTESIAN_POINT('Ctrl Pts',(-0.335339110308355,-2.02845347004202,
12.810881448604));
#51066=CARTESIAN_POINT('Ctrl Pts',(-0.40520147658915,-2.01440048795416,
12.8070220458812));
#51067=CARTESIAN_POINT('Ctrl Pts',(-0.475103399490517,-2.00033954895746,
12.8031604579343));
#51068=CARTESIAN_POINT('Ctrl Pts',(-0.544210015153872,-1.98264845651046,
12.7992988699874));
#51069=CARTESIAN_POINT('Ctrl Pts',(-0.612126452877568,-1.96145322865153,
12.7954372820404));
#51070=CARTESIAN_POINT('Ctrl Pts',(-0.680161712843429,-1.94022091898176,
12.791568938107));
#51071=CARTESIAN_POINT('Ctrl Pts',(-0.747002181878165,-1.91547240269251,
12.7877005941735));
#51072=CARTESIAN_POINT('Ctrl Pts',(-0.812272109325285,-1.88738220371822,
12.7838322502401));
#51073=CARTESIAN_POINT('Ctrl Pts',(-0.851027513938246,-1.8707030519329,
12.7815353389336));
#51074=CARTESIAN_POINT('Ctrl Pts',(-0.889229639044953,-1.85284664074278,
12.7792384276272));
#51075=CARTESIAN_POINT('Ctrl Pts',(-0.926804294388877,-1.83385696345226,
12.7769415163208));
#51076=CARTESIAN_POINT('Ctrl Pts',(-0.990097750284713,-1.80186938323196,
12.7730724334739));
#51077=CARTESIAN_POINT('Ctrl Pts',(-1.05185720819241,-1.76653855402879,
12.7692033506269));
#51078=CARTESIAN_POINT('Ctrl Pts',(-1.11170681581917,-1.72803516114725,
12.76533426778));
#51079=CARTESIAN_POINT('Ctrl Pts',(-1.17146725051544,-1.68958913640083,
12.7614709496736));
#51080=CARTESIAN_POINT('Ctrl Pts',(-1.22932307811853,-1.64798019155231,
12.7576076315671));
#51081=CARTESIAN_POINT('Ctrl Pts',(-1.28492205565918,-1.60342535634827,
12.7537443134607));
#51082=CARTESIAN_POINT('Ctrl Pts',(-1.34045581562056,-1.55892278394878,
12.7498855270249));
#51083=CARTESIAN_POINT('Ctrl Pts',(-1.39373760668099,-1.51148148734931,
12.7460267405891));
#51084=CARTESIAN_POINT('Ctrl Pts',(-1.44444472742131,-1.46136134885414,
12.7421679541533));
#51085=CARTESIAN_POINT('Ctrl Pts',(-1.49511990639376,-1.41127278237106,
12.7383115984701));
#51086=CARTESIAN_POINT('Ctrl Pts',(-1.54322328810036,-1.35850906260196,
12.7344552427868));
#51087=CARTESIAN_POINT('Ctrl Pts',(-1.58846692151022,-1.30336886634899,
12.7305988871035));
#51088=CARTESIAN_POINT('Ctrl Pts',(-1.63369718949773,-1.24824495906213,
12.7267436706263));
#51089=CARTESIAN_POINT('Ctrl Pts',(-1.67606907837354,-1.19074634436575,
12.7228884541491));
#51090=CARTESIAN_POINT('Ctrl Pts',(-1.71533420557472,-1.13120560716669,
12.7190332376719));
#51091=CARTESIAN_POINT('Ctrl Pts',(-1.7546008679249,-1.07166254210292,12.7151778704672));
#51092=CARTESIAN_POINT('Ctrl Pts',(-1.79076026184735,-1.01007760277419,
12.7113225032626));
#51093=CARTESIAN_POINT('Ctrl Pts',(-1.82360768758627,-0.94681178925712,
12.707467136058));
#51094=CARTESIAN_POINT('Ctrl Pts',(-1.85648949562289,-0.883479753685019,
12.7036077333352));
#51095=CARTESIAN_POINT('Ctrl Pts',(-1.88605219080747,-0.818463763753936,
12.6997483306124));
#51096=CARTESIAN_POINT('Ctrl Pts',(-1.91213778830766,-0.752148018029615,
12.6958889278896));
#51097=CARTESIAN_POINT('Ctrl Pts',(-1.93823815567809,-0.685794723809099,
12.6920273399427));
#51098=CARTESIAN_POINT('Ctrl Pts',(-1.96085735206333,-0.618140669715462,
12.6881657519957));
#51099=CARTESIAN_POINT('Ctrl Pts',(-1.97988707928822,-0.549585949390586,
12.6843041640488));
#51100=CARTESIAN_POINT('Ctrl Pts',(-1.99895009970299,-0.480911290125275,
12.6804358201154));
#51101=CARTESIAN_POINT('Ctrl Pts',(-2.01441100754087,-0.411333292970025,
12.6765674761819));
#51102=CARTESIAN_POINT('Ctrl Pts',(-2.02621262637065,-0.341262296827762,
12.6726991322485));
#51103=CARTESIAN_POINT('Ctrl Pts',(-2.03322008801068,-0.299656155786641,
12.670402220942));
#51104=CARTESIAN_POINT('Ctrl Pts',(-2.03893840716793,-0.257876320827019,
12.6681053096356));
#51105=CARTESIAN_POINT('Ctrl Pts',(-2.04336430473757,-0.216008982739983,
12.6658083983292));
#51106=CARTESIAN_POINT('Ctrl Pts',(-2.05090081120964,-0.144716446142108,
12.6618971720403));
#51107=CARTESIAN_POINT('Ctrl Pts',(-2.05470713587996,-0.0730227242236319,
12.6579859457513));
#51108=CARTESIAN_POINT('Ctrl Pts',(-2.05474964003149,-0.00121626084838144,
12.6540747194623));
#51109=CARTESIAN_POINT('Origin',(0.,0.,18.5459252805377));
#51110=CARTESIAN_POINT('',(1.25171901745462,1.62874802847325,13.8061758215987));
#51111=CARTESIAN_POINT('',(1.25206542099588,1.62921138715834,13.7478651251903));
#51112=CARTESIAN_POINT('',(1.25206542099588,1.62921138715835,18.5459252805377));
#51113=CARTESIAN_POINT('',(-2.05474946769684,-0.00147901978776689,13.2959253072757));
#51114=CARTESIAN_POINT('Ctrl Pts',(1.25206542099588,1.62921138715834,13.7478651251903));
#51115=CARTESIAN_POINT('Ctrl Pts',(1.30854407481545,1.58580697074604,13.7440082043291));
#51116=CARTESIAN_POINT('Ctrl Pts',(1.36281046402495,1.53942583980054,13.740151283468));
#51117=CARTESIAN_POINT('Ctrl Pts',(1.41454030475051,1.49032657117034,13.7362943626069));
#51118=CARTESIAN_POINT('Ctrl Pts',(1.46624989922677,1.44124651922472,13.7324389512841));
#51119=CARTESIAN_POINT('Ctrl Pts',(1.51542456358849,1.38945077514556,13.7285835399614));
#51120=CARTESIAN_POINT('Ctrl Pts',(1.56177476026823,1.3352367433115,13.7247281286387));
#51121=CARTESIAN_POINT('Ctrl Pts',(1.60812232080023,1.28102579487747,13.7208729365908));
#51122=CARTESIAN_POINT('Ctrl Pts',(1.65164541814656,1.22439720203785,13.717017744543));
#51123=CARTESIAN_POINT('Ctrl Pts',(1.69209406918464,1.16568229956973,13.7131625524951));
#51124=CARTESIAN_POINT('Ctrl Pts',(1.73258256853702,1.10690955364262,13.7093035624738));
#51125=CARTESIAN_POINT('Ctrl Pts',(1.76999029517012,1.0460467934869,13.7054445724524));
#51126=CARTESIAN_POINT('Ctrl Pts',(1.80411050084976,0.983454555749083,13.7015855824311));
#51127=CARTESIAN_POINT('Ctrl Pts',(1.83824708918921,0.920832264636221,13.6977247395335));
#51128=CARTESIAN_POINT('Ctrl Pts',(1.86909280168606,0.856479280384039,13.6938638966358));
#51129=CARTESIAN_POINT('Ctrl Pts',(1.89648806240337,0.790778471925942,13.6900030537382));
#51130=CARTESIAN_POINT('Ctrl Pts',(1.92393375738292,0.724956709269307,13.6861351030869));
#51131=CARTESIAN_POINT('Ctrl Pts',(1.94791614522091,0.657782623450311,13.6822671524356));
#51132=CARTESIAN_POINT('Ctrl Pts',(1.96832494877896,0.589656220618669,13.6783992017844));
#51133=CARTESIAN_POINT('Ctrl Pts',(1.98628939303304,0.529689306712218,13.6749945149955));
#51134=CARTESIAN_POINT('Ctrl Pts',(2.00148572043799,0.468984962301845,13.6715898282065));
#51135=CARTESIAN_POINT('Ctrl Pts',(2.01387175448042,0.407821185087241,13.6681851414176));
#51136=CARTESIAN_POINT('Ctrl Pts',(2.02794723185223,0.338314726505752,13.6643160585706));
#51137=CARTESIAN_POINT('Ctrl Pts',(2.03844765063878,0.267942577620449,13.6604469757236));
#51138=CARTESIAN_POINT('Ctrl Pts',(2.04527430002851,0.197105555839729,13.6565778928766));
#51139=CARTESIAN_POINT('Ctrl Pts',(2.05209077805113,0.126374077688449,13.6527145747701));
#51140=CARTESIAN_POINT('Ctrl Pts',(2.05524430566592,0.0551795811115907,
13.6488512566636));
#51141=CARTESIAN_POINT('Ctrl Pts',(2.05468718187911,-0.0160669574493126,
13.6449879385571));
#51142=CARTESIAN_POINT('Ctrl Pts',(2.05413071159829,-0.0872299238477516,
13.6411291521212));
#51143=CARTESIAN_POINT('Ctrl Pts',(2.0498722394188,-0.158444327562999,13.6372703656854));
#51144=CARTESIAN_POINT('Ctrl Pts',(2.04191600564024,-0.229295853451868,
13.6334115792495));
#51145=CARTESIAN_POINT('Ctrl Pts',(2.03396478370555,-0.300102748074791,
13.6295552235662));
#51146=CARTESIAN_POINT('Ctrl Pts',(2.02232047558545,-0.370546736775478,
13.6256988678828));
#51147=CARTESIAN_POINT('Ctrl Pts',(2.00703930184062,-0.440216768611935,
13.6218425121994));
#51148=CARTESIAN_POINT('Ctrl Pts',(1.9917626423075,-0.509866219223458,13.6179872957222));
#51149=CARTESIAN_POINT('Ctrl Pts',(1.97285135408459,-0.578741692629017,
13.6141320792449));
#51150=CARTESIAN_POINT('Ctrl Pts',(1.95041278457433,-0.646442211082326,
13.6102768627676));
#51151=CARTESIAN_POINT('Ctrl Pts',(1.92797333778316,-0.714145376423281,
13.6064214955629));
#51152=CARTESIAN_POINT('Ctrl Pts',(1.9020064908327,-0.780673035187002,13.6025661283582));
#51153=CARTESIAN_POINT('Ctrl Pts',(1.87266895251019,-0.845640914812181,
13.5987107611535));
#51154=CARTESIAN_POINT('Ctrl Pts',(1.84330070578498,-0.910676798091525,
13.5948513584306));
#51155=CARTESIAN_POINT('Ctrl Pts',(1.81055492495604,-0.974149199427638,
13.5909919557078));
#51156=CARTESIAN_POINT('Ctrl Pts',(1.77463546152237,-1.03569616259176,13.5871325529849));
#51157=CARTESIAN_POINT('Ctrl Pts',(1.73869566020634,-1.09727797412989,13.5832709650379));
#51158=CARTESIAN_POINT('Ctrl Pts',(1.69957886559094,-1.1569317708205,13.5794093770909));
#51159=CARTESIAN_POINT('Ctrl Pts',(1.65753217728701,-1.21432476865054,13.5755477891439));
#51160=CARTESIAN_POINT('Ctrl Pts',(1.61541192679481,-1.27181817758742,13.5716794452104));
#51161=CARTESIAN_POINT('Ctrl Pts',(1.57035185571098,-1.32704251419185,13.5678111012768));
#51162=CARTESIAN_POINT('Ctrl Pts',(1.52263876406622,-1.37969879200603,13.5639427573433));
#51163=CARTESIAN_POINT('Ctrl Pts',(1.49430810331966,-1.41096457444656,13.5616458460375));
#51164=CARTESIAN_POINT('Ctrl Pts',(1.4650427907852,-1.44132565585821,13.5593489347318));
#51165=CARTESIAN_POINT('Ctrl Pts',(1.43490847440599,-1.47072609026218,13.557052023426));
#51166=CARTESIAN_POINT('Ctrl Pts',(1.38414806136217,-1.52025029964636,13.5531829405791));
#51167=CARTESIAN_POINT('Ctrl Pts',(1.33072131183898,-1.56724051744266,13.5493138577322));
#51168=CARTESIAN_POINT('Ctrl Pts',(1.27491142699772,-1.61139641795885,13.5454447748853));
#51169=CARTESIAN_POINT('Ctrl Pts',(1.2191846961016,-1.65548652838537,13.5415814567789));
#51170=CARTESIAN_POINT('Ctrl Pts',(1.16108225589559,-1.69675040509438,13.5377181386725));
#51171=CARTESIAN_POINT('Ctrl Pts',(1.1009235092021,-1.73492506736923,13.5338548205661));
#51172=CARTESIAN_POINT('Ctrl Pts',(1.04083532869523,-1.77305495077999,13.5299960341304));
#51173=CARTESIAN_POINT('Ctrl Pts',(0.978696041021966,-1.80810255853046,
13.5261372476946));
#51174=CARTESIAN_POINT('Ctrl Pts',(0.914856025893739,-1.83984673665659,
13.5222784612589));
#51175=CARTESIAN_POINT('Ctrl Pts',(0.851056225293838,-1.87157091827821,
13.5184221055756));
#51176=CARTESIAN_POINT('Ctrl Pts',(0.785558256695593,-1.89999558300651,
13.5145657498924));
#51177=CARTESIAN_POINT('Ctrl Pts',(0.718737950517666,-1.92494501765262,
13.5107093942091));
#51178=CARTESIAN_POINT('Ctrl Pts',(0.651937383727202,-1.94988708198595,
13.5068541777319));
#51179=CARTESIAN_POINT('Ctrl Pts',(0.583815709716312,-1.97135578452716,
13.5029989612548));
#51180=CARTESIAN_POINT('Ctrl Pts',(0.514768026271573,-1.98922382894145,
13.4991437447776));
#51181=CARTESIAN_POINT('Ctrl Pts',(0.445717643268803,-2.00709257194285,
13.495288377573));
#51182=CARTESIAN_POINT('Ctrl Pts',(0.375741649796778,-2.02136025775853,
13.4914330103683));
#51183=CARTESIAN_POINT('Ctrl Pts',(0.305247881707282,-2.03195012074933,
13.4875776431637));
#51184=CARTESIAN_POINT('Ctrl Pts',(0.234680325865516,-2.04255106843894,
13.483718240441));
#51185=CARTESIAN_POINT('Ctrl Pts',(0.163594394891996,-2.0494664361701,13.4798588377182));
#51186=CARTESIAN_POINT('Ctrl Pts',(0.0924047452284538,-2.0526711683948,
13.4759994349954));
#51187=CARTESIAN_POINT('Ctrl Pts',(0.0211747874261737,-2.05587771516405,
13.4721378470485));
#51188=CARTESIAN_POINT('Ctrl Pts',(-0.050158519971401,-2.05536944746468,
13.4682762591017));
#51189=CARTESIAN_POINT('Ctrl Pts',(-0.121181572141126,-2.05117346635369,
13.4644146711548));
#51190=CARTESIAN_POINT('Ctrl Pts',(-0.192328881686445,-2.04697014422334,
13.4605463272213));
#51191=CARTESIAN_POINT('Ctrl Pts',(-0.263164369343408,-2.03906628139337,
13.4566779832879));
#51192=CARTESIAN_POINT('Ctrl Pts',(-0.333281292006573,-2.02754066368555,
13.4528096393545));
#51193=CARTESIAN_POINT('Ctrl Pts',(-0.374914702899041,-2.02069708356831,
13.4505127280478));
#51194=CARTESIAN_POINT('Ctrl Pts',(-0.416294981267516,-2.01257757953319,
13.4482158167411));
#51195=CARTESIAN_POINT('Ctrl Pts',(-0.457339518892111,-2.00320696059083,
13.4459189054345));
#51196=CARTESIAN_POINT('Ctrl Pts',(-0.526477894423543,-1.98742241509723,
13.4420498225876));
#51197=CARTESIAN_POINT('Ctrl Pts',(-0.594933548236747,-1.96802340496217,
13.4381807397407));
#51198=CARTESIAN_POINT('Ctrl Pts',(-0.66230056404705,-1.94508496610378,
13.4343116568937));
#51199=CARTESIAN_POINT('Ctrl Pts',(-0.729567206363272,-1.9221807043754,
13.4304483387873));
#51200=CARTESIAN_POINT('Ctrl Pts',(-0.795747974224224,-1.8957476371241,
13.4265850206809));
#51201=CARTESIAN_POINT('Ctrl Pts',(-0.860448691025966,-1.86591146966079,
13.4227217025745));
#51202=CARTESIAN_POINT('Ctrl Pts',(-0.925073513912106,-1.8361103000103,
13.4188629161387));
#51203=CARTESIAN_POINT('Ctrl Pts',(-0.988221295223039,-1.8029141617238,
13.4150041297029));
#51204=CARTESIAN_POINT('Ctrl Pts',(-1.04951619713821,-1.7664974708288,13.4111453432672));
#51205=CARTESIAN_POINT('Ctrl Pts',(-1.11077248775972,-1.73010371977875,
13.4072889875839));
#51206=CARTESIAN_POINT('Ctrl Pts',(-1.17017779800132,-1.69049368859268,
13.4034326319006));
#51207=CARTESIAN_POINT('Ctrl Pts',(-1.22738066237806,-1.64788782146128,
13.3995762762173));
#51208=CARTESIAN_POINT('Ctrl Pts',(-1.2845666284559,-1.60529454052963,13.3957210597401));
#51209=CARTESIAN_POINT('Ctrl Pts',(-1.33955105095852,-1.55970747064193,
13.3918658432629));
#51210=CARTESIAN_POINT('Ctrl Pts',(-1.39201269076037,-1.51138950349077,
13.3880106267857));
#51211=CARTESIAN_POINT('Ctrl Pts',(-1.44447638165533,-1.4630696472517,13.3841552595811));
#51212=CARTESIAN_POINT('Ctrl Pts',(-1.49441673819649,-1.4120190124909,13.3802998923765));
#51213=CARTESIAN_POINT('Ctrl Pts',(-1.54154806489132,-1.35853859942581,
13.3764445251719));
#51214=CARTESIAN_POINT('Ctrl Pts',(-1.58872872523317,-1.30500220695156,
13.3725851224491));
#51215=CARTESIAN_POINT('Ctrl Pts',(-1.63309416441128,-1.24903132434447,
13.3687257197263));
#51216=CARTESIAN_POINT('Ctrl Pts',(-1.67439843093734,-1.19096072856101,
13.3648663170035));
#51217=CARTESIAN_POINT('Ctrl Pts',(-1.71572608426352,-1.13285725275011,
13.3610047290566));
#51218=CARTESIAN_POINT('Ctrl Pts',(-1.75398885386358,-1.07265210726469,
13.3571431411097));
#51219=CARTESIAN_POINT('Ctrl Pts',(-1.78898517711555,-1.01070747427772,
13.3532815531627));
#51220=CARTESIAN_POINT('Ctrl Pts',(-1.82404272768947,-0.94865446693497,
13.3494132092293));
#51221=CARTESIAN_POINT('Ctrl Pts',(-1.85582220556054,-0.884856331025426,
13.3455448652958));
#51222=CARTESIAN_POINT('Ctrl Pts',(-1.88416919184789,-0.819697516765346,
13.3416765213624));
#51223=CARTESIAN_POINT('Ctrl Pts',(-1.9010008165506,-0.78100808796392,13.3393796100559));
#51224=CARTESIAN_POINT('Ctrl Pts',(-1.916623201266,-0.741839288145892,13.3370826987494));
#51225=CARTESIAN_POINT('Ctrl Pts',(-1.93101238379182,-0.702273975128398,
13.3347857874429));
#51226=CARTESIAN_POINT('Ctrl Pts',(-1.95903836976884,-0.625212133302755,
13.330312065329));
#51227=CARTESIAN_POINT('Ctrl Pts',(-1.98247429587934,-0.546396960948768,
13.3258383432151));
#51228=CARTESIAN_POINT('Ctrl Pts',(-2.00112975528962,-0.466344577533057,
13.3213646211012));
#51229=CARTESIAN_POINT('Ctrl Pts',(-2.01962152623802,-0.3869945971632,13.3169301527347));
#51230=CARTESIAN_POINT('Ctrl Pts',(-2.03341626232235,-0.306429189566792,
13.3124956843683));
#51231=CARTESIAN_POINT('Ctrl Pts',(-2.04237487167497,-0.225172036564603,
13.3080612160018));
#51232=CARTESIAN_POINT('Ctrl Pts',(-2.05054728051348,-0.151045947430806,
13.3040159130931));
#51233=CARTESIAN_POINT('Ctrl Pts',(-2.05469557909877,-0.0763445280967105,
13.2999706101844));
#51234=CARTESIAN_POINT('Ctrl Pts',(-2.05474946769684,-0.00147901978776689,
13.2959253072757));
#51235=CARTESIAN_POINT('Ctrl Pts',(-2.05258179091604,-0.00147696517085403,
13.2959252805377));
#51236=CARTESIAN_POINT('Ctrl Pts',(-2.04962018460403,0.443899356040318,
13.2718344101756));
#51237=CARTESIAN_POINT('Ctrl Pts',(-1.68832798325332,1.5785041446152,13.2106991671496));
#51238=CARTESIAN_POINT('Ctrl Pts',(-0.112928914327977,2.28830665208722,
13.1280482345611));
#51239=CARTESIAN_POINT('Ctrl Pts',(0.93349584868275,1.86810178948702,13.0694881723346));
#51240=CARTESIAN_POINT('Ctrl Pts',(1.25024324817659,1.62681756561327,13.047972482772));
#51241=CARTESIAN_POINT('',(-2.0547492176368,0.001793075842144,13.3540747194623));
#51242=CARTESIAN_POINT('Ctrl Pts',(-2.0547492176368,0.001793075842144,13.3540747194623));
#51243=CARTESIAN_POINT('Ctrl Pts',(-2.05465860807767,0.105625784059886,
13.3484351428617));
#51244=CARTESIAN_POINT('Ctrl Pts',(-2.04669415459996,0.209126407407667,
13.3427955662611));
#51245=CARTESIAN_POINT('Ctrl Pts',(-2.03102549815175,0.31134063075262,13.3371559896605));
#51246=CARTESIAN_POINT('Ctrl Pts',(-2.02681271789171,0.338822633681565,
13.3356396951998));
#51247=CARTESIAN_POINT('Ctrl Pts',(-2.02204324664326,0.366211817300818,
13.3341234007392));
#51248=CARTESIAN_POINT('Ctrl Pts',(-2.01672090784174,0.393489952062285,
13.3326071062786));
#51249=CARTESIAN_POINT('Ctrl Pts',(-2.00314005643268,0.463094745880791,
13.3287380234317));
#51250=CARTESIAN_POINT('Ctrl Pts',(-1.98592488139643,0.532131952383038,
13.3248689405848));
#51251=CARTESIAN_POINT('Ctrl Pts',(-1.9651374895038,0.600193477011109,13.3209998577379));
#51252=CARTESIAN_POINT('Ctrl Pts',(-1.94438106978837,0.668153593361924,
13.3171365396314));
#51253=CARTESIAN_POINT('Ctrl Pts',(-1.92006313882444,0.735140452615142,
13.313273221525));
#51254=CARTESIAN_POINT('Ctrl Pts',(-1.89229682005128,0.800756084787251,
13.3094099034186));
#51255=CARTESIAN_POINT('Ctrl Pts',(-1.86456307115937,0.866294749848045,
13.3055511169828));
#51256=CARTESIAN_POINT('Ctrl Pts',(-1.8333891575092,0.930464937546923,13.3016923305471));
#51257=CARTESIAN_POINT('Ctrl Pts',(-1.79893747109799,0.992885460453303,
13.2978335441113));
#51258=CARTESIAN_POINT('Ctrl Pts',(-1.76450748672299,1.05526666300735,13.2939771884281));
#51259=CARTESIAN_POINT('Ctrl Pts',(-1.72680406021419,1.11589996313947,13.2901208327448));
#51260=CARTESIAN_POINT('Ctrl Pts',(-1.68603636254319,1.17442707167458,13.2862644770616));
#51261=CARTESIAN_POINT('Ctrl Pts',(-1.64528070805828,1.23293689071581,13.2824092605844));
#51262=CARTESIAN_POINT('Ctrl Pts',(-1.60146285702327,1.28934135498523,13.2785540441072));
#51263=CARTESIAN_POINT('Ctrl Pts',(-1.5548353664441,1.34331103835063,13.27469882763));
#51264=CARTESIAN_POINT('Ctrl Pts',(-1.50820605286951,1.39728283176923,13.2708434604254));
#51265=CARTESIAN_POINT('Ctrl Pts',(-1.4587672009129,1.448819289138,13.2669880932208));
#51266=CARTESIAN_POINT('Ctrl Pts',(-1.40681058569492,1.49762529975849,13.2631327260162));
#51267=CARTESIAN_POINT('Ctrl Pts',(-1.35479958606871,1.54648239696333,13.2592733232934));
#51268=CARTESIAN_POINT('Ctrl Pts',(-1.30026591710236,1.59260300886624,13.2554139205707));
#51269=CARTESIAN_POINT('Ctrl Pts',(-1.24353637582797,1.63573067602605,13.2515545178479));
#51270=CARTESIAN_POINT('Ctrl Pts',(-1.18677471384167,1.67888276240979,13.247692929901));
#51271=CARTESIAN_POINT('Ctrl Pts',(-1.1278151061779,1.71903825698381,13.2438313419541));
#51272=CARTESIAN_POINT('Ctrl Pts',(-1.06701315098567,1.75598419643333,13.2399697540072));
#51273=CARTESIAN_POINT('Ctrl Pts',(-1.00610482059348,1.7929947741282,13.2361014100738));
#51274=CARTESIAN_POINT('Ctrl Pts',(-0.943348135217372,1.82678435536032,
13.2322330661404));
#51275=CARTESIAN_POINT('Ctrl Pts',(-0.879122447032021,1.85718638957549,
13.2283647222069));
#51276=CARTESIAN_POINT('Ctrl Pts',(-0.840987081638146,1.87523824259988,
13.2260678109003));
#51277=CARTESIAN_POINT('Ctrl Pts',(-0.802334183373884,1.89209668972226,
13.2237708995936));
#51278=CARTESIAN_POINT('Ctrl Pts',(-0.763245807256644,1.90773514938661,
13.221473988287));
#51279=CARTESIAN_POINT('Ctrl Pts',(-0.697402531066169,1.93407769725264,
13.2176049054401));
#51280=CARTESIAN_POINT('Ctrl Pts',(-0.630064918141975,1.95705908143398,
13.2137358225932));
#51281=CARTESIAN_POINT('Ctrl Pts',(-0.561609507711247,1.97651013742615,
13.2098667397462));
#51282=CARTESIAN_POINT('Ctrl Pts',(-0.493256092428051,1.99593221231496,
13.2060034216398));
#51283=CARTESIAN_POINT('Ctrl Pts',(-0.423788649014342,2.01183426830099,
13.2021401035334));
#51284=CARTESIAN_POINT('Ctrl Pts',(-0.353602881144418,2.02409549304038,
13.1982767854269));
#51285=CARTESIAN_POINT('Ctrl Pts',(-0.283499441153164,2.03634233536786,
13.1944179989912));
#51286=CARTESIAN_POINT('Ctrl Pts',(-0.21267982659666,2.04495674629938,13.1905592125554));
#51287=CARTESIAN_POINT('Ctrl Pts',(-0.141552363867611,2.0498684081627,13.1867004261196));
#51288=CARTESIAN_POINT('Ctrl Pts',(-0.070469706224526,2.05477697603921,
13.1828440704363));
#51289=CARTESIAN_POINT('Ctrl Pts',(0.000919931369931917,2.05598738902582,
13.1789877147531));
#51290=CARTESIAN_POINT('Ctrl Pts',(0.072202088109846,2.05348104957718,13.1751313590698));
#51291=CARTESIAN_POINT('Ctrl Pts',(0.143463187386881,2.0509754505263,13.1712761425926));
#51292=CARTESIAN_POINT('Ctrl Pts',(0.214616383625109,2.04475529586794,13.1674209261154));
#51293=CARTESIAN_POINT('Ctrl Pts',(0.285247933084463,2.03485409284574,13.1635657096382));
#51294=CARTESIAN_POINT('Ctrl Pts',(0.355882244026187,2.0249525027161,13.1597103424336));
#51295=CARTESIAN_POINT('Ctrl Pts',(0.425994386924309,2.01136964811211,13.1558549752289));
#51296=CARTESIAN_POINT('Ctrl Pts',(0.495178176436132,1.99419059672875,13.1519996080243));
#51297=CARTESIAN_POINT('Ctrl Pts',(0.564434382510014,1.97699356356312,13.1481402053015));
#51298=CARTESIAN_POINT('Ctrl Pts',(0.632759822969506,1.9561929366664,13.1442808025787));
#51299=CARTESIAN_POINT('Ctrl Pts',(0.699761789476065,1.93192417048114,13.140421399856));
#51300=CARTESIAN_POINT('Ctrl Pts',(0.766801693022361,1.90764166312985,13.136559811909));
#51301=CARTESIAN_POINT('Ctrl Pts',(0.832516183149191,1.87988729648662,13.1326982239621));
#51302=CARTESIAN_POINT('Ctrl Pts',(0.89653347289356,1.84884431320796,13.1288366360152));
#51303=CARTESIAN_POINT('Ctrl Pts',(0.960662763180963,1.81774701911736,13.1249682920817));
#51304=CARTESIAN_POINT('Ctrl Pts',(1.0230884991648,1.78334985577258,13.1210999481483));
#51305=CARTESIAN_POINT('Ctrl Pts',(1.08346500306139,1.74588119574076,13.1172316042149));
#51306=CARTESIAN_POINT('Ctrl Pts',(1.11931483359134,1.72363338366761,13.1149346929084));
#51307=CARTESIAN_POINT('Ctrl Pts',(1.15444274399193,1.70030349523615,13.1126377816019));
#51308=CARTESIAN_POINT('Ctrl Pts',(1.18878189719209,1.67594605026784,13.1103408702954));
#51309=CARTESIAN_POINT('Ctrl Pts',(1.21015704796113,1.66078423030358,13.1089111080298));
#51310=CARTESIAN_POINT('Ctrl Pts',(1.23125751467611,1.64520247351562,13.1074813457642));
#51311=CARTESIAN_POINT('Ctrl Pts',(1.25206542099588,1.62921138715834,13.1060515834985));
#51312=CARTESIAN_POINT('Ctrl Pts',(1.2517190174544,1.62874802847342,13.8061758215988));
#51313=CARTESIAN_POINT('Ctrl Pts',(1.39438384162289,1.52131572678504,13.7964970738141));
#51314=CARTESIAN_POINT('Ctrl Pts',(2.01423952061842,0.915915198607634,13.7497739533656));
#51315=CARTESIAN_POINT('Ctrl Pts',(2.28817075268951,-0.813789378500904,
13.6660064602532));
#51316=CARTESIAN_POINT('Ctrl Pts',(0.55736741032268,-2.36375128050173,13.5548733422617));
#51317=CARTESIAN_POINT('Ctrl Pts',(-1.53926415431828,-1.78981496460753,
13.4508962354953));
#51318=CARTESIAN_POINT('Ctrl Pts',(-2.05053220286094,-0.548727178269576,
13.3839635013926));
#51319=CARTESIAN_POINT('Ctrl Pts',(-2.05557322758416,0.00178604994939961,
13.3540751399538));
#51320=CARTESIAN_POINT('Origin',(0.,0.,18.5459252805377));
#51321=CARTESIAN_POINT('',(1.25206542099588,1.62921138715834,14.5060551473646));
#51322=CARTESIAN_POINT('',(1.25206542099587,1.62921138715835,14.4479364137113));
#51323=CARTESIAN_POINT('',(1.25206542099588,1.62921138715835,18.5459252805377));
#51324=CARTESIAN_POINT('',(-2.05474990309271,-0.000631062987199567,13.9959252805008));
#51325=CARTESIAN_POINT('Ctrl Pts',(1.25206542099587,1.62921138715835,14.4479364137114));
#51326=CARTESIAN_POINT('Ctrl Pts',(1.26088488177545,1.62243354239187,14.4473299315937));
#51327=CARTESIAN_POINT('Ctrl Pts',(1.26964669655897,1.61558608613413,14.4467234494761));
#51328=CARTESIAN_POINT('Ctrl Pts',(1.27834972325942,1.60867011768808,14.4461169673585));
#51329=CARTESIAN_POINT('Ctrl Pts',(1.33387111508418,1.56454935290619,14.4422478845157));
#51330=CARTESIAN_POINT('Ctrl Pts',(1.38721440473503,1.51746441295354,14.438378801673));
#51331=CARTESIAN_POINT('Ctrl Pts',(1.43804599837291,1.46765843065192,14.4345097188302));
#51332=CARTESIAN_POINT('Ctrl Pts',(1.4888018554701,1.41792665678123,14.430646400728));
#51333=CARTESIAN_POINT('Ctrl Pts',(1.53705310076354,1.36548222528367,14.4267830826258));
#51334=CARTESIAN_POINT('Ctrl Pts',(1.58249862997129,1.31060888469406,14.4229197645236));
#51335=CARTESIAN_POINT('Ctrl Pts',(1.62789085158941,1.25579991051348,14.4190609780921));
#51336=CARTESIAN_POINT('Ctrl Pts',(1.67048358601886,1.19856805885492,14.4152021916607));
#51337=CARTESIAN_POINT('Ctrl Pts',(1.71001332250266,1.13923307508315,14.4113434052293));
#51338=CARTESIAN_POINT('Ctrl Pts',(1.74951815815035,1.07993546800138,14.4074870495504));
#51339=CARTESIAN_POINT('Ctrl Pts',(1.78596355517878,1.01853776055163,14.4036306938715));
#51340=CARTESIAN_POINT('Ctrl Pts',(1.81912787742638,0.955390667774294,14.3997743381926));
#51341=CARTESIAN_POINT('Ctrl Pts',(1.85228240260056,0.89226222928148,14.3959191217199));
#51342=CARTESIAN_POINT('Ctrl Pts',(1.88215755149882,0.827385861267853,14.3920639052472));
#51343=CARTESIAN_POINT('Ctrl Pts',(1.90857729350246,0.761137489043105,14.3882086887745));
#51344=CARTESIAN_POINT('Ctrl Pts',(1.93499806843862,0.694886526706072,14.3843533215744));
#51345=CARTESIAN_POINT('Ctrl Pts',(1.95796299036314,0.627263905701272,14.3804979543743));
#51346=CARTESIAN_POINT('Ctrl Pts',(1.9773445533335,0.558664550425702,14.3766425871741));
#51347=CARTESIAN_POINT('Ctrl Pts',(1.99674640351495,0.489993390332135,14.3727831844559));
#51348=CARTESIAN_POINT('Ctrl Pts',(2.01255727495578,0.420343923520013,14.3689237817377));
#51349=CARTESIAN_POINT('Ctrl Pts',(2.02470010147728,0.350124351592271,14.3650643790195));
#51350=CARTESIAN_POINT('Ctrl Pts',(2.03684980336243,0.279865020791915,14.3612027910772));
#51351=CARTESIAN_POINT('Ctrl Pts',(2.04532726815123,0.209035424853614,14.3573412031349));
#51352=CARTESIAN_POINT('Ctrl Pts',(2.05010730359109,0.138049289250118,14.3534796151926));
#51353=CARTESIAN_POINT('Ctrl Pts',(2.05489570187429,0.0669389608579706,
14.3496112712638));
#51354=CARTESIAN_POINT('Ctrl Pts',(2.05597374834625,-0.00432796811090772,
14.3457429273349));
#51355=CARTESIAN_POINT('Ctrl Pts',(2.05336838815399,-0.0753380715833479,
14.3418745834061));
#51356=CARTESIAN_POINT('Ctrl Pts',(2.0518214002188,-0.117501828316216,14.3395776720597));
#51357=CARTESIAN_POINT('Ctrl Pts',(2.04897677048839,-0.159575120644791,
14.3372807607133));
#51358=CARTESIAN_POINT('Ctrl Pts',(2.04484870920189,-0.201472874043492,
14.3349838493669));
#51359=CARTESIAN_POINT('Ctrl Pts',(2.03789510554898,-0.272048466522004,
14.3311147665166));
#51360=CARTESIAN_POINT('Ctrl Pts',(2.02726984051678,-0.342401873588419,
14.3272456836663));
#51361=CARTESIAN_POINT('Ctrl Pts',(2.01299624329973,-0.412120961564876,
14.3233766008159));
#51362=CARTESIAN_POINT('Ctrl Pts',(1.99874391303048,-0.481736171578308,
14.319513282706));
#51363=CARTESIAN_POINT('Ctrl Pts',(1.98085413719419,-0.550718466471994,
14.3156499645961));
#51364=CARTESIAN_POINT('Ctrl Pts',(1.95940198928566,-0.618660978956498,
14.3117866464862));
#51365=CARTESIAN_POINT('Ctrl Pts',(1.93797500473801,-0.686523794901137,
14.3079278600469));
#51366=CARTESIAN_POINT('Ctrl Pts',(1.91299409390747,-0.753348790110171,
14.3040690736076));
#51367=CARTESIAN_POINT('Ctrl Pts',(1.88458496240443,-0.81874115688604,14.3002102871683));
#51368=CARTESIAN_POINT('Ctrl Pts',(1.85619372657082,-0.88409233126648,14.2963539314815));
#51369=CARTESIAN_POINT('Ctrl Pts',(1.82437874764256,-0.948012223162581,
14.2924975757947));
#51370=CARTESIAN_POINT('Ctrl Pts',(1.78931446183537,-1.01012440776709,14.2886412201078));
#51371=CARTESIAN_POINT('Ctrl Pts',(1.75426053436903,-1.0722182438108,14.284786003627));
#51372=CARTESIAN_POINT('Ctrl Pts',(1.71595944433067,-1.13250500993205,14.2809307871463));
#51373=CARTESIAN_POINT('Ctrl Pts',(1.67463154346597,-1.19063292249492,14.2770755706655));
#51374=CARTESIAN_POINT('Ctrl Pts',(1.63330202680369,-1.24876310768569,14.2732202034572));
#51375=CARTESIAN_POINT('Ctrl Pts',(1.58894574765226,-1.30473387710441,14.269364836249));
#51376=CARTESIAN_POINT('Ctrl Pts',(1.54182533834839,-1.35822390956972,14.2655094690408));
#51377=CARTESIAN_POINT('Ctrl Pts',(1.494655606825,-1.41176993151312,14.2616500663143));
#51378=CARTESIAN_POINT('Ctrl Pts',(1.44471629126146,-1.4628296677331,14.2577906635879));
#51379=CARTESIAN_POINT('Ctrl Pts',(1.39230853614955,-1.5111169718672,14.2539312608615));
#51380=CARTESIAN_POINT('Ctrl Pts',(1.33987110735488,-1.55943161665233,14.250069672911));
#51381=CARTESIAN_POINT('Ctrl Pts',(1.28496283081743,-1.6049703941579,14.2462080849604));
#51382=CARTESIAN_POINT('Ctrl Pts',(1.22791762721129,-1.64748774298439,14.2423464970099));
#51383=CARTESIAN_POINT('Ctrl Pts',(1.17077262097713,-1.69007947743633,14.2384781530728));
#51384=CARTESIAN_POINT('Ctrl Pts',(1.11148362761128,-1.72963895965841,14.2346098091357));
#51385=CARTESIAN_POINT('Ctrl Pts',(1.05041259455181,-1.76596459299357,14.2307414651987));
#51386=CARTESIAN_POINT('Ctrl Pts',(1.01415037313166,-1.78753370838652,14.2284445539242));
#51387=CARTESIAN_POINT('Ctrl Pts',(0.977260338518683,-1.80796356594284,
14.2261476426498));
#51388=CARTESIAN_POINT('Ctrl Pts',(0.939821671982243,-1.82721996140927,
14.2238507313754));
#51389=CARTESIAN_POINT('Ctrl Pts',(0.876757284563182,-1.85965682138151,
14.2199816485293));
#51390=CARTESIAN_POINT('Ctrl Pts',(0.811888125585217,-1.88888848819301,
14.2161125656831));
#51391=CARTESIAN_POINT('Ctrl Pts',(0.745573095478381,-1.91471102827523,
14.212243482837));
#51392=CARTESIAN_POINT('Ctrl Pts',(0.679356871459215,-1.94049509406051,
14.2083801647314));
#51393=CARTESIAN_POINT('Ctrl Pts',(0.611699501476661,-1.96287994081013,
14.2045168466258));
#51394=CARTESIAN_POINT('Ctrl Pts',(0.54298352658394,-1.98170796343923,14.2006535285201));
#51395=CARTESIAN_POINT('Ctrl Pts',(0.474348155503365,-2.00051390080502,
14.1967947420852));
#51396=CARTESIAN_POINT('Ctrl Pts',(0.404657112275731,-2.01577117361054,
14.1929359556502));
#51397=CARTESIAN_POINT('Ctrl Pts',(0.334310268155385,-2.02737125537132,
14.1890771692152));
#51398=CARTESIAN_POINT('Ctrl Pts',(0.264007737388558,-2.03896402993118,
14.1852208135327));
#51399=CARTESIAN_POINT('Ctrl Pts',(0.193050703503013,-2.04690410522378,
14.1813644578503));
#51400=CARTESIAN_POINT('Ctrl Pts',(0.121850024200273,-2.05113386547597,
14.1775081021678));
#51401=CARTESIAN_POINT('Ctrl Pts',(0.0506703782911608,-2.05536237621463,
14.1736528856914));
#51402=CARTESIAN_POINT('Ctrl Pts',(-0.0207522854801669,-2.05588271911257,
14.169797669215));
#51403=CARTESIAN_POINT('Ctrl Pts',(-0.0920029075953569,-2.05268921843858,
14.1659424527386));
#51404=CARTESIAN_POINT('Ctrl Pts',(-0.163256315396763,-2.04949559290827,
14.1620870855348));
#51405=CARTESIAN_POINT('Ctrl Pts',(-0.234337182990594,-2.04258785948211,
14.158231718331));
#51406=CARTESIAN_POINT('Ctrl Pts',(-0.304833111213674,-2.03201238598779,
14.1543763511271));
#51407=CARTESIAN_POINT('Ctrl Pts',(-0.375402829450457,-2.02142584285649,
14.1505169484051));
#51408=CARTESIAN_POINT('Ctrl Pts',(-0.445385904692635,-2.00716396812194,
14.1466575456832));
#51409=CARTESIAN_POINT('Ctrl Pts',(-0.514378601070832,-1.98932456307673,
14.1427981429612));
#51410=CARTESIAN_POINT('Ctrl Pts',(-0.583410361655732,-1.97147505722023,
14.138936555015));
#51411=CARTESIAN_POINT('Ctrl Pts',(-0.651450163514077,-1.95004413466785,
14.1350749670689));
#51412=CARTESIAN_POINT('Ctrl Pts',(-0.718110590390047,-1.92517914555235,
14.1312133791228));
#51413=CARTESIAN_POINT('Ctrl Pts',(-0.784887642072441,-1.90027065424704,
14.1273450351901));
#51414=CARTESIAN_POINT('Ctrl Pts',(-0.850280054788644,-1.87191629450514,
14.1234766912574));
#51415=CARTESIAN_POINT('Ctrl Pts',(-0.913922147352021,-1.84031080828198,
14.1196083473248));
#51416=CARTESIAN_POINT('Ctrl Pts',(-0.951710990582568,-1.82154438002661,
14.1173114360111));
#51417=CARTESIAN_POINT('Ctrl Pts',(-0.988883219120611,-1.80163259407143,
14.1150145246975));
#51418=CARTESIAN_POINT('Ctrl Pts',(-1.02536715047564,-1.78062342150873,
14.1127176133838));
#51419=CARTESIAN_POINT('Ctrl Pts',(-1.08682331212073,-1.74523405810712,
14.1088485305374));
#51420=CARTESIAN_POINT('Ctrl Pts',(-1.14656555754676,-1.70659001272789,
14.1049794476909));
#51421=CARTESIAN_POINT('Ctrl Pts',(-1.20422789488691,-1.66488219993975,
14.1011103648445));
#51422=CARTESIAN_POINT('Ctrl Pts',(-1.26180431821997,-1.62323652971276,
14.0972470467386));
#51423=CARTESIAN_POINT('Ctrl Pts',(-1.31730659441153,-1.57853643558272,
14.0933837286326));
#51424=CARTESIAN_POINT('Ctrl Pts',(-1.37039483147761,-1.53101782104567,
14.0895204105267));
#51425=CARTESIAN_POINT('Ctrl Pts',(-1.4234207960619,-1.48355494582533,14.0856616240914));
#51426=CARTESIAN_POINT('Ctrl Pts',(-1.47403798596418,-1.43328043969418,
14.0818028376561));
#51427=CARTESIAN_POINT('Ctrl Pts',(-1.52193834219604,-1.38047138509045,
14.0779440512208));
#51428=CARTESIAN_POINT('Ctrl Pts',(-1.56980852471574,-1.32769559631895,
14.0740876955381));
#51429=CARTESIAN_POINT('Ctrl Pts',(-1.61496494336878,-1.27238878562944,
14.0702313398553));
#51430=CARTESIAN_POINT('Ctrl Pts',(-1.6571363521066,-1.21486487850576,14.0663749841725));
#51431=CARTESIAN_POINT('Ctrl Pts',(-1.69929530298793,-1.15735796452035,
14.0625197676959));
#51432=CARTESIAN_POINT('Ctrl Pts',(-1.73847070751407,-1.09763564592932,
14.0586645512192));
#51433=CARTESIAN_POINT('Ctrl Pts',(-1.77443267720094,-1.03604354955837,
14.0548093347425));
#51434=CARTESIAN_POINT('Ctrl Pts',(-1.81039605289318,-0.974449045120822,
14.0509539675384));
#51435=CARTESIAN_POINT('Ctrl Pts',(-1.84314550127443,-0.910985038388832,
14.0470986003343));
#51436=CARTESIAN_POINT('Ctrl Pts',(-1.87249630030024,-0.846023148537866,
14.0432432331302));
#51437=CARTESIAN_POINT('Ctrl Pts',(-1.90187782160901,-0.780993261302558,
14.0393838304079));
#51438=CARTESIAN_POINT('Ctrl Pts',(-1.92785339165058,-0.714462804719801,
14.0355244276857));
#51439=CARTESIAN_POINT('Ctrl Pts',(-1.95028619813571,-0.64682401614454,
14.0316650249634));
#51440=CARTESIAN_POINT('Ctrl Pts',(-1.97273170625206,-0.579146929955948,
14.0278034370171));
#51441=CARTESIAN_POINT('Ctrl Pts',(-1.99163032884486,-0.51036073117081,
14.0239418490707));
#51442=CARTESIAN_POINT('Ctrl Pts',(-2.00689573268168,-0.44087082081271,
14.0200802611243));
#51443=CARTESIAN_POINT('Ctrl Pts',(-2.02218784388967,-0.371259335365698,
14.0162119171914));
#51444=CARTESIAN_POINT('Ctrl Pts',(-2.03383396611622,-0.300942159688749,
14.0123435732585));
#51445=CARTESIAN_POINT('Ctrl Pts',(-2.04179937024044,-0.230332138846787,
14.0084752293256));
#51446=CARTESIAN_POINT('Ctrl Pts',(-2.0465289979953,-0.188405940359313,
14.0061783180145));
#51447=CARTESIAN_POINT('Ctrl Pts',(-2.04996193318919,-0.14637656079547,
14.0038814067033));
#51448=CARTESIAN_POINT('Ctrl Pts',(-2.05209959875135,-0.104330241562734,
14.0015844953922));
#51449=CARTESIAN_POINT('Ctrl Pts',(-2.0538552185185,-0.0697984838886084,
13.9996980904407));
#51450=CARTESIAN_POINT('Ctrl Pts',(-2.05473927936225,-0.035222040657156,
13.9978116854892));
#51451=CARTESIAN_POINT('Ctrl Pts',(-2.0547499030925,-0.000631063664673059,
13.9959252805377));
#51452=CARTESIAN_POINT('Ctrl Pts',(-2.05474990309271,-0.000631062987199567,
13.9959252805008));
#51453=CARTESIAN_POINT('Ctrl Pts',(-2.05477152045948,0.0697553852428013,
13.9920867839909));
#51454=CARTESIAN_POINT('Ctrl Pts',(-2.05117219117543,0.140288018046474,
13.988248287481));
#51455=CARTESIAN_POINT('Ctrl Pts',(-2.0439330102198,0.210559759293677,13.9844097909711));
#51456=CARTESIAN_POINT('Ctrl Pts',(-2.03654967279865,0.282230847498369,
13.9804948570723));
#51457=CARTESIAN_POINT('Ctrl Pts',(-2.02537985399478,0.353630025937492,
13.9765799231736));
#51458=CARTESIAN_POINT('Ctrl Pts',(-2.01045943330037,0.424323496348664,
13.9726649892748));
#51459=CARTESIAN_POINT('Ctrl Pts',(-1.99586784174531,0.493458962899926,
13.9688363360762));
#51460=CARTESIAN_POINT('Ctrl Pts',(-1.97768938082227,0.561918997872263,
13.9650076828776));
#51461=CARTESIAN_POINT('Ctrl Pts',(-1.95600985617612,0.629303587342279,
13.9611790296791));
#51462=CARTESIAN_POINT('Ctrl Pts',(-1.93434249883849,0.696650358220673,
13.9573525252547));
#51463=CARTESIAN_POINT('Ctrl Pts',(-1.90917812574259,0.762922411139088,
13.9535260208304));
#51464=CARTESIAN_POINT('Ctrl Pts',(-1.88065280528506,0.827733404227122,
13.9496995164061));
#51465=CARTESIAN_POINT('Ctrl Pts',(-1.85213357842264,0.892530552354134,
13.9458738294018));
#51466=CARTESIAN_POINT('Ctrl Pts',(-1.82025502876711,0.955866808207142,
13.9420481423976));
#51467=CARTESIAN_POINT('Ctrl Pts',(-1.7852012286889,1.01737610331068,13.9382224553933));
#51468=CARTESIAN_POINT('Ctrl Pts',(-1.74872503901803,1.08138128134311,13.9342415322272));
#51469=CARTESIAN_POINT('Ctrl Pts',(-1.70881064470608,1.14340753871887,13.9302606090612));
#51470=CARTESIAN_POINT('Ctrl Pts',(-1.66571685187883,1.20307311991703,13.9262796858951));
#51471=CARTESIAN_POINT('Ctrl Pts',(-1.62425181462367,1.26048360492933,13.9224492240917));
#51472=CARTESIAN_POINT('Ctrl Pts',(-1.57984378140074,1.31570830617255,13.9186187622883));
#51473=CARTESIAN_POINT('Ctrl Pts',(-1.53276463744932,1.36844076550096,13.9147883004848));
#51474=CARTESIAN_POINT('Ctrl Pts',(-1.48565311409644,1.42120949238497,13.9109552042227));
#51475=CARTESIAN_POINT('Ctrl Pts',(-1.43586717517302,1.47148221951872,13.9071221079605));
#51476=CARTESIAN_POINT('Ctrl Pts',(-1.3837146116892,1.51899026853295,13.9032890116984));
#51477=CARTESIAN_POINT('Ctrl Pts',(-1.33147845967571,1.56657446199147,13.8994497718671));
#51478=CARTESIAN_POINT('Ctrl Pts',(-1.27686850329514,1.61138483359032,13.8956105320358));
#51479=CARTESIAN_POINT('Ctrl Pts',(-1.22022357684515,1.6531944788836,13.8917712922045));
#51480=CARTESIAN_POINT('Ctrl Pts',(-1.21373214622642,1.65798580669748,13.8913313206032));
#51481=CARTESIAN_POINT('Ctrl Pts',(-1.20721401848556,1.66273777538411,13.890891349002));
#51482=CARTESIAN_POINT('Ctrl Pts',(-1.20066972439088,1.66745008184087,13.8904513774007));
#51483=CARTESIAN_POINT('Ctrl Pts',(-1.1431196098986,1.70888981119686,13.8865822945539));
#51484=CARTESIAN_POINT('Ctrl Pts',(-1.08330889157962,1.74742779385032,13.8827132117072));
#51485=CARTESIAN_POINT('Ctrl Pts',(-1.02156221766485,1.78280907501047,13.8788441288604));
#51486=CARTESIAN_POINT('Ctrl Pts',(-0.959907543214647,1.81813763982629,
13.8749808107541));
#51487=CARTESIAN_POINT('Ctrl Pts',(-0.896323056833569,1.85031859957462,
13.8711174926478));
#51488=CARTESIAN_POINT('Ctrl Pts',(-0.831163663166718,1.87913930498281,
13.8672541745415));
#51489=CARTESIAN_POINT('Ctrl Pts',(-0.766080701443692,1.90792620371459,
13.8633953881059));
#51490=CARTESIAN_POINT('Ctrl Pts',(-0.699426944037772,1.93336048186316,
13.8595366016702));
#51491=CARTESIAN_POINT('Ctrl Pts',(-0.631581719784205,1.95527545213825,
13.8556778152346));
#51492=CARTESIAN_POINT('Ctrl Pts',(-0.563779233047022,1.97717661758902,
13.8518214595515));
#51493=CARTESIAN_POINT('Ctrl Pts',(-0.494787229687997,1.99556272450761,
13.8479651038683));
#51494=CARTESIAN_POINT('Ctrl Pts',(-0.425003461262185,2.01031580116537,
13.8441087481852));
#51495=CARTESIAN_POINT('Ctrl Pts',(-0.355240307660369,2.02506451961655,
13.8402535317081));
#51496=CARTESIAN_POINT('Ctrl Pts',(-0.284686328358028,2.03618223804894,
13.8363983152311));
#51497=CARTESIAN_POINT('Ctrl Pts',(-0.213751140990927,2.04360172544091,
13.832543098754));
#51498=CARTESIAN_POINT('Ctrl Pts',(-0.142813180270208,2.05102150291265,
13.8286877315496));
#51499=CARTESIAN_POINT('Ctrl Pts',(-0.0714944652711667,2.05474271393595,
13.8248323643451));
#51500=CARTESIAN_POINT('Ctrl Pts',(-0.000209708945903632,2.05474998929849,
13.8209769971406));
#51501=CARTESIAN_POINT('Ctrl Pts',(0.0711496630808504,2.05475727227636,
13.817117594418));
#51502=CARTESIAN_POINT('Ctrl Pts',(0.142474518698766,2.05104285926674,13.8132581916953));
#51503=CARTESIAN_POINT('Ctrl Pts',(0.213351076631586,2.04364353070689,13.8093987889727));
#51504=CARTESIAN_POINT('Ctrl Pts',(0.284267765428198,2.0362400125891,13.8055372010259));
#51505=CARTESIAN_POINT('Ctrl Pts',(0.354735171141851,2.02514750106051,13.8016756130791));
#51506=CARTESIAN_POINT('Ctrl Pts',(0.424348295436333,2.01045419909539,13.7978140251324));
#51507=CARTESIAN_POINT('Ctrl Pts',(0.494083210387085,1.99573519067179,13.7939456811991));
#51508=CARTESIAN_POINT('Ctrl Pts',(0.562960390327175,1.97740293924371,13.7900773372657));
#51509=CARTESIAN_POINT('Ctrl Pts',(0.630589295530054,1.95559574116506,13.7862089933324));
#51510=CARTESIAN_POINT('Ctrl Pts',(0.670745393273935,1.94264725449446,13.7839120820247));
#51511=CARTESIAN_POINT('Ctrl Pts',(0.710461744569614,1.92847456155713,13.7816151707169));
#51512=CARTESIAN_POINT('Ctrl Pts',(0.749660339633757,1.91311446016181,13.7793182594091));
#51513=CARTESIAN_POINT('Ctrl Pts',(0.815683790416979,1.88724294877625,13.7754494980305));
#51514=CARTESIAN_POINT('Ctrl Pts',(0.880495696393577,1.85789895683121,13.7715807366518));
#51515=CARTESIAN_POINT('Ctrl Pts',(0.943705875462188,1.82521691399081,13.7677119752731));
#51516=CARTESIAN_POINT('Ctrl Pts',(1.00681605076683,1.79258657686216,13.7638493345969));
#51517=CARTESIAN_POINT('Ctrl Pts',(1.06832910357685,1.75662889722033,13.7599866939208));
#51518=CARTESIAN_POINT('Ctrl Pts',(1.12787407849864,1.71752660111884,13.7561240532446));
#51519=CARTESIAN_POINT('Ctrl Pts',(1.17031289217566,1.68965766573388,13.7533710772265));
#51520=CARTESIAN_POINT('Ctrl Pts',(1.2117523357401,1.66019240070899,13.7506181012084));
#51521=CARTESIAN_POINT('Ctrl Pts',(1.25206542099588,1.62921138715834,13.7478651251903));
#51522=CARTESIAN_POINT('',(-2.05441708793377,9.11445141410593E-5,14.0540747126079));
#51523=CARTESIAN_POINT('Ctrl Pts',(-2.05138530455185,9.21659133880177E-5,
14.0540746501851));
#51524=CARTESIAN_POINT('Ctrl Pts',(-2.05151822953231,0.337478339785075,
14.0358517048661));
#51525=CARTESIAN_POINT('Ctrl Pts',(-1.81315401936802,1.36054008639431,13.9805843868831));
#51526=CARTESIAN_POINT('Ctrl Pts',(-0.369385311720978,2.3091885410961,13.897951444021));
#51527=CARTESIAN_POINT('Ctrl Pts',(0.848349475390589,1.93250137893999,13.833541446478));
#51528=CARTESIAN_POINT('Ctrl Pts',(1.2517190174544,1.62874802847342,13.8061758215988));
#51529=CARTESIAN_POINT('Ctrl Pts',(1.25206542099588,1.62921138715834,14.5060551473646));
#51530=CARTESIAN_POINT('Ctrl Pts',(1.30860924608552,1.58575688596617,14.5022000106753));
#51531=CARTESIAN_POINT('Ctrl Pts',(1.36290092959432,1.53934552907356,14.4983448739859));
#51532=CARTESIAN_POINT('Ctrl Pts',(1.41462456046657,1.49024659550853,14.4944897372965));
#51533=CARTESIAN_POINT('Ctrl Pts',(1.46635421293839,1.44114194590786,14.490634151797));
#51534=CARTESIAN_POINT('Ctrl Pts',(1.51551486871162,1.38934943476757,14.4867785662975));
#51535=CARTESIAN_POINT('Ctrl Pts',(1.56182696774729,1.33517567582596,14.482922980798));
#51536=CARTESIAN_POINT('Ctrl Pts',(1.60818974392862,1.28094263709505,14.4790631763131));
#51537=CARTESIAN_POINT('Ctrl Pts',(1.65169742786638,1.22432352138397,14.4752033718283));
#51538=CARTESIAN_POINT('Ctrl Pts',(1.69211093219569,1.16565782099373,14.4713435673434));
#51539=CARTESIAN_POINT('Ctrl Pts',(1.73255012112508,1.10695483591169,14.4674813097791));
#51540=CARTESIAN_POINT('Ctrl Pts',(1.76989096323924,1.04620309167034,14.4636190522149));
#51541=CARTESIAN_POINT('Ctrl Pts',(1.80393932467075,0.983768507021053,14.4597567946506));
#51542=CARTESIAN_POINT('Ctrl Pts',(1.83804488750296,0.921229031988096,14.4558880484762));
#51543=CARTESIAN_POINT('Ctrl Pts',(1.86884672327517,0.857001512854926,14.4520193023018));
#51544=CARTESIAN_POINT('Ctrl Pts',(1.89619834296505,0.791472934873064,14.4481505561275));
#51545=CARTESIAN_POINT('Ctrl Pts',(1.90612510821433,0.767690547646272,14.4467464661497));
#51546=CARTESIAN_POINT('Ctrl Pts',(1.91559788850765,0.743736934848507,14.4453423761719));
#51547=CARTESIAN_POINT('Ctrl Pts',(1.92461131969351,0.719631037829523,14.4439382861942));
#51548=CARTESIAN_POINT('Ctrl Pts',(1.94944855431137,0.65320529966295,14.4400692033241));
#51549=CARTESIAN_POINT('Ctrl Pts',(1.97089148697944,0.58536210665846,14.4362001204539));
#51550=CARTESIAN_POINT('Ctrl Pts',(1.98877956645739,0.516481750443847,14.4323310375838));
#51551=CARTESIAN_POINT('Ctrl Pts',(2.00664099359071,0.44770402251835,14.4284677194539));
#51552=CARTESIAN_POINT('Ctrl Pts',(2.02095795993475,0.377892665158933,14.4246044013239));
#51553=CARTESIAN_POINT('Ctrl Pts',(2.03161869003943,0.307446029056242,14.4207410831939));
#51554=CARTESIAN_POINT('Ctrl Pts',(2.04226691511295,0.237082026823042,14.4168822967342));
#51555=CARTESIAN_POINT('Ctrl Pts',(2.04926735054969,0.166084704012999,14.4130235102745));
#51556=CARTESIAN_POINT('Ctrl Pts',(2.05255898976634,0.0948638815851162,
14.4091647238148));
#51557=CARTESIAN_POINT('Ctrl Pts',(2.05584855549185,0.02368792304854,14.4053083681074));
#51558=CARTESIAN_POINT('Ctrl Pts',(2.0554339377446,-0.0477107716659809,
14.4014520124));
#51559=CARTESIAN_POINT('Ctrl Pts',(2.05130597628203,-0.118917425845184,
14.3975956566925));
#51560=CARTESIAN_POINT('Ctrl Pts',(2.0471792342604,-0.190103044869233,14.393740440191));
#51561=CARTESIAN_POINT('Ctrl Pts',(2.03934135439014,-0.261096251279422,
14.3898852236895));
#51562=CARTESIAN_POINT('Ctrl Pts',(2.02783525140285,-0.331484171066937,
14.386030007188));
#51563=CARTESIAN_POINT('Ctrl Pts',(2.01632869856094,-0.401874842814094,
14.3821746399589));
#51564=CARTESIAN_POINT('Ctrl Pts',(2.00115371841039,-0.471659701890479,
14.3783192727298));
#51565=CARTESIAN_POINT('Ctrl Pts',(1.98240460076224,-0.5404346041629,14.3744639055007));
#51566=CARTESIAN_POINT('Ctrl Pts',(1.96363585790037,-0.609281495004617,
14.3706045027534));
#51567=CARTESIAN_POINT('Ctrl Pts',(1.94128563740345,-0.677115849095894,
14.3667451000061));
#51568=CARTESIAN_POINT('Ctrl Pts',(1.91549829606384,-0.74354814254123,14.3628856972587));
#51569=CARTESIAN_POINT('Ctrl Pts',(1.8896963537286,-0.810018050474006,14.3590241092872));
#51570=CARTESIAN_POINT('Ctrl Pts',(1.86045361564986,-0.875083874135089,
14.3551625213157));
#51571=CARTESIAN_POINT('Ctrl Pts',(1.82796173831847,-0.938378093171251,
14.3513009333442));
#51572=CARTESIAN_POINT('Ctrl Pts',(1.79541301528476,-1.00178304770901,14.3474325893863));
#51573=CARTESIAN_POINT('Ctrl Pts',(1.75960404789974,-1.06340978925443,14.3435642454284));
#51574=CARTESIAN_POINT('Ctrl Pts',(1.72077101667156,-1.12291792695777,14.3396959014705));
#51575=CARTESIAN_POINT('Ctrl Pts',(1.6977130825711,-1.15825214306729,14.3373989903812));
#51576=CARTESIAN_POINT('Ctrl Pts',(1.67358978236133,-1.19283999979394,14.3351020792919));
#51577=CARTESIAN_POINT('Ctrl Pts',(1.64845714283379,-1.22661591818314,14.3328051682026));
#51578=CARTESIAN_POINT('Ctrl Pts',(1.60612191059531,-1.2835105132577,14.3289360853596));
#51579=CARTESIAN_POINT('Ctrl Pts',(1.5607548251177,-1.33832224264501,14.3250670025165));
#51580=CARTESIAN_POINT('Ctrl Pts',(1.51258830213628,-1.39070995924401,14.3211979196735));
#51581=CARTESIAN_POINT('Ctrl Pts',(1.46449354487208,-1.4430196207578,14.3173346015709));
#51582=CARTESIAN_POINT('Ctrl Pts',(1.4136079555805,-1.49291208383262,14.3134712834684));
#51583=CARTESIAN_POINT('Ctrl Pts',(1.36020557704207,-1.54007738464132,14.3096079653658));
#51584=CARTESIAN_POINT('Ctrl Pts',(1.30686583947285,-1.58718736057056,14.3057491789339));
#51585=CARTESIAN_POINT('Ctrl Pts',(1.25101553904864,-1.63157620843339,14.3018903925019));
#51586=CARTESIAN_POINT('Ctrl Pts',(1.19296589113649,-1.67297039575867,14.29803160607));
#51587=CARTESIAN_POINT('Ctrl Pts',(1.13495281024579,-1.71433850778134,14.2941752503906));
#51588=CARTESIAN_POINT('Ctrl Pts',(1.07474352512187,-1.75271542051358,14.2903188947111));
#51589=CARTESIAN_POINT('Ctrl Pts',(1.01268153506013,-1.78786847140617,14.2864625390317));
#51590=CARTESIAN_POINT('Ctrl Pts',(0.950637878731437,-1.82301113773569,
14.2826073225583));
#51591=CARTESIAN_POINT('Ctrl Pts',(0.88674302647926,-1.8549315936393,14.278752106085));
#51592=CARTESIAN_POINT('Ctrl Pts',(0.821367123515611,-1.88344195846532,
14.2748968896116));
#51593=CARTESIAN_POINT('Ctrl Pts',(0.755988664549258,-1.91195343796153,
14.2710415224108));
#51594=CARTESIAN_POINT('Ctrl Pts',(0.689129486072411,-1.93705436951408,
14.2671861552099));
#51595=CARTESIAN_POINT('Ctrl Pts',(0.621180263872119,-1.95860476928751,
14.2633307880091));
#51596=CARTESIAN_POINT('Ctrl Pts',(0.553159917363878,-1.98017772645335,
14.2594713852901));
#51597=CARTESIAN_POINT('Ctrl Pts',(0.484047713484457,-1.99819258583566,
14.255611982571));
#51598=CARTESIAN_POINT('Ctrl Pts',(0.4142492004212,-2.01255935625521,14.251752579852));
#51599=CARTESIAN_POINT('Ctrl Pts',(0.344411166890853,-2.02693426125318,
14.2478909919087));
#51600=CARTESIAN_POINT('Ctrl Pts',(0.273886531097746,-2.03765689230798,
14.2440294039655));
#51601=CARTESIAN_POINT('Ctrl Pts',(0.203088009751233,-2.04468893056995,
14.2401678160223));
#51602=CARTESIAN_POINT('Ctrl Pts',(0.132165623852401,-2.05173327163507,
14.2362994720925));
#51603=CARTESIAN_POINT('Ctrl Pts',(0.0609688811211802,-2.05507410589783,
14.2324311281626));
#51604=CARTESIAN_POINT('Ctrl Pts',(-0.0100881451754699,-2.05472523511707,
14.2285627842328));
#51605=CARTESIAN_POINT('Ctrl Pts',(-0.0522797632143424,-2.05451808568381,
14.2262658728922));
#51606=CARTESIAN_POINT('Ctrl Pts',(-0.0944221736534997,-2.05301107601554,
14.2239689615516));
#51607=CARTESIAN_POINT('Ctrl Pts',(-0.136429893586073,-2.05021570734303,
14.221672050211));
#51608=CARTESIAN_POINT('Ctrl Pts',(-0.207190721651772,-2.04550698708082,
14.2178029673682));
#51609=CARTESIAN_POINT('Ctrl Pts',(-0.277846082889716,-2.03712140126886,
14.2139338845255));
#51610=CARTESIAN_POINT('Ctrl Pts',(-0.34798331061511,-2.02506917857967,
14.2100648016827));
#51611=CARTESIAN_POINT('Ctrl Pts',(-0.418016037367383,-2.01303491310152,
14.2062014835805));
#51612=CARTESIAN_POINT('Ctrl Pts',(-0.487531688126347,-1.99734493646067,
14.2023381654784));
#51613=CARTESIAN_POINT('Ctrl Pts',(-0.556121216616893,-1.97806136278138,
14.1984748473762));
#51614=CARTESIAN_POINT('Ctrl Pts',(-0.62463028961483,-1.95880040872719,
14.1946160609447));
#51615=CARTESIAN_POINT('Ctrl Pts',(-0.692214932802764,-1.93595436146375,
14.1907572745133));
#51616=CARTESIAN_POINT('Ctrl Pts',(-0.75847654541342,-1.90963632468534,
14.1868984880819));
#51617=CARTESIAN_POINT('Ctrl Pts',(-0.82469641806565,-1.88333486634077,
14.1830421324031));
#51618=CARTESIAN_POINT('Ctrl Pts',(-0.889594463209346,-1.85356593654599,
14.1791857767242));
#51619=CARTESIAN_POINT('Ctrl Pts',(-0.952788906082997,-1.82049192883274,
14.1753294210453));
#51620=CARTESIAN_POINT('Ctrl Pts',(-1.01596468068449,-1.78742769151305,
14.1714742045726));
#51621=CARTESIAN_POINT('Ctrl Pts',(-1.07743742196365,-1.7510605397422,14.1676189880999));
#51622=CARTESIAN_POINT('Ctrl Pts',(-1.13684852569153,-1.71159954198784,
14.1637637716272));
#51623=CARTESIAN_POINT('Ctrl Pts',(-1.19626195221509,-1.67213700142701,
14.1599084044271));
#51624=CARTESIAN_POINT('Ctrl Pts',(-1.25361317772226,-1.62958064534053,
14.156053037227));
#51625=CARTESIAN_POINT('Ctrl Pts',(-1.30857270230379,-1.5841827689018,14.1521976700269));
#51626=CARTESIAN_POINT('Ctrl Pts',(-1.36358975452008,-1.53873737326644,
14.1483382673087));
#51627=CARTESIAN_POINT('Ctrl Pts',(-1.41620973304714,-1.49044482992165,
14.1444788645905));
#51628=CARTESIAN_POINT('Ctrl Pts',(-1.46613707196258,-1.43959704386921,
14.1406194618724));
#51629=CARTESIAN_POINT('Ctrl Pts',(-1.51609268012903,-1.38872046740139,
14.1367578739301));
#51630=CARTESIAN_POINT('Ctrl Pts',(-1.56335229170375,-1.33528613214971,
14.1328962859878));
#51631=CARTESIAN_POINT('Ctrl Pts',(-1.60765986433228,-1.27961999168312,
14.1290346980455));
#51632=CARTESIAN_POINT('Ctrl Pts',(-1.6520449546473,-1.22385646130848,14.1251663541167));
#51633=CARTESIAN_POINT('Ctrl Pts',(-1.69346741214216,-1.16585372547734,
14.1212980101879));
#51634=CARTESIAN_POINT('Ctrl Pts',(-1.73171424693945,-1.10596714663996,
14.117429666259));
#51635=CARTESIAN_POINT('Ctrl Pts',(-1.75442411721769,-1.07040821884861,
14.1151327549125));
#51636=CARTESIAN_POINT('Ctrl Pts',(-1.7760152426764,-1.03418561337468,14.112835843566));
#51637=CARTESIAN_POINT('Ctrl Pts',(-1.79645092163318,-0.997377385277664,
14.1105389322194));
#51638=CARTESIAN_POINT('Ctrl Pts',(-1.8325132064301,-0.932422909954774,
14.1064856354679));
#51639=CARTESIAN_POINT('Ctrl Pts',(-1.86510495352398,-0.86540946720002,
14.1024323387163));
#51640=CARTESIAN_POINT('Ctrl Pts',(-1.89399792216641,-0.796724188994735,
14.0983790419647));
#51641=CARTESIAN_POINT('Ctrl Pts',(-1.92280997820391,-0.728231258791105,
14.0943370961685));
#51642=CARTESIAN_POINT('Ctrl Pts',(-1.94794371962189,-0.658076199843631,
14.0902951503723));
#51643=CARTESIAN_POINT('Ctrl Pts',(-1.96921717900164,-0.586669638233323,
14.0862532045761));
#51644=CARTESIAN_POINT('Ctrl Pts',(-1.99045484462435,-0.51538322206207,
14.0822180595745));
#51645=CARTESIAN_POINT('Ctrl Pts',(-2.00784502257861,-0.44284988883517,
14.0781829145728));
#51646=CARTESIAN_POINT('Ctrl Pts',(-2.02125400722186,-0.369499392136954,
14.0741477695712));
#51647=CARTESIAN_POINT('Ctrl Pts',(-2.03463537803434,-0.296299949993299,
14.0701209343569));
#51648=CARTESIAN_POINT('Ctrl Pts',(-2.04405180395157,-0.222287105409238,
14.0660940991425));
#51649=CARTESIAN_POINT('Ctrl Pts',(-2.04941996305247,-0.147903270896886,
14.0620672639282));
#51650=CARTESIAN_POINT('Ctrl Pts',(-2.05297157352164,-0.0986904214962947,
14.0594030824396));
#51651=CARTESIAN_POINT('Ctrl Pts',(-2.05475218685897,-0.0493154866282622,
14.0567389009509));
#51652=CARTESIAN_POINT('Ctrl Pts',(-2.05474999798348,9.10323576868401E-5,
14.0540747194623));
#51653=CARTESIAN_POINT('Origin',(0.,0.,18.5459252805377));
#51654=CARTESIAN_POINT('',(1.25206542099588,1.62921138715835,15.2060150049977));
#51655=CARTESIAN_POINT('',(1.25109478256769,1.6279226134271,15.1480161847457));
#51656=CARTESIAN_POINT('',(1.25206542099588,1.62921138715835,18.5459252805377));
#51657=CARTESIAN_POINT('',(-2.05474914219178,0.00187754151781767,14.6959252704371));
#51658=CARTESIAN_POINT('Ctrl Pts',(1.25109478256748,1.62792261342726,15.1480161847458));
#51659=CARTESIAN_POINT('Ctrl Pts',(1.42360946980995,1.49766989531232,15.1363160149331));
#51660=CARTESIAN_POINT('Ctrl Pts',(2.05683536821899,0.846821926034871,15.0875714724566));
#51661=CARTESIAN_POINT('Ctrl Pts',(2.24042116521983,-0.937279091896088,
15.0017825573163));
#51662=CARTESIAN_POINT('Ctrl Pts',(0.427721193935683,-2.39061364822391,
14.8906494393247));
#51663=CARTESIAN_POINT('Ctrl Pts',(-1.59436008174594,-1.71665379493215,
14.7886970137319));
#51664=CARTESIAN_POINT('Ctrl Pts',(-2.04978635669156,-0.51206744035561,
14.7237889608028));
#51665=CARTESIAN_POINT('Ctrl Pts',(-2.05444347718377,0.00187707591058038,
14.6959252805377));
#51666=CARTESIAN_POINT('Ctrl Pts',(-2.05474914219178,0.00187754151781767,
14.6959252704371));
#51667=CARTESIAN_POINT('Ctrl Pts',(-2.05466440026703,0.0946176463469028,
14.6908980355964));
#51668=CARTESIAN_POINT('Ctrl Pts',(-2.04829723603806,0.187078217758331,
14.6858708007558));
#51669=CARTESIAN_POINT('Ctrl Pts',(-2.03578285247768,0.278542169263164,
14.6808435659151));
#51670=CARTESIAN_POINT('Ctrl Pts',(-2.02544358636103,0.354108826632005,
14.6766901117239));
#51671=CARTESIAN_POINT('Ctrl Pts',(-2.01090920585382,0.428995861661035,
14.6725366575328));
#51672=CARTESIAN_POINT('Ctrl Pts',(-1.99227978030212,0.502810938126188,
14.6683832033416));
#51673=CARTESIAN_POINT('Ctrl Pts',(-1.9749258411557,0.571572175100983,14.6645141204716));
#51674=CARTESIAN_POINT('Ctrl Pts',(-1.95397391117961,0.639568607569909,
14.6606450376015));
#51675=CARTESIAN_POINT('Ctrl Pts',(-1.9295082448856,0.70639613208063,14.6567759547315));
#51676=CARTESIAN_POINT('Ctrl Pts',(-1.90507903121191,0.773124086918992,
14.6529126366016));
#51677=CARTESIAN_POINT('Ctrl Pts',(-1.8771466387746,0.838686138398381,14.6490493184717));
#51678=CARTESIAN_POINT('Ctrl Pts',(-1.84584571117744,0.902691072863716,
14.6451860003418));
#51679=CARTESIAN_POINT('Ctrl Pts',(-1.81458149955306,0.9666209295722,14.6413272138822));
#51680=CARTESIAN_POINT('Ctrl Pts',(-1.77995681374694,1.02899686303295,14.6374684274226));
#51681=CARTESIAN_POINT('Ctrl Pts',(-1.74215457810066,1.08944710220501,14.633609640963));
#51682=CARTESIAN_POINT('Ctrl Pts',(-1.70437615508864,1.14985926216268,14.6297532852556));
#51683=CARTESIAN_POINT('Ctrl Pts',(-1.66342441038333,1.20834772359031,14.6258969295483));
#51684=CARTESIAN_POINT('Ctrl Pts',(-1.61952772989123,1.26456612899972,14.622040573841));
#51685=CARTESIAN_POINT('Ctrl Pts',(-1.57564401691594,1.32076792693203,14.6181853573395));
#51686=CARTESIAN_POINT('Ctrl Pts',(-1.52881739407797,1.37470061748818,14.6143301408381));
#51687=CARTESIAN_POINT('Ctrl Pts',(-1.47931799588639,1.42604902774999,14.6104749243367));
#51688=CARTESIAN_POINT('Ctrl Pts',(-1.4298166624145,1.47739944558301,14.6066195571077));
#51689=CARTESIAN_POINT('Ctrl Pts',(-1.37764268485453,1.52616503431371,14.6027641898787));
#51690=CARTESIAN_POINT('Ctrl Pts',(-1.32310348745199,1.57206702274183,14.5989088226497));
#51691=CARTESIAN_POINT('Ctrl Pts',(-1.26850720238146,1.61801705803534,14.5950494199025));
#51692=CARTESIAN_POINT('Ctrl Pts',(-1.21154112776492,1.66109719607844,14.5911900171552));
#51693=CARTESIAN_POINT('Ctrl Pts',(-1.15254555132663,1.70106916808729,14.587330614408));
#51694=CARTESIAN_POINT('Ctrl Pts',(-1.09351657112867,1.74106377254127,14.5834690264366));
#51695=CARTESIAN_POINT('Ctrl Pts',(-1.03245621757575,1.77794645632113,14.5796074384652));
#51696=CARTESIAN_POINT('Ctrl Pts',(-0.969731166288907,1.81152395171247,
14.5757458504937));
#51697=CARTESIAN_POINT('Ctrl Pts',(-0.906896375279786,1.8451601921338,14.5718775065359));
#51698=CARTESIAN_POINT('Ctrl Pts',(-0.842391511530458,1.87547949244146,
14.5680091625781));
#51699=CARTESIAN_POINT('Ctrl Pts',(-0.776604440019373,1.90233622323768,
14.5641408186203));
#51700=CARTESIAN_POINT('Ctrl Pts',(-0.737541974068368,1.91828297551264,
14.5618439075302));
#51701=CARTESIAN_POINT('Ctrl Pts',(-0.698027781771188,1.93300989149292,
14.5595469964402));
#51702=CARTESIAN_POINT('Ctrl Pts',(-0.658145244802309,1.9464949009037,14.5572500853501));
#51703=CARTESIAN_POINT('Ctrl Pts',(-0.590963485530717,1.9692102727146,14.5533809601727));
#51704=CARTESIAN_POINT('Ctrl Pts',(-0.522472755723196,1.98848796324828,
14.5495118349954));
#51705=CARTESIAN_POINT('Ctrl Pts',(-0.453058266798325,2.00417957513435,
14.545642709818));
#51706=CARTESIAN_POINT('Ctrl Pts',(-0.383747422431103,2.01984775747137,
14.541779361731));
#51707=CARTESIAN_POINT('Ctrl Pts',(-0.313516026828389,2.0319403835457,14.5379160136439));
#51708=CARTESIAN_POINT('Ctrl Pts',(-0.242765789127639,2.04035838374763,
14.5340526655568));
#51709=CARTESIAN_POINT('Ctrl Pts',(-0.172099404093816,2.04876640699697,
14.5301938962817));
#51710=CARTESIAN_POINT('Ctrl Pts',(-0.100915878549273,2.05350839865137,
14.5263351270067));
#51711=CARTESIAN_POINT('Ctrl Pts',(-0.0296267588397955,2.05453639969231,
14.5224763577316));
#51712=CARTESIAN_POINT('Ctrl Pts',(0.0416171306537917,2.05556374850597,
14.5186200366979));
#51713=CARTESIAN_POINT('Ctrl Pts',(0.112965996818219,2.0528817750382,14.5147637156641));
#51714=CARTESIAN_POINT('Ctrl Pts',(0.184004992428342,2.04649449675816,14.5109073946304));
#51715=CARTESIAN_POINT('Ctrl Pts',(0.255022680246738,2.04010913431033,14.5070522302809));
#51716=CARTESIAN_POINT('Ctrl Pts',(0.325730198514623,2.0300207172167,14.5031970659314));
#51717=CARTESIAN_POINT('Ctrl Pts',(0.395716261069186,2.01628524847687,14.4993419015818));
#51718=CARTESIAN_POINT('Ctrl Pts',(0.465704742375029,2.00254930503276,14.495486603996));
#51719=CARTESIAN_POINT('Ctrl Pts',(0.534971242295313,1.9851661556892,14.4916313064102));
#51720=CARTESIAN_POINT('Ctrl Pts',(0.603114836539192,1.96424287104378,14.4877760088244));
#51721=CARTESIAN_POINT('Ctrl Pts',(0.671326171198658,1.9432987869085,14.4839168787513));
#51722=CARTESIAN_POINT('Ctrl Pts',(0.738411907158264,1.91880768673003,14.4800577486781));
#51723=CARTESIAN_POINT('Ctrl Pts',(0.803987381797254,1.89092618904356,14.476198618605));
#51724=CARTESIAN_POINT('Ctrl Pts',(0.869599866550078,1.86302895533064,14.4723373104791));
#51725=CARTESIAN_POINT('Ctrl Pts',(0.933699956603814,1.83173772811405,14.4684760023532));
#51726=CARTESIAN_POINT('Ctrl Pts',(0.995926478592241,1.79725568902671,14.4646146942273));
#51727=CARTESIAN_POINT('Ctrl Pts',(1.05825441429214,1.76271745281551,14.4607470931322));
#51728=CARTESIAN_POINT('Ctrl Pts',(1.11870227588255,1.72497828292203,14.4568794920371));
#51729=CARTESIAN_POINT('Ctrl Pts',(1.17693752772968,1.68428489820503,14.4530118909419));
#51730=CARTESIAN_POINT('Ctrl Pts',(1.20241169009358,1.66648417001142,14.4513200651984));
#51731=CARTESIAN_POINT('Ctrl Pts',(1.22746289710024,1.64811867548308,14.4496282394549));
#51732=CARTESIAN_POINT('Ctrl Pts',(1.25206542099587,1.62921138715835,14.4479364137114));
#51733=CARTESIAN_POINT('',(-2.0547491753793,-0.00184086341081391,14.7540747194092));
#51734=CARTESIAN_POINT('Ctrl Pts',(-2.0547491753793,-0.00184086341080706,
14.7540747194092));
#51735=CARTESIAN_POINT('Ctrl Pts',(-2.05481200415796,0.068287849233049,
14.7502679504067));
#51736=CARTESIAN_POINT('Ctrl Pts',(-2.05128035637574,0.138528733663465,
14.7464611814043));
#51737=CARTESIAN_POINT('Ctrl Pts',(-2.04414642809902,0.208477679836533,
14.7426544124019));
#51738=CARTESIAN_POINT('Ctrl Pts',(-2.03701831865898,0.278369571680172,
14.7388507484163));
#51739=CARTESIAN_POINT('Ctrl Pts',(-2.02629380219727,0.347969501103903,
14.7350470844307));
#51740=CARTESIAN_POINT('Ctrl Pts',(-2.01201710821451,0.416874943780628,
14.7312434204451));
#51741=CARTESIAN_POINT('Ctrl Pts',(-1.99774696631999,0.485748763272034,
14.7274415020976));
#51742=CARTESIAN_POINT('Ctrl Pts',(-1.97992798093516,0.553928238327332,
14.7236395837502));
#51743=CARTESIAN_POINT('Ctrl Pts',(-1.95865575939417,0.621019467240785,
14.7198376654028));
#51744=CARTESIAN_POINT('Ctrl Pts',(-1.93738571327467,0.688103835013735,
14.7160361358617));
#51745=CARTESIAN_POINT('Ctrl Pts',(-1.91266328488549,0.754099700744834,
14.7122346063206));
#51746=CARTESIAN_POINT('Ctrl Pts',(-1.88463382974959,0.818628664452574,
14.7084330767795));
#51747=CARTESIAN_POINT('Ctrl Pts',(-1.8565783874181,0.883217455466713,14.7046280226928));
#51748=CARTESIAN_POINT('Ctrl Pts',(-1.82520999617619,0.946336168563494,
14.7008229686062));
#51749=CARTESIAN_POINT('Ctrl Pts',(-1.79072159216291,1.00762777942131,14.6970179145196));
#51750=CARTESIAN_POINT('Ctrl Pts',(-1.75621664581928,1.06894878874228,14.6932110353423));
#51751=CARTESIAN_POINT('Ctrl Pts',(-1.71858897733662,1.1284405288387,14.6894041561651));
#51752=CARTESIAN_POINT('Ctrl Pts',(-1.67807525655495,1.18577442873341,14.6855972769878));
#51753=CARTESIAN_POINT('Ctrl Pts',(-1.63749044941838,1.24320892807632,14.6817837181683));
#51754=CARTESIAN_POINT('Ctrl Pts',(-1.59400979112279,1.29847763551897,14.6779701593487));
#51755=CARTESIAN_POINT('Ctrl Pts',(-1.54791012952976,1.35128523761608,14.6741566005291));
#51756=CARTESIAN_POINT('Ctrl Pts',(-1.51586760806649,1.38799025160423,14.6715059077452));
#51757=CARTESIAN_POINT('Ctrl Pts',(-1.48256060688962,1.42350698204244,14.6688552149612));
#51758=CARTESIAN_POINT('Ctrl Pts',(-1.44809173787727,1.45774753684977,14.6662045221772));
#51759=CARTESIAN_POINT('Ctrl Pts',(-1.39777926479025,1.50772675118406,14.6623354393446));
#51760=CARTESIAN_POINT('Ctrl Pts',(-1.34477774896543,1.55519608254071,14.658466356512));
#51761=CARTESIAN_POINT('Ctrl Pts',(-1.28936767615483,1.59985266765008,14.6545972736794));
#51762=CARTESIAN_POINT('Ctrl Pts',(-1.23404016158673,1.64444271667683,14.6507339555871));
#51763=CARTESIAN_POINT('Ctrl Pts',(-1.1763115885187,1.68622803583219,14.6468706374948));
#51764=CARTESIAN_POINT('Ctrl Pts',(-1.11649897912541,1.72494277937325,14.6430073194025));
#51765=CARTESIAN_POINT('Ctrl Pts',(-1.0567565298946,1.76361211053848,14.6391485329805));
#51766=CARTESIAN_POINT('Ctrl Pts',(-0.994935305920528,1.79921775777028,
14.6352897465584));
#51767=CARTESIAN_POINT('Ctrl Pts',(-0.931383681591147,1.83153542148814,
14.6314309601364));
#51768=CARTESIAN_POINT('Ctrl Pts',(-0.867872090121343,1.86383272744949,
14.6275746044666));
#51769=CARTESIAN_POINT('Ctrl Pts',(-0.802632692876482,1.89284593942531,
14.6237182487969));
#51770=CARTESIAN_POINT('Ctrl Pts',(-0.736039723038107,1.91839596762764,
14.6198618931271));
#51771=CARTESIAN_POINT('Ctrl Pts',(-0.669466425425528,1.94393844809745,
14.6160066766632));
#51772=CARTESIAN_POINT('Ctrl Pts',(-0.601540802349471,1.96601960193036,
14.6121514601993));
#51773=CARTESIAN_POINT('Ctrl Pts',(-0.532656789490892,1.98450858075979,
14.6082962437353));
#51774=CARTESIAN_POINT('Ctrl Pts',(-0.463770083468561,2.00299828245431,
14.6044408765437));
#51775=CARTESIAN_POINT('Ctrl Pts',(-0.39392538301915,2.01789540651023,14.6005855093521));
#51776=CARTESIAN_POINT('Ctrl Pts',(-0.323529816316513,2.02911951852379,
14.5967301421604));
#51777=CARTESIAN_POINT('Ctrl Pts',(-0.253060564641824,2.04035537912349,
14.5928707394501));
#51778=CARTESIAN_POINT('Ctrl Pts',(-0.182039776383841,2.0479104762673,14.5890113367398));
#51779=CARTESIAN_POINT('Ctrl Pts',(-0.110881865592379,2.05175602213878,
14.5851519340295));
#51780=CARTESIAN_POINT('Ctrl Pts',(-0.0396836646277538,2.05560374538881,
14.5812903460948));
#51781=CARTESIAN_POINT('Ctrl Pts',(0.0316513274151431,2.05573773525014,
14.5774287581601));
#51782=CARTESIAN_POINT('Ctrl Pts',(0.102709278480053,2.05218136786545,14.5735671702254));
#51783=CARTESIAN_POINT('Ctrl Pts',(0.173891547988154,2.048618778488,14.5696988263036));
#51784=CARTESIAN_POINT('Ctrl Pts',(0.244795325409388,2.04135299099028,14.5658304823818));
#51785=CARTESIAN_POINT('Ctrl Pts',(0.315013174792762,2.03045912596314,14.5619621384599));
#51786=CARTESIAN_POINT('Ctrl Pts',(0.356706515335843,2.02399066205552,14.5596652270352));
#51787=CARTESIAN_POINT('Ctrl Pts',(0.398158221144476,2.01624404678126,14.5573683156105));
#51788=CARTESIAN_POINT('Ctrl Pts',(0.439285463970684,2.00724334440149,14.5550714041857));
#51789=CARTESIAN_POINT('Ctrl Pts',(0.508568827310319,1.99208067142763,14.5512020042974));
#51790=CARTESIAN_POINT('Ctrl Pts',(0.577201932179294,1.97329693947935,14.547332604409));
#51791=CARTESIAN_POINT('Ctrl Pts',(0.644778103482944,1.95096354649925,14.5434632045207));
#51792=CARTESIAN_POINT('Ctrl Pts',(0.712237378025983,1.92866878697889,14.5396004981206));
#51793=CARTESIAN_POINT('Ctrl Pts',(0.778642894299039,1.90283671819843,14.5357377917206));
#51794=CARTESIAN_POINT('Ctrl Pts',(0.84359954762269,1.8735894336142,14.5318750853206));
#51795=CARTESIAN_POINT('Ctrl Pts',(0.90849154592418,1.84437126050257,14.5280162236902));
#51796=CARTESIAN_POINT('Ctrl Pts',(0.971937101666074,1.81174481386403,14.5241573620598));
#51797=CARTESIAN_POINT('Ctrl Pts',(1.0335587985445,1.77588112565319,14.5202985004294));
#51798=CARTESIAN_POINT('Ctrl Pts',(1.09513639691661,1.74004310267329,14.5164424003268));
#51799=CARTESIAN_POINT('Ctrl Pts',(1.15489230980045,1.70097268283746,14.5125863002243));
#51800=CARTESIAN_POINT('Ctrl Pts',(1.2124731690813,1.65888708981593,14.5087302001218));
#51801=CARTESIAN_POINT('Ctrl Pts',(1.22578816197413,1.64915522094542,14.5078385158694));
#51802=CARTESIAN_POINT('Ctrl Pts',(1.23898696426032,1.63926231337188,14.506946831617));
#51803=CARTESIAN_POINT('Ctrl Pts',(1.25206542099588,1.62921138715834,14.5060551473646));
#51804=CARTESIAN_POINT('Ctrl Pts',(1.25206542099588,1.62921138715835,15.2060150049977));
#51805=CARTESIAN_POINT('Ctrl Pts',(1.31002493594645,1.5846689139966,15.2020450878788));
#51806=CARTESIAN_POINT('Ctrl Pts',(1.3656874068559,1.53696607619391,15.1980751707598));
#51807=CARTESIAN_POINT('Ctrl Pts',(1.41869350001138,1.48637354508396,15.1941052536409));
#51808=CARTESIAN_POINT('Ctrl Pts',(1.47020089051233,1.43721147519384,15.190247582586));
#51809=CARTESIAN_POINT('Ctrl Pts',(1.51919974906799,1.38532131376408,15.1863899115311));
#51810=CARTESIAN_POINT('Ctrl Pts',(1.56539333322814,1.33099259005634,15.1825322404761));
#51811=CARTESIAN_POINT('Ctrl Pts',(1.61156391415845,1.276690920671,15.1786764904433));
#51812=CARTESIAN_POINT('Ctrl Pts',(1.6549316785281,1.21995346821481,15.1748207404104));
#51813=CARTESIAN_POINT('Ctrl Pts',(1.69523825658542,1.16110499779703,15.1709649903775));
#51814=CARTESIAN_POINT('Ctrl Pts',(1.73553824609788,1.10226614679635,15.1671098706086));
#51815=CARTESIAN_POINT('Ctrl Pts',(1.77277776903087,1.04131736415472,15.1632547508396));
#51816=CARTESIAN_POINT('Ctrl Pts',(1.80674114035724,0.978613311906503,15.1593996310707));
#51817=CARTESIAN_POINT('Ctrl Pts',(1.84246738032578,0.912654606096864,15.1553444113267));
#51818=CARTESIAN_POINT('Ctrl Pts',(1.8745678293376,0.844753972659132,15.1512891915828));
#51819=CARTESIAN_POINT('Ctrl Pts',(1.90284681176006,0.775352547861011,15.1472339718389));
#51820=CARTESIAN_POINT('Ctrl Pts',(1.92976604909418,0.709288168402204,15.1433737401976));
#51821=CARTESIAN_POINT('Ctrl Pts',(1.95322274739721,0.641864500279134,15.1395135085564));
#51822=CARTESIAN_POINT('Ctrl Pts',(1.97309880704926,0.573479433040795,15.1356532769152));
#51823=CARTESIAN_POINT('Ctrl Pts',(1.99298878077377,0.50504649339728,15.1317903429505));
#51824=CARTESIAN_POINT('Ctrl Pts',(2.00929301886529,0.435651288130338,15.1279274089858));
#51825=CARTESIAN_POINT('Ctrl Pts',(2.02194445546334,0.365702312709494,15.1240644750211));
#51826=CARTESIAN_POINT('Ctrl Pts',(2.03461637026184,0.295640114641596,15.1201952883328));
#51827=CARTESIAN_POINT('Ctrl Pts',(2.0436236323153,0.225022839254271,15.1163261016445));
#51828=CARTESIAN_POINT('Ctrl Pts',(2.04895103336775,0.154263493287422,15.1124569149562));
#51829=CARTESIAN_POINT('Ctrl Pts',(2.0497404075253,0.143778906420101,15.1118836080186));
#51830=CARTESIAN_POINT('Ctrl Pts',(2.05044908328428,0.13329119718587,15.1113103010811));
#51831=CARTESIAN_POINT('Ctrl Pts',(2.0510771082687,0.122801703718274,15.1107369941435));
#51832=CARTESIAN_POINT('Ctrl Pts',(2.05531546848585,0.0520111254545155,
15.1068679103067));
#51833=CARTESIAN_POINT('Ctrl Pts',(2.05589294399514,-0.0191377846633052,
15.1029988264699));
#51834=CARTESIAN_POINT('Ctrl Pts',(2.05276772273151,-0.0902343560496397,
15.0991297426331));
#51835=CARTESIAN_POINT('Ctrl Pts',(2.04964715788051,-0.161224997344817,
15.0952664235244));
#51836=CARTESIAN_POINT('Ctrl Pts',(2.04283486815184,-0.232162973339852,
15.0914031044157));
#51837=CARTESIAN_POINT('Ctrl Pts',(2.0323409698537,-0.302634672095116,15.087539785307));
#51838=CARTESIAN_POINT('Ctrl Pts',(2.02185938085436,-0.373023707842593,
15.0836809978554));
#51839=CARTESIAN_POINT('Ctrl Pts',(2.0077048325131,-0.442947074607792,15.0798222104038));
#51840=CARTESIAN_POINT('Ctrl Pts',(1.989939340115,-0.511995102674516,15.0759634229523));
#51841=CARTESIAN_POINT('Ctrl Pts',(1.97218503863566,-0.58099963569729,15.0721070662455));
#51842=CARTESIAN_POINT('Ctrl Pts',(1.95082442667367,-0.649129454636971,
15.0682507095386));
#51843=CARTESIAN_POINT('Ctrl Pts',(1.92597053566178,-0.715985375732399,
15.0643943528318));
#51844=CARTESIAN_POINT('Ctrl Pts',(1.90112398669591,-0.782821547032968,
15.0605391353248));
#51845=CARTESIAN_POINT('Ctrl Pts',(1.87278637655547,-0.848384112500162,
15.0566839178178));
#51846=CARTESIAN_POINT('Ctrl Pts',(1.8411199575779,-0.912290997603469,15.0528287003108));
#51847=CARTESIAN_POINT('Ctrl Pts',(1.80945230049949,-0.9762003813527,15.0489733320716));
#51848=CARTESIAN_POINT('Ctrl Pts',(1.77445579384431,-1.03845352191843,15.0451179638324));
#51849=CARTESIAN_POINT('Ctrl Pts',(1.73633923719926,-1.09869177473134,15.0412625955933));
#51850=CARTESIAN_POINT('Ctrl Pts',(1.69818278292289,-1.15899308055358,15.0374031918358));
#51851=CARTESIAN_POINT('Ctrl Pts',(1.65690001959088,-1.21727487716614,15.0335437880784));
#51852=CARTESIAN_POINT('Ctrl Pts',(1.61274331405848,-1.27320719659436,15.0296843843209));
#51853=CARTESIAN_POINT('Ctrl Pts',(1.56856160664066,-1.32917118535626,15.0258227953377));
#51854=CARTESIAN_POINT('Ctrl Pts',(1.52150303828498,-1.38278268347052,15.0219612063545));
#51855=CARTESIAN_POINT('Ctrl Pts',(1.47185872990816,-1.43374664487598,15.0180996173713));
#51856=CARTESIAN_POINT('Ctrl Pts',(1.42212756716924,-1.48479976942024,15.0142312724103));
#51857=CARTESIAN_POINT('Ctrl Pts',(1.36980198918227,-1.5331957794779,15.0103629274492));
#51858=CARTESIAN_POINT('Ctrl Pts',(1.31520771249558,-1.57867863591427,15.0064945824881));
#51859=CARTESIAN_POINT('Ctrl Pts',(1.28279134045791,-1.60568493190458,15.0041976803761));
#51860=CARTESIAN_POINT('Ctrl Pts',(1.24957571633715,-1.63166495949266,15.001900778264));
#51861=CARTESIAN_POINT('Ctrl Pts',(1.21563365191156,-1.65657248161382,14.999603876152));
#51862=CARTESIAN_POINT('Ctrl Pts',(1.15845896507748,-1.69852867376624,14.9957347933143));
#51863=CARTESIAN_POINT('Ctrl Pts',(1.09899764070911,-1.73760358972471,14.9918657104766));
#51864=CARTESIAN_POINT('Ctrl Pts',(1.03757201844991,-1.77353936213149,14.9879966276389));
#51865=CARTESIAN_POINT('Ctrl Pts',(0.976237917260044,-1.80942159205556,
14.9841333095388));
#51866=CARTESIAN_POINT('Ctrl Pts',(0.912945743490394,-1.84217371916727,
14.9802699914388));
#51867=CARTESIAN_POINT('Ctrl Pts',(0.848048472860544,-1.87157990750566,
14.9764066733388));
#51868=CARTESIAN_POINT('Ctrl Pts',(0.783227326633131,-1.90095160242864,
14.9725478869052));
#51869=CARTESIAN_POINT('Ctrl Pts',(0.71680526370732,-1.92698495500048,14.9686891004716));
#51870=CARTESIAN_POINT('Ctrl Pts',(0.649160096811672,-1.94950986948193,
14.9648303140379));
#51871=CARTESIAN_POINT('Ctrl Pts',(0.581557541365009,-1.97202059493424,
14.9609739583542));
#51872=CARTESIAN_POINT('Ctrl Pts',(0.512733870351755,-1.99102711390201,
14.9571176026705));
#51873=CARTESIAN_POINT('Ctrl Pts',(0.443085757073116,-2.00640787836844,
14.9532612469867));
#51874=CARTESIAN_POINT('Ctrl Pts',(0.373458218497088,-2.02178409921352,
14.9494060305065));
#51875=CARTESIAN_POINT('Ctrl Pts',(0.303007195261644,-2.03353658725471,
14.9455508140262));
#51876=CARTESIAN_POINT('Ctrl Pts',(0.232141683100166,-2.04159442629221,
14.9416955975459));
#51877=CARTESIAN_POINT('Ctrl Pts',(0.161273400260681,-2.04965258037263,
14.9378402303356));
#51878=CARTESIAN_POINT('Ctrl Pts',(0.0899910792428621,-2.05401574596433,
14.9339848631252));
#51879=CARTESIAN_POINT('Ctrl Pts',(0.0187092778158862,-2.05466482070035,
14.9301294959149));
#51880=CARTESIAN_POINT('Ctrl Pts',(-0.0526471362938743,-2.05531457484131,
14.9262700931823));
#51881=CARTESIAN_POINT('Ctrl Pts',(-0.124002542968951,-2.05224247308525,
14.9224106904498));
#51882=CARTESIAN_POINT('Ctrl Pts',(-0.194942846560374,-2.0454815689893,
14.9185512877173));
#51883=CARTESIAN_POINT('Ctrl Pts',(-0.265923317150839,-2.03871683681235,
14.9146896997583));
#51884=CARTESIAN_POINT('Ctrl Pts',(-0.336487736013471,-2.02825921572408,
14.9108281117994));
#51885=CARTESIAN_POINT('Ctrl Pts',(-0.406230327112479,-2.01419325880961,
14.9069665238404));
#51886=CARTESIAN_POINT('Ctrl Pts',(-0.476094935437547,-2.00010269298662,
14.9030981798914));
#51887=CARTESIAN_POINT('Ctrl Pts',(-0.545134374660318,-1.98239130817406,
14.8992298359424));
#51888=CARTESIAN_POINT('Ctrl Pts',(-0.612956875764157,-1.96119387898123,
14.8953614919934));
#51889=CARTESIAN_POINT('Ctrl Pts',(-0.653227924491973,-1.94860745574358,
14.8930645807158));
#51890=CARTESIAN_POINT('Ctrl Pts',(-0.693070266519139,-1.93479291673721,
14.8907676694381));
#51891=CARTESIAN_POINT('Ctrl Pts',(-0.73240556392774,-1.91978635593331,
14.8884707581604));
#51892=CARTESIAN_POINT('Ctrl Pts',(-0.798664768406605,-1.89450822544146,
14.8846016755795));
#51893=CARTESIAN_POINT('Ctrl Pts',(-0.863743545098733,-1.86574626808071,
14.8807325929986));
#51894=CARTESIAN_POINT('Ctrl Pts',(-0.927250420455131,-1.83363142977693,
14.8768635104177));
#51895=CARTESIAN_POINT('Ctrl Pts',(-0.990662673646188,-1.80156444102523,
14.8730001925823));
#51896=CARTESIAN_POINT('Ctrl Pts',(-1.05250724444457,-1.76615470495226,
14.8691368747469));
#51897=CARTESIAN_POINT('Ctrl Pts',(-1.11241135485258,-1.72758170287111,
14.8652735569115));
#51898=CARTESIAN_POINT('Ctrl Pts',(-1.17224519766254,-1.68905394697068,
14.8614147707528));
#51899=CARTESIAN_POINT('Ctrl Pts',(-1.23014269485957,-1.64737055712081,
14.8575559845942));
#51900=CARTESIAN_POINT('Ctrl Pts',(-1.28575602520601,-1.60275668962773,
14.8536971984355));
#51901=CARTESIAN_POINT('Ctrl Pts',(-1.34133432317754,-1.55817092564368,
14.8498408430329));
#51902=CARTESIAN_POINT('Ctrl Pts',(-1.39463093094656,-1.5106586496889,14.8459844876304));
#51903=CARTESIAN_POINT('Ctrl Pts',(-1.44532858421168,-1.46048719479517,
14.8421281322279));
#51904=CARTESIAN_POINT('Ctrl Pts',(-1.4960112608391,-1.41033056109442,14.8382729160346));
#51905=CARTESIAN_POINT('Ctrl Pts',(-1.54409616207844,-1.35751664950813,
14.8344176998414));
#51906=CARTESIAN_POINT('Ctrl Pts',(-1.58930187764166,-1.30235060725778,
14.8305624836481));
#51907=CARTESIAN_POINT('Ctrl Pts',(-1.63450936058051,-1.24718240821999,
14.8267071167302));
#51908=CARTESIAN_POINT('Ctrl Pts',(-1.67683712816198,-1.18966227308283,
14.8228517498124));
#51909=CARTESIAN_POINT('Ctrl Pts',(-1.71604428386948,-1.13012812472696,
14.8189963828945));
#51910=CARTESIAN_POINT('Ctrl Pts',(-1.75529247875725,-1.07053166038305,
14.8151369804607));
#51911=CARTESIAN_POINT('Ctrl Pts',(-1.79141327351683,-1.008917381075,14.811277578027));
#51912=CARTESIAN_POINT('Ctrl Pts',(-1.82420984019043,-0.945651109792833,
14.8074181755933));
#51913=CARTESIAN_POINT('Ctrl Pts',(-1.8570249765243,-0.882349016676732,
14.8035565879372));
#51914=CARTESIAN_POINT('Ctrl Pts',(-1.88651193698957,-0.817393512101275,
14.799695000281));
#51915=CARTESIAN_POINT('Ctrl Pts',(-1.91252167247767,-0.751171361809826,
14.7958334126249));
#51916=CARTESIAN_POINT('Ctrl Pts',(-1.93857691293627,-0.684833353477571,
14.7919650689819));
#51917=CARTESIAN_POINT('Ctrl Pts',(-1.96114262862931,-0.617224735977862,
14.7880967253389));
#51918=CARTESIAN_POINT('Ctrl Pts',(-1.98011956034221,-0.548747746464777,
14.7842283816958));
#51919=CARTESIAN_POINT('Ctrl Pts',(-1.9913875295711,-0.508088032745304,
14.7819314678535));
#51920=CARTESIAN_POINT('Ctrl Pts',(-2.00139119319373,-0.467122383110239,
14.7796345540112));
#51921=CARTESIAN_POINT('Ctrl Pts',(-2.01011838596074,-0.425936188791907,
14.7773376401688));
#51922=CARTESIAN_POINT('Ctrl Pts',(-2.03070219490438,-0.328795128934876,
14.7719201781105));
#51923=CARTESIAN_POINT('Ctrl Pts',(-2.04425025502673,-0.230114996413423,
14.7665027160522));
#51924=CARTESIAN_POINT('Ctrl Pts',(-2.05058606170274,-0.13074542458709,
14.7610852539939));
#51925=CARTESIAN_POINT('Ctrl Pts',(-2.05331903832598,-0.0878819455148026,
14.7587484091501));
#51926=CARTESIAN_POINT('Ctrl Pts',(-2.05471060692694,-0.0448904742936152,
14.7564115643062));
#51927=CARTESIAN_POINT('Ctrl Pts',(-2.05474917537842,-0.00184086438999942,
14.7540747194623));
#51928=CARTESIAN_POINT('Origin',(0.,0.,18.5459252805377));
#51929=CARTESIAN_POINT('',(1.25299305265164,1.63043997671401,15.9061636440672));
#51930=CARTESIAN_POINT('',(1.2504235345857,1.62710269720821,15.8478625066523));
#51931=CARTESIAN_POINT('',(1.25206542099588,1.62921138715835,18.5459252805377));
#51932=CARTESIAN_POINT('',(-2.05150243251667,-0.000517798691100392,15.3959252805377));
#51933=CARTESIAN_POINT('Ctrl Pts',(1.25042353458576,1.62710269720817,15.8478625066523));
#51934=CARTESIAN_POINT('Ctrl Pts',(1.58212812467986,1.36911001369144,15.8251464655206));
#51935=CARTESIAN_POINT('Ctrl Pts',(2.25955063105262,0.431477643030573,15.765386051725));
#51936=CARTESIAN_POINT('Ctrl Pts',(1.86646051514274,-1.55380379648575,15.6685812652657));
#51937=CARTESIAN_POINT('Ctrl Pts',(-0.2930698752374,-2.41082710471087,15.5574481472741));
#51938=CARTESIAN_POINT('Ctrl Pts',(-1.83978745574197,-1.30723126236958,
15.4665628190314));
#51939=CARTESIAN_POINT('Ctrl Pts',(-2.05220371074748,-0.311451552032415,
15.4127218634526));
#51940=CARTESIAN_POINT('Ctrl Pts',(-2.05150243251667,-0.000517798691100392,
15.3959252805377));
#51941=CARTESIAN_POINT('Ctrl Pts',(-2.05150243251667,-0.000517798691100392,
15.3959252805377));
#51942=CARTESIAN_POINT('Ctrl Pts',(-2.05065706210741,0.374303752535962,
15.3756774907888));
#51943=CARTESIAN_POINT('Ctrl Pts',(-1.77290639219337,1.43604706618453,15.318385328376));
#51944=CARTESIAN_POINT('Ctrl Pts',(-0.27952259961467,2.30464022739995,15.235748963112));
#51945=CARTESIAN_POINT('Ctrl Pts',(0.877403861982676,1.91006820299453,15.173360387597));
#51946=CARTESIAN_POINT('Ctrl Pts',(1.25109478256748,1.62792261342726,15.1480161847458));
#51947=CARTESIAN_POINT('',(-2.05474972764537,0.00105794200385854,15.4540747194623));
#51948=CARTESIAN_POINT('Ctrl Pts',(-2.05474972764537,0.00105794200385854,
15.4540747194623));
#51949=CARTESIAN_POINT('Ctrl Pts',(-2.05471842613035,0.0618521814117124,
15.4507619290143));
#51950=CARTESIAN_POINT('Ctrl Pts',(-2.05198927252303,0.122574948398337,
15.4474491385663));
#51951=CARTESIAN_POINT('Ctrl Pts',(-2.04657974197177,0.183054424286241,
15.4441363481182));
#51952=CARTESIAN_POINT('Ctrl Pts',(-2.04026181886476,0.253689884164068,
15.4402672590869));
#51953=CARTESIAN_POINT('Ctrl Pts',(-2.03027037040625,0.32413621977251,15.4363981700556));
#51954=CARTESIAN_POINT('Ctrl Pts',(-2.01662501546903,0.393981102953597,
15.4325290810243));
#51955=CARTESIAN_POINT('Ctrl Pts',(-2.0029999911493,0.463721922179577,15.4286657566631));
#51956=CARTESIAN_POINT('Ctrl Pts',(-1.98573195905279,0.532862594871243,
15.4248024323018));
#51957=CARTESIAN_POINT('Ctrl Pts',(-1.96489232765821,0.600995593336517,
15.4209391079406));
#51958=CARTESIAN_POINT('Ctrl Pts',(-1.94407714070403,0.669048673256756,
15.4170803151759));
#51959=CARTESIAN_POINT('Ctrl Pts',(-1.91969881743501,0.736095964480883,
15.4132215224112));
#51960=CARTESIAN_POINT('Ctrl Pts',(-1.89187950494207,0.80174154269325,15.4093627296466));
#51961=CARTESIAN_POINT('Ctrl Pts',(-1.86407771624265,0.867345769791767,
15.4055063675921));
#51962=CARTESIAN_POINT('Ctrl Pts',(-1.8328394277634,0.931549589438368,15.4016500055377));
#51963=CARTESIAN_POINT('Ctrl Pts',(-1.79833568069386,0.993975020834709,
15.3977936434833));
#51964=CARTESIAN_POINT('Ctrl Pts',(-1.76384212606679,1.05638201169423,15.3939384206022));
#51965=CARTESIAN_POINT('Ctrl Pts',(-1.72608526275411,1.11701123231624,15.390083197721));
#51966=CARTESIAN_POINT('Ctrl Pts',(-1.68528226742459,1.17550892876415,15.3862279748399));
#51967=CARTESIAN_POINT('Ctrl Pts',(-1.64447767657622,1.23400891264651,15.3823726012081));
#51968=CARTESIAN_POINT('Ctrl Pts',(-1.60062699694711,1.29037680970439,15.3785172275763));
#51969=CARTESIAN_POINT('Ctrl Pts',(-1.55398995830775,1.34428894661032,15.3746618539445));
#51970=CARTESIAN_POINT('Ctrl Pts',(-1.50730410359366,1.39825751460579,15.3708024448033));
#51971=CARTESIAN_POINT('Ctrl Pts',(-1.45782638625428,1.44976482300761,15.366943035662));
#51972=CARTESIAN_POINT('Ctrl Pts',(-1.40585536331072,1.4985220251803,15.3630836265208));
#51973=CARTESIAN_POINT('Ctrl Pts',(-1.35385491395087,1.5473068340778,15.3592220321507));
#51974=CARTESIAN_POINT('Ctrl Pts',(-1.29935871995349,1.59333812336112,15.3553604377807));
#51975=CARTESIAN_POINT('Ctrl Pts',(-1.24269847857761,1.63636733462902,15.3514988434106));
#51976=CARTESIAN_POINT('Ctrl Pts',(-1.18593910915725,1.67947182622516,15.3476304931162));
#51977=CARTESIAN_POINT('Ctrl Pts',(-1.12700853520048,1.71956348033388,15.3437621428219));
#51978=CARTESIAN_POINT('Ctrl Pts',(-1.06626687541195,1.75643744918492,15.3398937925276));
#51979=CARTESIAN_POINT('Ctrl Pts',(-1.03020118286736,1.7783315697623,15.3375969383939));
#51980=CARTESIAN_POINT('Ctrl Pts',(-0.99349747827102,1.7990921871023,15.3353000842603));
#51981=CARTESIAN_POINT('Ctrl Pts',(-0.956234625635777,1.81868438802207,
15.3330032301266));
#51982=CARTESIAN_POINT('Ctrl Pts',(-0.893464821043241,1.85168772878371,
15.3291341467111));
#51983=CARTESIAN_POINT('Ctrl Pts',(-0.828861460673923,1.88150225355187,
15.3252650632955));
#51984=CARTESIAN_POINT('Ctrl Pts',(-0.76278159456887,1.90792080587402,15.32139597988));
#51985=CARTESIAN_POINT('Ctrl Pts',(-0.696800183655339,1.93429999607603,
15.3175326611757));
#51986=CARTESIAN_POINT('Ctrl Pts',(-0.62934708115861,1.95729307853427,15.3136693424714));
#51987=CARTESIAN_POINT('Ctrl Pts',(-0.560803393863145,1.97673901057564,
15.3098060237672));
#51988=CARTESIAN_POINT('Ctrl Pts',(-0.492340107551227,1.99616213275482,
15.3059472366928));
#51989=CARTESIAN_POINT('Ctrl Pts',(-0.422789242523565,2.0120462372698,15.3020884496184));
#51990=CARTESIAN_POINT('Ctrl Pts',(-0.35254967690598,2.02427920204044,15.2982296625441));
#51991=CARTESIAN_POINT('Ctrl Pts',(-0.282354356604742,2.03650446102031,
15.2943733061974));
#51992=CARTESIAN_POINT('Ctrl Pts',(-0.211471673866081,2.04508306012134,
15.2905169498507));
#51993=CARTESIAN_POINT('Ctrl Pts',(-0.140311951151932,2.04995368700465,
15.286660593504));
#51994=CARTESIAN_POINT('Ctrl Pts',(-0.069173249287603,2.05482287508644,
15.2828053763394));
#51995=CARTESIAN_POINT('Ctrl Pts',(0.00224184569476071,2.05598623236786,
15.2789501591749));
#51996=CARTESIAN_POINT('Ctrl Pts',(0.0735183420835199,2.05343434661965,
15.2750949420104));
#51997=CARTESIAN_POINT('Ctrl Pts',(0.144797625594737,2.05088236108514,15.2712395740954));
#51998=CARTESIAN_POINT('Ctrl Pts',(0.215937814359383,2.04461486367519,15.2673842061804));
#51999=CARTESIAN_POINT('Ctrl Pts',(0.286526108375765,2.03467450756111,15.2635288382655));
#52000=CARTESIAN_POINT('Ctrl Pts',(0.357188289632059,2.02472374652809,15.2596694348019));
#52001=CARTESIAN_POINT('Ctrl Pts',(0.427296940924071,2.01109252016697,15.2558100313383));
#52002=CARTESIAN_POINT('Ctrl Pts',(0.496447462142931,1.99387499102422,15.2519506278747));
#52003=CARTESIAN_POINT('Ctrl Pts',(0.565637137250949,1.97664771310133,15.2480890391686));
#52004=CARTESIAN_POINT('Ctrl Pts',(0.633867137467881,1.95583023191119,15.2442274504625));
#52005=CARTESIAN_POINT('Ctrl Pts',(0.700748735555524,1.9315664037556,15.2403658617565));
#52006=CARTESIAN_POINT('Ctrl Pts',(0.767747345736748,1.90726012503943,15.2364975170429));
#52007=CARTESIAN_POINT('Ctrl Pts',(0.833392396257111,1.8794956505322,15.2326291723293));
#52008=CARTESIAN_POINT('Ctrl Pts',(0.897316467401261,1.84846442211651,15.2287608276157));
#52009=CARTESIAN_POINT('Ctrl Pts',(0.935272632051664,1.8300390247041,15.2264639224555));
#52010=CARTESIAN_POINT('Ctrl Pts',(0.972622522132005,1.81046277088973,15.2241670172953));
#52011=CARTESIAN_POINT('Ctrl Pts',(1.00929402677359,1.78978298405677,15.2218701121351));
#52012=CARTESIAN_POINT('Ctrl Pts',(1.07106081302598,1.75495147153661,15.2180013739565));
#52013=CARTESIAN_POINT('Ctrl Pts',(1.13114335760791,1.71685056090996,15.2141326357779));
#52014=CARTESIAN_POINT('Ctrl Pts',(1.18917406150476,1.67566781133501,15.2102638975993));
#52015=CARTESIAN_POINT('Ctrl Pts',(1.21041838950633,1.66059131249516,15.2088476000654));
#52016=CARTESIAN_POINT('Ctrl Pts',(1.23138793186196,1.64510224658988,15.2074313025316));
#52017=CARTESIAN_POINT('Ctrl Pts',(1.25206542099588,1.62921138715835,15.2060150049977));
#52018=CARTESIAN_POINT('Ctrl Pts',(1.25299305265161,1.63043997671403,15.9061636440672));
#52019=CARTESIAN_POINT('Ctrl Pts',(1.33870026031667,1.5658514984805,15.9003320360729));
#52020=CARTESIAN_POINT('Ctrl Pts',(1.92956475440913,1.0413794257925,15.8574560554148));
#52021=CARTESIAN_POINT('Ctrl Pts',(2.35999751615834,-0.573068146683373,
15.7775357020929));
#52022=CARTESIAN_POINT('Ctrl Pts',(0.798563541884426,-2.29352622680378,
15.6664025841013));
#52023=CARTESIAN_POINT('Ctrl Pts',(-1.42540407770296,-1.92615524732257,
15.5585825778216));
#52024=CARTESIAN_POINT('Ctrl Pts',(-2.05354142278375,-0.618786125786745,
15.4878069442056));
#52025=CARTESIAN_POINT('Ctrl Pts',(-2.05744064634435,0.00104161743516934,
15.4540756832536));
#52026=CARTESIAN_POINT('Origin',(0.,0.,18.5459252805377));
#52027=CARTESIAN_POINT('',(1.25005477124305,1.62658000731212,16.6061086772888));
#52028=CARTESIAN_POINT('',(1.25371187806425,1.63132526051507,16.5478693678287));
#52029=CARTESIAN_POINT('',(1.25206542099588,1.62921138715835,18.5459252805377));
#52030=CARTESIAN_POINT('',(-2.05269453305337,-0.0025315228670039,16.8540747194623));
#52031=CARTESIAN_POINT('Ctrl Pts',(-2.05269453305337,-0.0025315228670039,
16.8540747194623));
#52032=CARTESIAN_POINT('Ctrl Pts',(-2.04912705821622,0.467702877218055,
16.8286277343139));
#52033=CARTESIAN_POINT('Ctrl Pts',(-1.65656296491944,1.62962812348302,16.7661363765015));
#52034=CARTESIAN_POINT('Ctrl Pts',(-0.0552297434345721,2.27982805376088,
16.6834810291103));
#52035=CARTESIAN_POINT('Ctrl Pts',(0.953586651517499,1.85321350766304,16.6262726668676));
#52036=CARTESIAN_POINT('Ctrl Pts',(1.25005477124305,1.62658000731212,16.6061086772888));
#52037=CARTESIAN_POINT('',(-0.530170217188714,-1.9851743256717,17.));
#52038=CARTESIAN_POINT('Ctrl Pts',(-0.5301702171887,-1.9851743256717,17.));
#52039=CARTESIAN_POINT('Ctrl Pts',(-1.19025956241818,-1.80888768575364,
16.9629556273361));
#52040=CARTESIAN_POINT('Ctrl Pts',(-1.9249882932336,-1.11315381096668,16.9143138671569));
#52041=CARTESIAN_POINT('Ctrl Pts',(-2.05432039906053,-0.216839446930442,
16.8656721069777));
#52042=CARTESIAN_POINT('Ctrl Pts',(-2.05269453305337,-0.0025315228670039,
16.8540747194623));
#52043=CARTESIAN_POINT('',(0.530281684557416,-1.98514455330662,16.9999999985106));
#52044=CARTESIAN_POINT('Origin',(0.,0.,17.));
#52045=CARTESIAN_POINT('',(-2.05474946839643,0.00147804755778122,16.7959252805377));
#52046=CARTESIAN_POINT('Ctrl Pts',(0.530281684557416,-1.98514455330662,
16.9999999985106));
#52047=CARTESIAN_POINT('Ctrl Pts',(0.461903534585254,-2.00341006474949,
16.9961388750594));
#52048=CARTESIAN_POINT('Ctrl Pts',(0.392444315027901,-2.01817488207207,
16.9922777516081));
#52049=CARTESIAN_POINT('Ctrl Pts',(0.322296520861052,-2.02931577511753,
16.9884166281568));
#52050=CARTESIAN_POINT('Ctrl Pts',(0.248587777035769,-2.0410222192221,16.9843595004492));
#52051=CARTESIAN_POINT('Ctrl Pts',(0.174119182236965,-2.04872680208598,
16.9803023727415));
#52052=CARTESIAN_POINT('Ctrl Pts',(0.0993639973638922,-2.05234606207819,
16.9762452450338));
#52053=CARTESIAN_POINT('Ctrl Pts',(0.0284118419057885,-2.05578119902618,
16.9723945160668));
#52054=CARTESIAN_POINT('Ctrl Pts',(-0.042797896797022,-2.05553648246812,
16.9685437870997));
#52055=CARTESIAN_POINT('Ctrl Pts',(-0.113852662049382,-2.05159331589969,
16.9646930581327));
#52056=CARTESIAN_POINT('Ctrl Pts',(-0.184864600835995,-2.04765252597534,
16.9608446500953));
#52057=CARTESIAN_POINT('Ctrl Pts',(-0.255721265268953,-2.04001773536084,
16.9569962420579));
#52058=CARTESIAN_POINT('Ctrl Pts',(-0.326010522590318,-2.02872243090581,
16.9531478340205));
#52059=CARTESIAN_POINT('Ctrl Pts',(-0.396281187004936,-2.0174301142835,
16.9493004439636));
#52060=CARTESIAN_POINT('Ctrl Pts',(-0.465984260690645,-2.00247928372715,
16.9454530539067));
#52061=CARTESIAN_POINT('Ctrl Pts',(-0.53471491016292,-1.98395502150363,
16.9416056638498));
#52062=CARTESIAN_POINT('Ctrl Pts',(-0.603450623543465,-1.9654293944572,
16.9377579903265));
#52063=CARTESIAN_POINT('Ctrl Pts',(-0.671213300002006,-1.94332994266954,
16.9339103168031));
#52064=CARTESIAN_POINT('Ctrl Pts',(-0.737612151282778,-1.91779192739463,
16.9300626432798));
#52065=CARTESIAN_POINT('Ctrl Pts',(-0.804080286638563,-1.89222726440319,
16.9262109548903));
#52066=CARTESIAN_POINT('Ctrl Pts',(-0.869181301035828,-1.86321705420353,
16.9223592665009));
#52067=CARTESIAN_POINT('Ctrl Pts',(-0.932544247534814,-1.83094478040429,
16.9185075781114));
#52068=CARTESIAN_POINT('Ctrl Pts',(-0.995945525859085,-1.79865298328379,
16.9146535596181));
#52069=CARTESIAN_POINT('Ctrl Pts',(-1.05760622149396,-1.76309543961573,
16.9107995411247));
#52070=CARTESIAN_POINT('Ctrl Pts',(-1.11718225388515,-1.72450032592171,
16.9069455226314));
#52071=CARTESIAN_POINT('Ctrl Pts',(-1.17685661880791,-1.68584150950894,
16.9030851429324));
#52072=CARTESIAN_POINT('Ctrl Pts',(-1.23443906058148,-1.64413540551827,
16.8992247632333));
#52073=CARTESIAN_POINT('Ctrl Pts',(-1.28961731996744,-1.59965144032692,
16.8953643835343));
#52074=CARTESIAN_POINT('Ctrl Pts',(-1.31019431055133,-1.58306254928428,
16.8939247767472));
#52075=CARTESIAN_POINT('Ctrl Pts',(-1.33043731809827,-1.56608772108779,
16.89248516996));
#52076=CARTESIAN_POINT('Ctrl Pts',(-1.35033149230716,-1.54874220688387,
16.8910455631728));
#52077=CARTESIAN_POINT('Ctrl Pts',(-1.40510164118834,-1.50098870953365,
16.887082218063));
#52078=CARTESIAN_POINT('Ctrl Pts',(-1.45745853908989,-1.45021867236757,
16.8831188729532));
#52079=CARTESIAN_POINT('Ctrl Pts',(-1.50704767249473,-1.39671216624193,
16.8791555278434));
#52080=CARTESIAN_POINT('Ctrl Pts',(-1.55473296292161,-1.34525990020817,
16.8753443448352));
#52081=CARTESIAN_POINT('Ctrl Pts',(-1.59985872901899,-1.29127783962401,
16.8715331618271));
#52082=CARTESIAN_POINT('Ctrl Pts',(-1.64214309495677,-1.23505611944794,
16.8677219788189));
#52083=CARTESIAN_POINT('Ctrl Pts',(-1.68438888372789,-1.17888569186242,
16.8639142728557));
#52084=CARTESIAN_POINT('Ctrl Pts',(-1.72379811160458,-1.12048005229482,
16.8601065668925));
#52085=CARTESIAN_POINT('Ctrl Pts',(-1.76012795126868,-1.06016374096774,
16.8562988609293));
#52086=CARTESIAN_POINT('Ctrl Pts',(-1.79643756910928,-0.999881002753381,
16.8524932744018));
#52087=CARTESIAN_POINT('Ctrl Pts',(-1.82967094081488,-0.937690129505748,
16.8486876878742));
#52088=CARTESIAN_POINT('Ctrl Pts',(-1.85962861413517,-0.873944494799123,
16.8448821013467));
#52089=CARTESIAN_POINT('Ctrl Pts',(-1.8895802663825,-0.810211672072712,
16.8410772796888));
#52090=CARTESIAN_POINT('Ctrl Pts',(-1.91625731622662,-0.744925161216608,
16.8372724580309));
#52091=CARTESIAN_POINT('Ctrl Pts',(-1.93950719738421,-0.67846104810436,
16.833467636373));
#52092=CARTESIAN_POINT('Ctrl Pts',(-1.96277242162608,-0.611953073929635,
16.8296603038334));
#52093=CARTESIAN_POINT('Ctrl Pts',(-1.98260579677084,-0.544266418605556,
16.8258529712939));
#52094=CARTESIAN_POINT('Ctrl Pts',(-1.99890412464787,-0.475793929097164,
16.8220456387543));
#52095=CARTESIAN_POINT('Ctrl Pts',(-2.01520895611267,-0.407294116734022,
16.8182367869595));
#52096=CARTESIAN_POINT('Ctrl Pts',(-2.02797584107969,-0.338008337619496,
16.8144279351646));
#52097=CARTESIAN_POINT('Ctrl Pts',(-2.03715290029361,-0.268338635543442,
16.8106190833698));
#52098=CARTESIAN_POINT('Ctrl Pts',(-2.04634216010382,-0.198576309905946,
16.8068051678326));
#52099=CARTESIAN_POINT('Ctrl Pts',(-2.05193203507066,-0.128429540871885,
16.8029912522954));
#52100=CARTESIAN_POINT('Ctrl Pts',(-2.05392266042328,-0.0583032374721763,
16.7991773367582));
#52101=CARTESIAN_POINT('Ctrl Pts',(-2.05448845040103,-0.038371430822669,
16.7980933180181));
#52102=CARTESIAN_POINT('Ctrl Pts',(-2.05476379699637,-0.0184412594723448,
16.7970092992779));
#52103=CARTESIAN_POINT('Ctrl Pts',(-2.05474946839643,0.00147804755778125,
16.7959252805377));
#52104=CARTESIAN_POINT('Ctrl Pts',(-2.05654452918444,0.00147933880289632,
16.7959252805377));
#52105=CARTESIAN_POINT('Ctrl Pts',(-2.05736468201256,0.099646559291543,
16.7905876687522));
#52106=CARTESIAN_POINT('Ctrl Pts',(-2.00636216552464,0.87829705013526,16.7482056843029));
#52107=CARTESIAN_POINT('Ctrl Pts',(-1.01136481471932,2.20819937049432,16.6687793271897));
#52108=CARTESIAN_POINT('Ctrl Pts',(0.601793643796052,2.09609164757904,16.5914316347388));
#52109=CARTESIAN_POINT('Ctrl Pts',(1.20647580811204,1.66813506378572,16.5511283149519));
#52110=CARTESIAN_POINT('Ctrl Pts',(1.25371187806425,1.63132526051507,16.5478693678287));
#52111=CARTESIAN_POINT('Origin',(0.,0.,11.));
#52112=CARTESIAN_POINT('',(-1.56343130033213,0.575533291080357,6.73212871955268));
#52113=CARTESIAN_POINT('',(-1.56343130033213,0.575533291080354,6.53916105310504));
#52114=CARTESIAN_POINT('',(-1.56343130033213,0.575533291080363,11.));
#52115=CARTESIAN_POINT('',(-0.769902040670541,-1.47743251885537,6.));
#52116=CARTESIAN_POINT('Ctrl Pts',(-1.56343130033213,0.575533291080354,
6.53916105310504));
#52117=CARTESIAN_POINT('Ctrl Pts',(-1.54247217282036,0.6324685830737,6.5350982232025));
#52118=CARTESIAN_POINT('Ctrl Pts',(-1.51836822901476,0.688340720433169,
6.53103539329996));
#52119=CARTESIAN_POINT('Ctrl Pts',(-1.49125198995376,0.742780924942838,
6.52697256339742));
#52120=CARTESIAN_POINT('Ctrl Pts',(-1.46415901312368,0.79717442678827,6.52291321887821));
#52121=CARTESIAN_POINT('Ctrl Pts',(-1.43405909049039,0.850137972438081,
6.51885387435899));
#52122=CARTESIAN_POINT('Ctrl Pts',(-1.40113273296279,0.901322952453898,
6.51479452983978));
#52123=CARTESIAN_POINT('Ctrl Pts',(-1.36822229829313,0.95248317992415,6.51073714837906));
#52124=CARTESIAN_POINT('Ctrl Pts',(-1.33248841656539,1.00186611597768,6.50667976691835));
#52125=CARTESIAN_POINT('Ctrl Pts',(-1.29415635636569,1.04914981069354,6.50262238545764));
#52126=CARTESIAN_POINT('Ctrl Pts',(-1.25582848671796,1.09642833624345,6.49856544755951));
#52127=CARTESIAN_POINT('Ctrl Pts',(-1.21490332691312,1.14160767809269,6.49450850966139));
#52128=CARTESIAN_POINT('Ctrl Pts',(-1.17164677677384,1.18439850999378,6.49045157176326));
#52129=CARTESIAN_POINT('Ctrl Pts',(-1.12834727602848,1.22723183007663,6.48639060562107));
#52130=CARTESIAN_POINT('Ctrl Pts',(-1.08271212759999,1.26767154162889,6.48232963947888));
#52131=CARTESIAN_POINT('Ctrl Pts',(-1.0350435982904,1.30546572135697,6.47826867333669));
#52132=CARTESIAN_POINT('Ctrl Pts',(-0.987351235684329,1.34327879740729,
6.4742056767939));
#52133=CARTESIAN_POINT('Ctrl Pts',(-0.937623887328302,1.3784434103523,6.47014268025112));
#52134=CARTESIAN_POINT('Ctrl Pts',(-0.88619381793384,1.41075033831498,6.46607968370834));
#52135=CARTESIAN_POINT('Ctrl Pts',(-0.83466622959496,1.44311852494501,6.46200898312902));
#52136=CARTESIAN_POINT('Ctrl Pts',(-0.781429921829616,1.47261795464689,
6.45793828254969));
#52137=CARTESIAN_POINT('Ctrl Pts',(-0.726841985000047,1.49908529738677,
6.45386758197037));
#52138=CARTESIAN_POINT('Ctrl Pts',(-0.685114164012645,1.51931732306875,
6.45075587863566));
#52139=CARTESIAN_POINT('Ctrl Pts',(-0.642597072760685,1.53777855804026,
6.44764417530095));
#52140=CARTESIAN_POINT('Ctrl Pts',(-0.599456592805752,1.55441557935506,
6.44453247196624));
#52141=CARTESIAN_POINT('Ctrl Pts',(-0.542819354942529,1.5762575925762,6.44044725357943));
#52142=CARTESIAN_POINT('Ctrl Pts',(-0.484871782532727,1.59504445632831,
6.43636203519262));
#52143=CARTESIAN_POINT('Ctrl Pts',(-0.425975071864993,1.61062138261902,
6.43227681680581));
#52144=CARTESIAN_POINT('Ctrl Pts',(-0.366578437783686,1.62633052801121,
6.42815692252118));
#52145=CARTESIAN_POINT('Ctrl Pts',(-0.306216934237057,1.63877471927378,
6.42403702823655));
#52146=CARTESIAN_POINT('Ctrl Pts',(-0.245281539516207,1.64784494609552,
6.41991713395192));
#52147=CARTESIAN_POINT('Ctrl Pts',(-0.185026578161849,1.65681389048529,
6.41584324435062));
#52148=CARTESIAN_POINT('Ctrl Pts',(-0.124210992214787,1.66248375485769,
6.41176935474932));
#52149=CARTESIAN_POINT('Ctrl Pts',(-0.0632254082952299,1.66479985215818,
6.40769546514802));
#52150=CARTESIAN_POINT('Ctrl Pts',(-0.00227792857393501,1.66711450234568,
6.40362412094002));
#52151=CARTESIAN_POINT('Ctrl Pts',(0.0588388300897228,1.66607952143167,
6.39955277673203));
#52152=CARTESIAN_POINT('Ctrl Pts',(0.119729966205783,1.66169213008679,6.39548143252403));
#52153=CARTESIAN_POINT('Ctrl Pts',(0.180605449286772,1.65730586659063,6.39141113491982));
#52154=CARTESIAN_POINT('Ctrl Pts',(0.241254916691805,1.64956894018868,6.38734083731562));
#52155=CARTESIAN_POINT('Ctrl Pts',(0.301286393336598,1.63853059452371,6.38327053971141));
#52156=CARTESIAN_POINT('Ctrl Pts',(0.362580865570188,1.62726001432676,6.37911460756668));
#52157=CARTESIAN_POINT('Ctrl Pts',(0.423230495090953,1.61254755918519,6.37495867542195));
#52158=CARTESIAN_POINT('Ctrl Pts',(0.482829061560443,1.59450057927636,6.37080274327722));
#52159=CARTESIAN_POINT('Ctrl Pts',(0.541270234380646,1.57680406853438,6.36672751860175));
#52160=CARTESIAN_POINT('Ctrl Pts',(0.598700337090838,1.55590163855073,6.36265229392628));
#52161=CARTESIAN_POINT('Ctrl Pts',(0.654754249728767,1.53194414795779,6.35857706925082));
#52162=CARTESIAN_POINT('Ctrl Pts',(0.712473335378472,1.50727496098385,6.35438078337146));
#52163=CARTESIAN_POINT('Ctrl Pts',(0.768732632032523,1.47936654553491,6.3501844974921));
#52164=CARTESIAN_POINT('Ctrl Pts',(0.823160899611873,1.44843437315958,6.34598821161275));
#52165=CARTESIAN_POINT('Ctrl Pts',(0.877589167191229,1.41750220078424,6.34179192573339));
#52166=CARTESIAN_POINT('Ctrl Pts',(0.930185952300682,1.38354664391381,6.33759563985403));
#52167=CARTESIAN_POINT('Ctrl Pts',(0.980614989643535,1.34682970047679,6.33339935397468));
#52168=CARTESIAN_POINT('Ctrl Pts',(1.02968244606439,1.3111041122655,6.32931636755725));
#52169=CARTESIAN_POINT('Ctrl Pts',(1.07689333142065,1.27262204689111,6.32523338113982));
#52170=CARTESIAN_POINT('Ctrl Pts',(1.12192208578457,1.23160335880867,6.32115039472239));
#52171=CARTESIAN_POINT('Ctrl Pts',(1.16736095126946,1.19021108232949,6.31703022144159));
#52172=CARTESIAN_POINT('Ctrl Pts',(1.21057726258409,1.14623598390422,6.31291004816079));
#52173=CARTESIAN_POINT('Ctrl Pts',(1.25126733031905,1.09994821154281,6.30878987487998));
#52174=CARTESIAN_POINT('Ctrl Pts',(1.29148153737639,1.0542017636851,6.3047178860471));
#52175=CARTESIAN_POINT('Ctrl Pts',(1.32922792601312,1.00619683655384,6.30064589721421));
#52176=CARTESIAN_POINT('Ctrl Pts',(1.36424921820571,0.956232226305472,6.29657390838132));
#52177=CARTESIAN_POINT('Ctrl Pts',(1.39924971771825,0.906297280814998,6.29250433715085));
#52178=CARTESIAN_POINT('Ctrl Pts',(1.4315280368189,0.854405376351585,6.28843476592039));
#52179=CARTESIAN_POINT('Ctrl Pts',(1.46086825225904,0.800886976758657,6.28436519468992));
#52180=CARTESIAN_POINT('Ctrl Pts',(1.49020185549971,0.747380638233718,6.28029654059031));
#52181=CARTESIAN_POINT('Ctrl Pts',(1.51659842460062,0.692248979560936,6.2762278864907));
#52182=CARTESIAN_POINT('Ctrl Pts',(1.53988738324474,0.635848131965233,6.27215923239108));
#52183=CARTESIAN_POINT('Ctrl Pts',(1.56368632472775,0.578212215648232,6.26800148269042));
#52184=CARTESIAN_POINT('Ctrl Pts',(1.58423968049731,0.519251356928695,6.26384373298975));
#52185=CARTESIAN_POINT('Ctrl Pts',(1.60141775831342,0.459366045064748,6.25968598328909));
#52186=CARTESIAN_POINT('Ctrl Pts',(1.61824946449418,0.400688235787859,6.25561206872869));
#52187=CARTESIAN_POINT('Ctrl Pts',(1.63184070452812,0.341123435405091,6.25153815416829));
#52188=CARTESIAN_POINT('Ctrl Pts',(1.64212094537824,0.281060137248377,6.24746423960789));
#52189=CARTESIAN_POINT('Ctrl Pts',(1.65271851447157,0.219142818241058,6.2432645723371));
#52190=CARTESIAN_POINT('Ctrl Pts',(1.6597972102613,0.156696296827122,6.2390649050663));
#52191=CARTESIAN_POINT('Ctrl Pts',(1.66333751254052,0.0941505144729865,
6.2348652377955));
#52192=CARTESIAN_POINT('Ctrl Pts',(1.66687781481973,0.0316047321188593,
6.23066557052471));
#52193=CARTESIAN_POINT('Ctrl Pts',(1.66687979361413,-0.0310397249814722,
6.22646590325391));
#52194=CARTESIAN_POINT('Ctrl Pts',(1.66338222244431,-0.093357281752649,
6.22226623598312));
#52195=CARTESIAN_POINT('Ctrl Pts',(1.66002325794814,-0.153205230662976,
6.21823299903858));
#52196=CARTESIAN_POINT('Ctrl Pts',(1.6534222319083,-0.213010620528822,6.21419976209404));
#52197=CARTESIAN_POINT('Ctrl Pts',(1.64358156678773,-0.272388754018175,
6.2101665251495));
#52198=CARTESIAN_POINT('Ctrl Pts',(1.63351361341894,-0.333138334638226,
6.20604013318458));
#52199=CARTESIAN_POINT('Ctrl Pts',(1.62005441559245,-0.393440119787072,
6.20191374121967));
#52200=CARTESIAN_POINT('Ctrl Pts',(1.60326314871747,-0.452883291770124,
6.19778734925476));
#52201=CARTESIAN_POINT('Ctrl Pts',(1.58689626677036,-0.51082408835517,6.19376524832216));
#52202=CARTESIAN_POINT('Ctrl Pts',(1.56736391839693,-0.567948626115506,
6.18974314738957));
#52203=CARTESIAN_POINT('Ctrl Pts',(1.54477275985811,-0.623885502636782,
6.18572104645698));
#52204=CARTESIAN_POINT('Ctrl Pts',(1.52219478243197,-0.67978974204158,6.18170129227281));
#52205=CARTESIAN_POINT('Ctrl Pts',(1.4965617259929,-0.73450720808756,6.17768153808864));
#52206=CARTESIAN_POINT('Ctrl Pts',(1.46802939675063,-0.787683750166262,
6.17366178390447));
#52207=CARTESIAN_POINT('Ctrl Pts',(1.43950256879724,-0.840850039330887,
6.16964280476494));
#52208=CARTESIAN_POINT('Ctrl Pts',(1.40807782472183,-0.892475532430629,
6.16562382562542));
#52209=CARTESIAN_POINT('Ctrl Pts',(1.37395720126328,-0.94223012533923,6.16160484648589));
#52210=CARTESIAN_POINT('Ctrl Pts',(1.33824898649299,-0.994299739235551,
6.15739886911136));
#52211=CARTESIAN_POINT('Ctrl Pts',(1.29958818278729,-1.04431954101807,6.15319289173684));
#52212=CARTESIAN_POINT('Ctrl Pts',(1.25825577968416,-1.0919470650592,6.14898691436231));
#52213=CARTESIAN_POINT('Ctrl Pts',(1.21870051728244,-1.13752678144517,6.14496177848308));
#52214=CARTESIAN_POINT('Ctrl Pts',(1.1766991429464,-1.18091540677872,6.14093664260385));
#52215=CARTESIAN_POINT('Ctrl Pts',(1.13253587503068,-1.2218504375612,6.13691150672463));
#52216=CARTESIAN_POINT('Ctrl Pts',(1.08833659888746,-1.26281884444944,6.13288308897756));
#52217=CARTESIAN_POINT('Ctrl Pts',(1.04197233113928,-1.3013293507988,6.1288546712305));
#52218=CARTESIAN_POINT('Ctrl Pts',(0.993759007638126,-1.33716081109868,
6.12482625348344));
#52219=CARTESIAN_POINT('Ctrl Pts',(0.945455378020833,-1.37305938562717,
6.12079029029594));
#52220=CARTESIAN_POINT('Ctrl Pts',(0.895296228032955,-1.40626863101897,
6.11675432710843));
#52221=CARTESIAN_POINT('Ctrl Pts',(0.84362365034703,-1.4366123821599,6.11271836392093));
#52222=CARTESIAN_POINT('Ctrl Pts',(0.836858330675631,-1.44058518912428,
6.11218994861114));
#52223=CARTESIAN_POINT('Ctrl Pts',(0.830067096357697,-1.44450894389794,
6.11166153330135));
#52224=CARTESIAN_POINT('Ctrl Pts',(0.823250739277983,-1.44838331262075,
6.11113311799157));
#52225=CARTESIAN_POINT('Ctrl Pts',(0.769183237850171,-1.47911489460841,
6.10694171557788));
#52226=CARTESIAN_POINT('Ctrl Pts',(0.713301855134838,-1.50686694462979,
6.1027503131642));
#52227=CARTESIAN_POINT('Ctrl Pts',(0.655958678299715,-1.53142881400452,
6.09855891075051));
#52228=CARTESIAN_POINT('Ctrl Pts',(0.59873760766417,-1.5559383814893,6.09437643348273));
#52229=CARTESIAN_POINT('Ctrl Pts',(0.540061369584661,-1.57727109296317,
6.09019395621495));
#52230=CARTESIAN_POINT('Ctrl Pts',(0.480306060998282,-1.59526238837638,
6.08601147894716));
#52231=CARTESIAN_POINT('Ctrl Pts',(0.420626058013942,-1.61323101056834,
6.08183427257457));
#52232=CARTESIAN_POINT('Ctrl Pts',(0.35987013933105,-1.62786644215779,6.07765706620198));
#52233=CARTESIAN_POINT('Ctrl Pts',(0.298432871660621,-1.63905272066288,
6.07347985982939));
#52234=CARTESIAN_POINT('Ctrl Pts',(0.237054984453405,-1.65022818738509,
6.06930669081814));
#52235=CARTESIAN_POINT('Ctrl Pts',(0.174997524326245,-1.65796103802397,
6.06513352180688));
#52236=CARTESIAN_POINT('Ctrl Pts',(0.112667056339353,-1.66218595061318,
6.06096035279563));
#52237=CARTESIAN_POINT('Ctrl Pts',(0.0503785495936725,-1.66640801896613,
6.05678999318654));
#52238=CARTESIAN_POINT('Ctrl Pts',(-0.012182124448017,-1.66712681027999,
6.05261963357745));
#52239=CARTESIAN_POINT('Ctrl Pts',(-0.0746030895967543,-1.66432880736428,
6.04844927396836));
#52240=CARTESIAN_POINT('Ctrl Pts',(-0.137019316940818,-1.66153101681939,
6.04427923089314));
#52241=CARTESIAN_POINT('Ctrl Pts',(-0.199295379105893,-1.65521697056048,
6.04010918781791));
#52242=CARTESIAN_POINT('Ctrl Pts',(-0.261020497571679,-1.64542526413309,
6.03593914474268));
#52243=CARTESIAN_POINT('Ctrl Pts',(-0.322737670498844,-1.63563481813878,
6.03176963845441));
#52244=CARTESIAN_POINT('Ctrl Pts',(-0.383903569929177,-1.6223676827034,
6.02760013216614));
#52245=CARTESIAN_POINT('Ctrl Pts',(-0.444115707757167,-1.60571393408769,
6.02343062587786));
#52246=CARTESIAN_POINT('Ctrl Pts',(-0.504373373391242,-1.58904759318302,
6.01925796692834));
#52247=CARTESIAN_POINT('Ctrl Pts',(-0.563675376158753,-1.56898965280899,
6.01508530797882));
#52248=CARTESIAN_POINT('Ctrl Pts',(-0.621633450291989,-1.54568038529253,
6.01091264902929));
#52249=CARTESIAN_POINT('Ctrl Pts',(-0.672158876970822,-1.52536034007963,
6.00727509935286));
#52250=CARTESIAN_POINT('Ctrl Pts',(-0.721663027466453,-1.50257025897668,
6.00363754967643));
#52251=CARTESIAN_POINT('Ctrl Pts',(-0.769902040670518,-1.47743251885539,
6.));
#52252=CARTESIAN_POINT('',(-1.33524939639864,0.997598393459654,6.00000056028684));
#52253=CARTESIAN_POINT('Origin',(0.,0.,6.));
#52254=CARTESIAN_POINT('',(-1.56343130033213,0.575533291080356,6.03223733991315));
#52255=CARTESIAN_POINT('Ctrl Pts',(-1.33464070599239,0.99714100603081,6.00000056115665));
#52256=CARTESIAN_POINT('Ctrl Pts',(-1.37078624190903,0.948761385412975,
6.00406393220756));
#52257=CARTESIAN_POINT('Ctrl Pts',(-1.40437715109543,0.898307539445458,
6.00812730325847));
#52258=CARTESIAN_POINT('Ctrl Pts',(-1.43516660948121,0.846080848991512,
6.01219067430938));
#52259=CARTESIAN_POINT('Ctrl Pts',(-1.46590351276494,0.79394330525176,6.01624710951629));
#52260=CARTESIAN_POINT('Ctrl Pts',(-1.49384819256357,0.7400393601093,6.02030354472319));
#52261=CARTESIAN_POINT('Ctrl Pts',(-1.51879562492657,0.684701285016984,
6.0243599799301));
#52262=CARTESIAN_POINT('Ctrl Pts',(-1.53494444323233,0.64888018298719,6.02698576659112));
#52263=CARTESIAN_POINT('Ctrl Pts',(-1.54983820983774,0.612458806035863,
6.02961155325213));
#52264=CARTESIAN_POINT('Ctrl Pts',(-1.56343130033213,0.575533291080356,
6.03223733991315));
#52265=CARTESIAN_POINT('',(-1.56343130033213,0.575533291080363,5.));
#52266=CARTESIAN_POINT('',(-1.56343130033213,0.575533291080363,11.));
#52267=CARTESIAN_POINT('Origin',(0.,0.,5.));
#52268=CARTESIAN_POINT('',(-1.66599954285828,-0.001234178273358,6.07148036342561));
#52269=CARTESIAN_POINT('Ctrl Pts',(-1.56343130033213,0.575533291080356,
6.03223733991315));
#52270=CARTESIAN_POINT('Ctrl Pts',(-1.58439805255523,0.518577286623392,
6.03628750189324));
#52271=CARTESIAN_POINT('Ctrl Pts',(-1.60226784904869,0.460421099189002,
6.04033766387333));
#52272=CARTESIAN_POINT('Ctrl Pts',(-1.61691251877963,0.401434809917774,
6.04438782585341));
#52273=CARTESIAN_POINT('Ctrl Pts',(-1.63155002543007,0.342477372341142,
6.04843600679625));
#52274=CARTESIAN_POINT('Ctrl Pts',(-1.64296541408166,0.282691138748249,
6.05248418773908));
#52275=CARTESIAN_POINT('Ctrl Pts',(-1.65108070322902,0.222460134461837,
6.05653236868192));
#52276=CARTESIAN_POINT('Ctrl Pts',(-1.65919668658871,0.162223977788912,
6.06058089592137));
#52277=CARTESIAN_POINT('Ctrl Pts',(-1.66401193639875,0.101543484887501,
6.06462942316082));
#52278=CARTESIAN_POINT('Ctrl Pts',(-1.66550009488837,0.04080972833555,6.06867795040027));
#52279=CARTESIAN_POINT('Ctrl Pts',(-1.66584346540607,0.0267963140556828,
6.06961208806358));
#52280=CARTESIAN_POINT('Ctrl Pts',(-1.66600992466137,0.0127800747921988,
6.0705462257269));
#52281=CARTESIAN_POINT('Ctrl Pts',(-1.66599954285867,-0.00123417774222995,
6.07148036339021));
#52282=CARTESIAN_POINT('Ctrl Pts',(-1.66599954285828,-0.00123417827337041,
6.07148036342561));
#52283=CARTESIAN_POINT('Ctrl Pts',(-1.66594753062002,-0.0714447524100149,
6.07616033772347));
#52284=CARTESIAN_POINT('Ctrl Pts',(-1.66145315819263,-0.141478574425917,
6.08084031202132));
#52285=CARTESIAN_POINT('Ctrl Pts',(-1.6526070389996,-0.210822139845356,
6.08552028631918));
#52286=CARTESIAN_POINT('Ctrl Pts',(-1.64367765414105,-0.280818413870458,
6.09024431170498));
#52287=CARTESIAN_POINT('Ctrl Pts',(-1.63031432693859,-0.350111196841199,
6.09496833709077));
#52288=CARTESIAN_POINT('Ctrl Pts',(-1.61265978947049,-0.418191826109729,
6.09969236247657));
#52289=CARTESIAN_POINT('Ctrl Pts',(-1.60112177366817,-0.462685508130673,
6.10277972059345));
#52290=CARTESIAN_POINT('Ctrl Pts',(-1.58775190295344,-0.506661860727517,
6.10586707871033));
#52291=CARTESIAN_POINT('Ctrl Pts',(-1.57260095361437,-0.549983854936836,
6.10895443682722));
#52292=CARTESIAN_POINT('Ctrl Pts',(-1.55255693979627,-0.607296874149416,
6.11303887057267));
#52293=CARTESIAN_POINT('Ctrl Pts',(-1.52933597420523,-0.663626358690032,
6.11712330431812));
#52294=CARTESIAN_POINT('Ctrl Pts',(-1.50305498755847,-0.718597038941581,
6.12120773806358));
#52295=CARTESIAN_POINT('Ctrl Pts',(-1.47654520160721,-0.774046287733134,
6.12532773042838));
#52296=CARTESIAN_POINT('Ctrl Pts',(-1.44692195174979,-0.8281124372478,6.12944772279318));
#52297=CARTESIAN_POINT('Ctrl Pts',(-1.41435640680187,-0.880427143231349,
6.13356771515798));
#52298=CARTESIAN_POINT('Ctrl Pts',(-1.38215784537766,-0.93215231094141,
6.13764127902548));
#52299=CARTESIAN_POINT('Ctrl Pts',(-1.34708323540234,-0.982164862027837,
6.14171484289298));
#52300=CARTESIAN_POINT('Ctrl Pts',(-1.30934474178789,-1.03013219887178,
6.14578840676048));
#52301=CARTESIAN_POINT('Ctrl Pts',(-1.27162823510276,-1.07807158933143,
6.14985959731754));
#52302=CARTESIAN_POINT('Ctrl Pts',(-1.23125123711747,-1.12396772848948,
6.1539307878746));
#52303=CARTESIAN_POINT('Ctrl Pts',(-1.18846814411064,-1.16751850967521,
6.15800197843166));
#52304=CARTESIAN_POINT('Ctrl Pts',(-1.1456942440287,-1.21105993298069,6.16207229420042));
#52305=CARTESIAN_POINT('Ctrl Pts',(-1.10051563268515,-1.25225663541508,
6.16614260996919));
#52306=CARTESIAN_POINT('Ctrl Pts',(-1.0532243429506,-1.29084254787959,6.17021292573795));
#52307=CARTESIAN_POINT('Ctrl Pts',(-1.00493497859783,-1.33024280945719,
6.17436914482802));
#52308=CARTESIAN_POINT('Ctrl Pts',(-0.954443134280577,-1.3669204304962,
6.17852536391809));
#52309=CARTESIAN_POINT('Ctrl Pts',(-0.902094275076489,-1.40063625501921,
6.18268158300815));
#52310=CARTESIAN_POINT('Ctrl Pts',(-0.85076001401308,-1.43369861710975,
6.18675724843908));
#52311=CARTESIAN_POINT('Ctrl Pts',(-0.797640573016811,-1.46391277769745,
6.19083291387));
#52312=CARTESIAN_POINT('Ctrl Pts',(-0.743087775427189,-1.49109911072694,
6.19490857930092));
#52313=CARTESIAN_POINT('Ctrl Pts',(-0.686917661277731,-1.5190914318735,
6.19910507522056));
#52314=CARTESIAN_POINT('Ctrl Pts',(-0.629228375774907,-1.54387328901976,
6.2033015711402));
#52315=CARTESIAN_POINT('Ctrl Pts',(-0.570424688362431,-1.56530242282654,
6.20749806705984));
#52316=CARTESIAN_POINT('Ctrl Pts',(-0.511621000949956,-1.58673155663331,
6.21169456297949));
#52317=CARTESIAN_POINT('Ctrl Pts',(-0.451703489315339,-1.60480786594618,
6.21589105889913));
#52318=CARTESIAN_POINT('Ctrl Pts',(-0.39108948985327,-1.619445896264,6.22008755481877));
#52319=CARTESIAN_POINT('Ctrl Pts',(-0.332275257023779,-1.63364929037952,
6.22415944729041));
#52320=CARTESIAN_POINT('Ctrl Pts',(-0.272561676081544,-1.64467460318456,
6.22823133976206));
#52321=CARTESIAN_POINT('Ctrl Pts',(-0.212324570981963,-1.65241468056821,
6.2323032322337));
#52322=CARTESIAN_POINT('Ctrl Pts',(-0.151352714266586,-1.66024916876981,
6.23642479225773));
#52323=CARTESIAN_POINT('Ctrl Pts',(-0.0898449686004922,-1.66471751880863,
6.24054635228175));
#52324=CARTESIAN_POINT('Ctrl Pts',(-0.0282053183113921,-1.66576122539185,
6.24466791230578));
#52325=CARTESIAN_POINT('Ctrl Pts',(0.0325208065838762,-1.66678946380704,
6.24872838908669));
#52326=CARTESIAN_POINT('Ctrl Pts',(0.0933744219731093,-1.66449386898338,
6.2527888658676));
#52327=CARTESIAN_POINT('Ctrl Pts',(0.153963202056404,-1.65887049898795,
6.25684934264851));
#52328=CARTESIAN_POINT('Ctrl Pts',(0.214514070017212,-1.65325064769502,
6.26090727867365));
#52329=CARTESIAN_POINT('Ctrl Pts',(0.274799920958721,-1.64430719665915,
6.26496521469878));
#52330=CARTESIAN_POINT('Ctrl Pts',(0.334430872690372,-1.63208823027174,
6.26902315072391));
#52331=CARTESIAN_POINT('Ctrl Pts',(0.394046829711921,-1.61987233644738,
6.27308006634651));
#52332=CARTESIAN_POINT('Ctrl Pts',(0.453007711537243,-1.60438266514088,
6.27713698196911));
#52333=CARTESIAN_POINT('Ctrl Pts',(0.510933284968012,-1.58571850538227,
6.28119389759171));
#52334=CARTESIAN_POINT('Ctrl Pts',(0.570457767584166,-1.56653916217863,
6.2853627955266));
#52335=CARTESIAN_POINT('Ctrl Pts',(0.628888381830324,-1.54400760526379,
6.28953169346148));
#52336=CARTESIAN_POINT('Ctrl Pts',(0.685831073304624,-1.51828578959622,
6.29370059139637));
#52337=CARTESIAN_POINT('Ctrl Pts',(0.741314463005289,-1.49322316109128,
6.2977626506836));
#52338=CARTESIAN_POINT('Ctrl Pts',(0.795384852046118,-1.46513215726107,
6.30182470997084));
#52339=CARTESIAN_POINT('Ctrl Pts',(0.847702110907871,-1.43420958411326,
6.30588676925808));
#52340=CARTESIAN_POINT('Ctrl Pts',(0.902083410982519,-1.40206704136509,
6.31010908651679));
#52341=CARTESIAN_POINT('Ctrl Pts',(0.954569835289881,-1.36686515395936,
6.3143314037755));
#52342=CARTESIAN_POINT('Ctrl Pts',(1.00481450032127,-1.32887313914614,6.31855372103421));
#52343=CARTESIAN_POINT('Ctrl Pts',(1.05505916535267,-1.29088112433292,6.32277603829291));
#52344=CARTESIAN_POINT('Ctrl Pts',(1.10306165111379,-1.25009943725184,6.32699835555162));
#52345=CARTESIAN_POINT('Ctrl Pts',(1.14851763589996,-1.20684018827133,6.33122067281033));
#52346=CARTESIAN_POINT('Ctrl Pts',(1.19242570771038,-1.16505404680642,6.33529920746917));
#52347=CARTESIAN_POINT('Ctrl Pts',(1.23414067015834,-1.12078260523448,6.339377742128));
#52348=CARTESIAN_POINT('Ctrl Pts',(1.27336854985667,-1.07428512799718,6.34345627678683));
#52349=CARTESIAN_POINT('Ctrl Pts',(1.31300226746573,-1.02730660413791,6.34757700653746));
#52350=CARTESIAN_POINT('Ctrl Pts',(1.35009670262528,-0.97805601886764,6.35169773628809));
#52351=CARTESIAN_POINT('Ctrl Pts',(1.3843850598368,-0.926840874206924,6.35581846603871));
#52352=CARTESIAN_POINT('Ctrl Pts',(1.41822892632856,-0.876289647516156,
6.35988577747824));
#52353=CARTESIAN_POINT('Ctrl Pts',(1.4493387417139,-0.823824930299692,6.36395308891776));
#52354=CARTESIAN_POINT('Ctrl Pts',(1.47749842961004,-0.769775545532505,
6.36802040035728));
#52355=CARTESIAN_POINT('Ctrl Pts',(1.5056408939184,-0.715759219523877,6.37208522406697));
#52356=CARTESIAN_POINT('Ctrl Pts',(1.53083657254523,-0.660160600538697,
6.37615004777666));
#52357=CARTESIAN_POINT('Ctrl Pts',(1.55291447988775,-0.603334582263409,
6.38021487148635));
#52358=CARTESIAN_POINT('Ctrl Pts',(1.57498707235554,-0.546522243870179,
6.38427871665997));
#52359=CARTESIAN_POINT('Ctrl Pts',(1.59394319832293,-0.488483569435168,
6.38834256183358));
#52360=CARTESIAN_POINT('Ctrl Pts',(1.60966015635893,-0.429593041180322,
6.3924064070072));
#52361=CARTESIAN_POINT('Ctrl Pts',(1.62575781964685,-0.369276032474007,
6.39656868899009));
#52362=CARTESIAN_POINT('Ctrl Pts',(1.63845714538738,-0.308065888929439,
6.40073097097298));
#52363=CARTESIAN_POINT('Ctrl Pts',(1.64768127900689,-0.246378576199764,
6.40489325295587));
#52364=CARTESIAN_POINT('Ctrl Pts',(1.65669871766469,-0.186073556622871,
6.40896226626437));
#52365=CARTESIAN_POINT('Ctrl Pts',(1.66239512475955,-0.125313062025278,
6.41303127957287));
#52366=CARTESIAN_POINT('Ctrl Pts',(1.66475131859362,-0.064490675611387,
6.41710029288137));
#52367=CARTESIAN_POINT('Ctrl Pts',(1.66718852435571,-0.0015770610825209,
6.42130920920146));
#52368=CARTESIAN_POINT('Ctrl Pts',(1.66605160417627,0.0614021824037467,
6.42551812552154));
#52369=CARTESIAN_POINT('Ctrl Pts',(1.66137784548386,0.124014735154304,6.42972704184163));
#52370=CARTESIAN_POINT('Ctrl Pts',(1.65670408679146,0.18662728790487,6.43393595816171));
#52371=CARTESIAN_POINT('Ctrl Pts',(1.64849363888062,0.248872566572567,6.4381448744818));
#52372=CARTESIAN_POINT('Ctrl Pts',(1.63684178780226,0.310330407315007,6.44235379080188));
#52373=CARTESIAN_POINT('Ctrl Pts',(1.62555182528446,0.369879462116787,6.44643198465922));
#52374=CARTESIAN_POINT('Ctrl Pts',(1.61098479711917,0.42893395946793,6.45051017851655));
#52375=CARTESIAN_POINT('Ctrl Pts',(1.59319910883432,0.487106353489169,6.45458837237389));
#52376=CARTESIAN_POINT('Ctrl Pts',(1.57522772858898,0.545886097966566,6.4587091447247));
#52377=CARTESIAN_POINT('Ctrl Pts',(1.55397010000998,0.60376467875591,6.46282991707552));
#52378=CARTESIAN_POINT('Ctrl Pts',(1.52953992863024,0.660351123816555,6.46695068942633));
#52379=CARTESIAN_POINT('Ctrl Pts',(1.50542850256665,0.71619927424801,6.47101769723881));
#52380=CARTESIAN_POINT('Ctrl Pts',(1.47822703288719,0.770788321482814,6.47508470505129));
#52381=CARTESIAN_POINT('Ctrl Pts',(1.44809461484857,0.823758451517545,6.47915171286377));
#52382=CARTESIAN_POINT('Ctrl Pts',(1.41798051848918,0.87669637365809,6.48321624777771));
#52383=CARTESIAN_POINT('Ctrl Pts',(1.38493925978072,0.928016886466262,6.48728078269165));
#52384=CARTESIAN_POINT('Ctrl Pts',(1.34917628873037,0.977383927598429,6.49134531760559));
#52385=CARTESIAN_POINT('Ctrl Pts',(1.31342179239797,1.02673927026884,6.49540888935048));
#52386=CARTESIAN_POINT('Ctrl Pts',(1.2749471641762,1.07414164602324,6.49947246109536));
#52387=CARTESIAN_POINT('Ctrl Pts',(1.23400049281121,1.11928494305145,6.50353603284025));
#52388=CARTESIAN_POINT('Ctrl Pts',(1.19205623312917,1.16552807125536,6.50769860583635));
#52389=CARTESIAN_POINT('Ctrl Pts',(1.14751823004332,1.20940014664625,6.51186117883245));
#52390=CARTESIAN_POINT('Ctrl Pts',(1.10069440802769,1.25061097873663,6.51602375182855));
#52391=CARTESIAN_POINT('Ctrl Pts',(1.05492562545604,1.29089324388173,6.52009253327773));
#52392=CARTESIAN_POINT('Ctrl Pts',(1.00697342147985,1.32863267997271,6.52416131472692));
#52393=CARTESIAN_POINT('Ctrl Pts',(0.957158064882367,1.36359980889946,6.5282300961761));
#52394=CARTESIAN_POINT('Ctrl Pts',(0.905620229670406,1.3997760053889,6.53243956494566));
#52395=CARTESIAN_POINT('Ctrl Pts',(0.852088517331065,1.43298430956935,6.53664903371522));
#52396=CARTESIAN_POINT('Ctrl Pts',(0.796946566940896,1.46302158884998,6.54085850248478));
#52397=CARTESIAN_POINT('Ctrl Pts',(0.741804616550727,1.4930588681306,6.54506797125434));
#52398=CARTESIAN_POINT('Ctrl Pts',(0.685052999916675,1.5199249316788,6.54927744002389));
#52399=CARTESIAN_POINT('Ctrl Pts',(0.627096590274101,1.54347201674232,6.55348690879345));
#52400=CARTESIAN_POINT('Ctrl Pts',(0.570970011416014,1.56627566063341,6.55756347396204));
#52401=CARTESIAN_POINT('Ctrl Pts',(0.513481638667367,1.58606110557588,6.56164003913063));
#52402=CARTESIAN_POINT('Ctrl Pts',(0.454988330986168,1.60266703300044,6.56571660429921));
#52403=CARTESIAN_POINT('Ctrl Pts',(0.39585778763514,1.61945386811691,6.56983758023612));
#52404=CARTESIAN_POINT('Ctrl Pts',(0.335700735833276,1.63299120758289,6.57395855617303));
#52405=CARTESIAN_POINT('Ctrl Pts',(0.274907480839262,1.64316215784645,6.57807953210994));
#52406=CARTESIAN_POINT('Ctrl Pts',(0.214935497216141,1.65319570618496,6.58214483674651));
#52407=CARTESIAN_POINT('Ctrl Pts',(0.154344913616217,1.65995316979927,6.58621014138308));
#52408=CARTESIAN_POINT('Ctrl Pts',(0.0935239959668483,1.66337285723267,
6.59027544601966));
#52409=CARTESIAN_POINT('Ctrl Pts',(0.0327404210518218,1.6667904450516,6.59433825464668));
#52410=CARTESIAN_POINT('Ctrl Pts',(-0.0282726972042708,1.66687429113425,
6.59840106327371));
#52411=CARTESIAN_POINT('Ctrl Pts',(-0.0891218696325091,1.66361452637118,
6.60246387190073));
#52412=CARTESIAN_POINT('Ctrl Pts',(-0.149956312603149,1.66035555068321,
6.60652569706381));
#52413=CARTESIAN_POINT('Ctrl Pts',(-0.210626377302139,1.65375459821952,
6.61058752222689));
#52414=CARTESIAN_POINT('Ctrl Pts',(-0.27074058094533,1.64385386754096,6.61464934738997));
#52415=CARTESIAN_POINT('Ctrl Pts',(-0.332370256373181,1.63370354064252,
6.61881357067289));
#52416=CARTESIAN_POINT('Ctrl Pts',(-0.393415100212304,1.62008483939551,
6.62297779395581));
#52417=CARTESIAN_POINT('Ctrl Pts',(-0.453463527979288,1.60309913255312,
6.62714201723873));
#52418=CARTESIAN_POINT('Ctrl Pts',(-0.512110054751508,1.58650997696453,
6.63120902184366));
#52419=CARTESIAN_POINT('Ctrl Pts',(-0.569805714942126,1.56670957536178,
6.63527602644859));
#52420=CARTESIAN_POINT('Ctrl Pts',(-0.626184237321801,1.54384238215231,
6.63934303105352));
#52421=CARTESIAN_POINT('Ctrl Pts',(-0.684584288791703,1.52015525442995,
6.64355586367544));
#52422=CARTESIAN_POINT('Ctrl Pts',(-0.741570391087137,1.49317744674347,
6.64776869629735));
#52423=CARTESIAN_POINT('Ctrl Pts',(-0.796762667802162,1.46312174858991,
6.65198152891926));
#52424=CARTESIAN_POINT('Ctrl Pts',(-0.851954944517186,1.43306605043634,
6.65619436154118));
#52425=CARTESIAN_POINT('Ctrl Pts',(-0.905352921888731,1.3999328414526,6.66040719416309));
#52426=CARTESIAN_POINT('Ctrl Pts',(-0.95661190713044,1.36398301277408,6.664620026785));
#52427=CARTESIAN_POINT('Ctrl Pts',(-1.00591490356432,1.32940499163734,6.66867210215785));
#52428=CARTESIAN_POINT('Ctrl Pts',(-1.05344849322557,1.29207460725326,6.67272417753069));
#52429=CARTESIAN_POINT('Ctrl Pts',(-1.09888593881631,1.25220034078888,6.67677625290353));
#52430=CARTESIAN_POINT('Ctrl Pts',(-1.1442566087339,1.21238467425129,6.68082237327478));
#52431=CARTESIAN_POINT('Ctrl Pts',(-1.18753685284736,1.17003287360593,6.68486849364603));
#52432=CARTESIAN_POINT('Ctrl Pts',(-1.22842991906173,1.12539590098506,6.68891461401728));
#52433=CARTESIAN_POINT('Ctrl Pts',(-1.2692780118434,1.08080801927545,6.6929562845407));
#52434=CARTESIAN_POINT('Ctrl Pts',(-1.30774378443032,1.03394033042938,6.69699795506411));
#52435=CARTESIAN_POINT('Ctrl Pts',(-1.34356618508168,0.985081674941245,
6.70103962558753));
#52436=CARTESIAN_POINT('Ctrl Pts',(-1.37936537676592,0.93625467447647,6.70507867755394));
#52437=CARTESIAN_POINT('Ctrl Pts',(-1.41252428754029,0.885439683712039,
6.70911772952034));
#52438=CARTESIAN_POINT('Ctrl Pts',(-1.44282250171624,0.832958119320112,
6.71315678148675));
#52439=CARTESIAN_POINT('Ctrl Pts',(-1.4731207834657,0.78047643787958,6.71719584246137));
#52440=CARTESIAN_POINT('Ctrl Pts',(-1.50055808611293,0.726328618815754,
6.72123490343599));
#52441=CARTESIAN_POINT('Ctrl Pts',(-1.52495866950945,0.670862919148136,
6.72527396441062));
#52442=CARTESIAN_POINT('Ctrl Pts',(-1.5387622099493,0.639485676401743,6.7275588827913));
#52443=CARTESIAN_POINT('Ctrl Pts',(-1.55159476705925,0.607687133252561,
6.72984380117199));
#52444=CARTESIAN_POINT('Ctrl Pts',(-1.56343130033213,0.575533291080356,
6.73212871955268));
#52445=CARTESIAN_POINT('Origin',(0.,0.,11.));
#52446=CARTESIAN_POINT('',(-1.56542652693575,0.576282819883045,7.43212287682542));
#52447=CARTESIAN_POINT('',(-1.56343130033213,0.575533291080368,7.23929268604744));
#52448=CARTESIAN_POINT('',(-1.56343130033213,0.575533291080363,11.));
#52449=CARTESIAN_POINT('',(-1.66599935370279,0.00146746784764705,6.57851963665102));
#52450=CARTESIAN_POINT('Ctrl Pts',(-1.56343130033213,0.575533291080367,
7.23929268604743));
#52451=CARTESIAN_POINT('Ctrl Pts',(-1.54138234413752,0.635429093440622,
7.23501522736555));
#52452=CARTESIAN_POINT('Ctrl Pts',(-1.51591964574246,0.693968813501019,
7.23073776868366));
#52453=CARTESIAN_POINT('Ctrl Pts',(-1.4872440411031,0.750773709051744,7.22646031000177));
#52454=CARTESIAN_POINT('Ctrl Pts',(-1.47831443503859,0.768462798651881,
7.22512830597023));
#52455=CARTESIAN_POINT('Ctrl Pts',(-1.46907359443735,0.78598386460582,7.22379630193869));
#52456=CARTESIAN_POINT('Ctrl Pts',(-1.45952843832683,0.803326046954314,
7.22246429790715));
#52457=CARTESIAN_POINT('Ctrl Pts',(-1.43031089589254,0.856410139325714,
7.21838705874379));
#52458=CARTESIAN_POINT('Ctrl Pts',(-1.3981331718646,0.908007795322158,7.21430981958043));
#52459=CARTESIAN_POINT('Ctrl Pts',(-1.36317088397108,0.957768834893627,
7.21023258041707));
#52460=CARTESIAN_POINT('Ctrl Pts',(-1.32783427608864,1.00806263570309,7.20611168872951));
#52461=CARTESIAN_POINT('Ctrl Pts',(-1.28965329993057,1.05647975370382,7.20199079704195));
#52462=CARTESIAN_POINT('Ctrl Pts',(-1.2488573994866,1.10268363357201,7.19786990535439));
#52463=CARTESIAN_POINT('Ctrl Pts',(-1.20860484307088,1.14827214273051,7.19380389814946));
#52464=CARTESIAN_POINT('Ctrl Pts',(-1.16580694026357,1.19170561312127,7.18973789094453));
#52465=CARTESIAN_POINT('Ctrl Pts',(-1.12072644732855,1.2326914578508,7.18567188373961));
#52466=CARTESIAN_POINT('Ctrl Pts',(-1.07567353141141,1.27365223037505,7.18160836382677));
#52467=CARTESIAN_POINT('Ctrl Pts',(-1.02834117191007,1.31216800219547,7.17754484391393));
#52468=CARTESIAN_POINT('Ctrl Pts',(-0.979028826309048,1.34798314427738,
7.17348132400109));
#52469=CARTESIAN_POINT('Ctrl Pts',(-0.929728323804896,1.38378968481759,
7.16941878000329));
#52470=CARTESIAN_POINT('Ctrl Pts',(-0.878449193254686,1.41689658243843,
7.1653562360055));
#52471=CARTESIAN_POINT('Ctrl Pts',(-0.825522135047476,1.44708990893678,
7.1612936920077));
#52472=CARTESIAN_POINT('Ctrl Pts',(-0.77127926023977,1.47803387001745,7.15713014933336));
#52473=CARTESIAN_POINT('Ctrl Pts',(-0.715305882186241,1.50591712507302,
7.15296660665902));
#52474=CARTESIAN_POINT('Ctrl Pts',(-0.657985199821807,1.53055920395634,
7.14880306398467));
#52475=CARTESIAN_POINT('Ctrl Pts',(-0.601983544797386,1.55463423488382,
7.14473533012475));
#52476=CARTESIAN_POINT('Ctrl Pts',(-0.544696453213824,1.57561556209212,
7.14066759626482));
#52477=CARTESIAN_POINT('Ctrl Pts',(-0.486499465941723,1.5933845328854,7.13659986240489));
#52478=CARTESIAN_POINT('Ctrl Pts',(-0.426246376471802,1.61178128222209,
7.13238841532334));
#52479=CARTESIAN_POINT('Ctrl Pts',(-0.365018465458375,1.62673425465843,
7.12817696824179));
#52480=CARTESIAN_POINT('Ctrl Pts',(-0.303244253389687,1.63816938159219,
7.12396552116024));
#52481=CARTESIAN_POINT('Ctrl Pts',(-0.241470041321007,1.64960450852595,
7.11975407407868));
#52482=CARTESIAN_POINT('Ctrl Pts',(-0.179150133517697,1.65752178616255,
7.11554262699714));
#52483=CARTESIAN_POINT('Ctrl Pts',(-0.11671604163373,1.66190654539458,7.11133117991559));
#52484=CARTESIAN_POINT('Ctrl Pts',(-0.0562682154602125,1.66615180877349,
7.10725371496907));
#52485=CARTESIAN_POINT('Ctrl Pts',(0.00453631480646224,1.6671035694609,
7.10317625002255));
#52486=CARTESIAN_POINT('Ctrl Pts',(0.065308063584061,1.66471945289016,7.09909878507604));
#52487=CARTESIAN_POINT('Ctrl Pts',(0.126726636767738,1.662309960963,7.09497792161137));
#52488=CARTESIAN_POINT('Ctrl Pts',(0.188111206837704,1.65649303449352,7.0908570581467));
#52489=CARTESIAN_POINT('Ctrl Pts',(0.24905461762166,1.64727890699824,7.08673619468204));
#52490=CARTESIAN_POINT('Ctrl Pts',(0.309190061268199,1.63818693729034,7.08266996423207));
#52491=CARTESIAN_POINT('Ctrl Pts',(0.368895450941059,1.62578737574579,7.07860373378211));
#52492=CARTESIAN_POINT('Ctrl Pts',(0.427782428687343,1.61014228989439,7.07453750333214));
#52493=CARTESIAN_POINT('Ctrl Pts',(0.486633363102706,1.59450678003124,7.07047376172598));
#52494=CARTESIAN_POINT('Ctrl Pts',(0.544666385047516,1.57562981571251,7.06641002011981));
#52495=CARTESIAN_POINT('Ctrl Pts',(0.601504280451816,1.55362434346213,7.06234627851365));
#52496=CARTESIAN_POINT('Ctrl Pts',(0.658328499581683,1.53162416614528,7.05828351472071));
#52497=CARTESIAN_POINT('Ctrl Pts',(0.713957685855581,1.50649716001936,7.05422075092777));
#52498=CARTESIAN_POINT('Ctrl Pts',(0.768032713517711,1.47840513762859,7.05015798713482));
#52499=CARTESIAN_POINT('Ctrl Pts',(0.823446229936901,1.44961776920179,7.04599466003392));
#52500=CARTESIAN_POINT('Ctrl Pts',(0.877227099802084,1.41771685332561,7.04183133293302));
#52501=CARTESIAN_POINT('Ctrl Pts',(0.929015940646776,1.38292638344352,7.03766800583213));
#52502=CARTESIAN_POINT('Ctrl Pts',(0.979618314271451,1.34893295306668,7.03360005933931));
#52503=CARTESIAN_POINT('Ctrl Pts',(1.02831859242541,1.3121813429381,7.02953211284648));
#52504=CARTESIAN_POINT('Ctrl Pts',(1.07481336684084,1.27292271032465,7.02546416635366));
#52505=CARTESIAN_POINT('Ctrl Pts',(1.12294337657611,1.23228333969353,7.02125314894873));
#52506=CARTESIAN_POINT('Ctrl Pts',(1.16870938909863,1.18895769286279,7.01704213154379));
#52507=CARTESIAN_POINT('Ctrl Pts',(1.21181684266056,1.14326547216479,7.01283111413885));
#52508=CARTESIAN_POINT('Ctrl Pts',(1.25492429622248,1.09757325146681,7.00862009673391));
#52509=CARTESIAN_POINT('Ctrl Pts',(1.29537285953596,1.04951496289525,7.00440907932897));
#52510=CARTESIAN_POINT('Ctrl Pts',(1.3329162180352,0.999445023850107,7.00019806192404));
#52511=CARTESIAN_POINT('Ctrl Pts',(1.369269928637,0.950961666296099,6.99612048031712));
#52512=CARTESIAN_POINT('Ctrl Pts',(1.40304988782896,0.90039221972186,6.99204289871021));
#52513=CARTESIAN_POINT('Ctrl Pts',(1.43400925267186,0.848040956116805,6.9879653171033));
#52514=CARTESIAN_POINT('Ctrl Pts',(1.46529712776615,0.795134192524742,6.98384446822118));
#52515=CARTESIAN_POINT('Ctrl Pts',(1.49370380886418,0.74040794320345,6.97972361933906));
#52516=CARTESIAN_POINT('Ctrl Pts',(1.5190170897545,0.684209822374529,6.97560277045694));
#52517=CARTESIAN_POINT('Ctrl Pts',(1.54399562256727,0.628754877153322,6.97153641653528));
#52518=CARTESIAN_POINT('Ctrl Pts',(1.56596185831363,0.571867233513525,6.96747006261362));
#52519=CARTESIAN_POINT('Ctrl Pts',(1.5847573135943,0.513906856355669,6.96340370869196));
#52520=CARTESIAN_POINT('Ctrl Pts',(1.60354127503716,0.455981923254109,6.95933984143592));
#52521=CARTESIAN_POINT('Ctrl Pts',(1.61915814293015,0.396986043224092,6.95527597417988));
#52522=CARTESIAN_POINT('Ctrl Pts',(1.63149822433278,0.33729741178813,6.95121210692384));
#52523=CARTESIAN_POINT('Ctrl Pts',(1.64383534250147,0.277623113432597,6.9471492155276));
#52524=CARTESIAN_POINT('Ctrl Pts',(1.65289713262305,0.217256894970195,6.94308632413137));
#52525=CARTESIAN_POINT('Ctrl Pts',(1.6586247670321,0.156588256864011,6.93902343273513));
#52526=CARTESIAN_POINT('Ctrl Pts',(1.66449382126762,0.0944216620691974,
6.93486022533491));
#52527=CARTESIAN_POINT('Ctrl Pts',(1.66686177525296,0.0319380680069127,
6.93069701793469));
#52528=CARTESIAN_POINT('Ctrl Pts',(1.66572190280597,-0.0304391608371186,
6.92653381053446));
#52529=CARTESIAN_POINT('Ctrl Pts',(1.66460807664504,-0.0913910590218248,
6.92246573315618));
#52530=CARTESIAN_POINT('Ctrl Pts',(1.660145155455,-0.152240882502124,6.91839765577791));
#52531=CARTESIAN_POINT('Ctrl Pts',(1.65237958996264,-0.212597485109536,
6.91432957839963));
#52532=CARTESIAN_POINT('Ctrl Pts',(1.64434163348051,-0.275071202657193,
6.91011880598843));
#52533=CARTESIAN_POINT('Ctrl Pts',(1.63276509875916,-0.337015858767348,
6.90590803357724));
#52534=CARTESIAN_POINT('Ctrl Pts',(1.61775879022358,-0.398010674045737,
6.90169726116605));
#52535=CARTESIAN_POINT('Ctrl Pts',(1.60275248168799,-0.459005489324134,
6.89748648875485));
#52536=CARTESIAN_POINT('Ctrl Pts',(1.58431664462742,-0.519049911293533,
6.89327571634366));
#52537=CARTESIAN_POINT('Ctrl Pts',(1.56261539719853,-0.577744857560916,
6.88906494393246));
#52538=CARTESIAN_POINT('Ctrl Pts',(1.54160607127545,-0.63456837704797,6.88498842758176));
#52539=CARTESIAN_POINT('Ctrl Pts',(1.5174496925766,-0.690362018593101,6.88091191123105));
#52540=CARTESIAN_POINT('Ctrl Pts',(1.49026783765061,-0.744753497517247,
6.87683539488034));
#52541=CARTESIAN_POINT('Ctrl Pts',(1.4627894893984,-0.799738265992379,6.87271441284119));
#52542=CARTESIAN_POINT('Ctrl Pts',(1.43221936086653,-0.853289571210904,
6.86859343080205));
#52543=CARTESIAN_POINT('Ctrl Pts',(1.39873439205661,-0.90504038610331,6.86447244876291));
#52544=CARTESIAN_POINT('Ctrl Pts',(1.36570199812458,-0.956091749284591,
6.86040716493731));
#52545=CARTESIAN_POINT('Ctrl Pts',(1.32983335510675,-1.0053905476909,6.8563418811117));
#52546=CARTESIAN_POINT('Ctrl Pts',(1.29134477954824,-1.05260850287916,6.8522765972861));
#52547=CARTESIAN_POINT('Ctrl Pts',(1.25287973596075,-1.09979758894101,6.84821379898094));
#52548=CARTESIAN_POINT('Ctrl Pts',(1.21179825868441,-1.14490795801612,6.84415100067577));
#52549=CARTESIAN_POINT('Ctrl Pts',(1.16835844803008,-1.18764242805516,6.84008820237061));
#52550=CARTESIAN_POINT('Ctrl Pts',(1.12492904067245,-1.23036666371784,6.83602637705533));
#52551=CARTESIAN_POINT('Ctrl Pts',(1.07914278607903,-1.27071577083916,6.83196455174004));
#52552=CARTESIAN_POINT('Ctrl Pts',(1.03129487317033,-1.30842916681515,6.82790272642476));
#52553=CARTESIAN_POINT('Ctrl Pts',(0.982240504983445,-1.34709348254642,
6.82373848471777));
#52554=CARTESIAN_POINT('Ctrl Pts',(0.931019507188232,-1.38298697528364,
6.81957424301078));
#52555=CARTESIAN_POINT('Ctrl Pts',(0.877984313423429,-1.41587412766192,
6.8154100013038));
#52556=CARTESIAN_POINT('Ctrl Pts',(0.826187186692727,-1.44799355400178,
6.81134297071293));
#52557=CARTESIAN_POINT('Ctrl Pts',(0.772660150675267,-1.47724530121765,
6.80727594012206));
#52558=CARTESIAN_POINT('Ctrl Pts',(0.717756886887557,-1.50345636828126,
6.80320890953119));
#52559=CARTESIAN_POINT('Ctrl Pts',(0.660885157127391,-1.53060718992515,
6.79899606226615));
#52560=CARTESIAN_POINT('Ctrl Pts',(0.602537179699622,-1.55449488489614,
6.7947832150011));
#52561=CARTESIAN_POINT('Ctrl Pts',(0.543126256529309,-1.57498249814671,
6.79057036773605));
#52562=CARTESIAN_POINT('Ctrl Pts',(0.483715333358995,-1.59547011139728,
6.786357520471));
#52563=CARTESIAN_POINT('Ctrl Pts',(0.423242064269878,-1.61255754928539,
6.78214467320596));
#52564=CARTESIAN_POINT('Ctrl Pts',(0.362131530765831,-1.62616627514692,
6.77793182594091));
#52565=CARTESIAN_POINT('Ctrl Pts',(0.30297272154368,-1.63934037085245,6.77385352694163));
#52566=CARTESIAN_POINT('Ctrl Pts',(0.242972147781927,-1.64930917517476,
6.76977522794235));
#52567=CARTESIAN_POINT('Ctrl Pts',(0.182508823830435,-1.65597298565648,
6.76569692894307));
#52568=CARTESIAN_POINT('Ctrl Pts',(0.121416000825612,-1.66270617476504,
6.761576169735));
#52569=CARTESIAN_POINT('Ctrl Pts',(0.0598512310689139,-1.66606495194213,
6.75745541052693));
#52570=CARTESIAN_POINT('Ctrl Pts',(-0.00178146810142189,-1.66599904753016,
6.75333465131886));
#52571=CARTESIAN_POINT('Ctrl Pts',(-0.0626108826772973,-1.66593400207779,
6.74926759967891));
#52572=CARTESIAN_POINT('Ctrl Pts',(-0.123505940107628,-1.66253301251172,
6.74520054803896));
#52573=CARTESIAN_POINT('Ctrl Pts',(-0.184073250022131,-1.65579981840387,
6.74113349639901));
#52574=CARTESIAN_POINT('Ctrl Pts',(-0.244603391048747,-1.64907075631603,
6.73706894062336));
#52575=CARTESIAN_POINT('Ctrl Pts',(-0.304805675828415,-1.63901360062296,
6.73300438484771));
#52576=CARTESIAN_POINT('Ctrl Pts',(-0.364290181355777,-1.62568406025518,
6.72893982907206));
#52577=CARTESIAN_POINT('Ctrl Pts',(-0.423760255386181,-1.61235775375847,
6.72487625939563));
#52578=CARTESIAN_POINT('Ctrl Pts',(-0.482512396761071,-1.5957607504669,
6.7208126897192));
#52579=CARTESIAN_POINT('Ctrl Pts',(-0.540167313231385,-1.57599976958005,
6.71674912004276));
#52580=CARTESIAN_POINT('Ctrl Pts',(-0.599226364472407,-1.55575752738775,
6.71258658570165));
#52581=CARTESIAN_POINT('Ctrl Pts',(-0.657133497568174,-1.53219530111909,
6.70842405136053));
#52582=CARTESIAN_POINT('Ctrl Pts',(-0.713500365734518,-1.50548106201862,
6.70426151701941));
#52583=CARTESIAN_POINT('Ctrl Pts',(-0.768596887935652,-1.47936888450076,
6.70019279414729));
#52584=CARTESIAN_POINT('Ctrl Pts',(-0.822221423291491,-1.45024560818,6.69612407127516));
#52585=CARTESIAN_POINT('Ctrl Pts',(-0.874036493550831,-1.41831456593429,
6.69205534840304));
#52586=CARTESIAN_POINT('Ctrl Pts',(-0.927643593401453,-1.38527918527316,
6.68784590832743));
#52587=CARTESIAN_POINT('Ctrl Pts',(-0.979313256794647,-1.34923856743358,
6.68363646825181));
#52588=CARTESIAN_POINT('Ctrl Pts',(-1.0287071089368,-1.31046468247828,6.6794270281762));
#52589=CARTESIAN_POINT('Ctrl Pts',(-1.07810096107896,-1.27169079752297,
6.67521758810058));
#52590=CARTESIAN_POINT('Ctrl Pts',(-1.12521860026201,-1.23018409495752,
6.67100814802497));
#52591=CARTESIAN_POINT('Ctrl Pts',(-1.16976409477779,-1.1862579662825,6.66679870794936));
#52592=CARTESIAN_POINT('Ctrl Pts',(-1.21228423010985,-1.14432903595683,
6.66278065935358));
#52593=CARTESIAN_POINT('Ctrl Pts',(-1.25264669484434,-1.10001260281998,
6.6587626107578));
#52594=CARTESIAN_POINT('Ctrl Pts',(-1.29056624785872,-1.05356288843517,
6.65474456216203));
#52595=CARTESIAN_POINT('Ctrl Pts',(-1.3284330151471,-1.00717783414526,6.6507321068709));
#52596=CARTESIAN_POINT('Ctrl Pts',(-1.36386327246504,-0.958665782258545,
6.64671965157978));
#52597=CARTESIAN_POINT('Ctrl Pts',(-1.39660808940078,-0.908318140642536,
6.64270719628865));
#52598=CARTESIAN_POINT('Ctrl Pts',(-1.42932031439161,-0.858020611615776,
6.63869873472032));
#52599=CARTESIAN_POINT('Ctrl Pts',(-1.45935210695291,-0.805891551873217,
6.63469027315199));
#52600=CARTESIAN_POINT('Ctrl Pts',(-1.48649583580301,-0.752254032983745,
6.63068181158365));
#52601=CARTESIAN_POINT('Ctrl Pts',(-1.513623308913,-0.69864863634145,6.62667575058858));
#52602=CARTESIAN_POINT('Ctrl Pts',(-1.53786590946504,-0.64353704156858,
6.6226696895935));
#52603=CARTESIAN_POINT('Ctrl Pts',(-1.55906143185519,-0.587267785342983,
6.61866362859842));
#52604=CARTESIAN_POINT('Ctrl Pts',(-1.5802611282017,-0.530987448219456,
6.61465677870447));
#52605=CARTESIAN_POINT('Ctrl Pts',(-1.59841235068726,-0.473549484378439,
6.61064992881052));
#52606=CARTESIAN_POINT('Ctrl Pts',(-1.61340136598415,-0.415321600979855,
6.60664307891656));
#52607=CARTESIAN_POINT('Ctrl Pts',(-1.62839221593782,-0.357086590483304,
6.60263573858384));
#52608=CARTESIAN_POINT('Ctrl Pts',(-1.64021997286835,-0.298061983443024,
6.59862839825111));
#52609=CARTESIAN_POINT('Ctrl Pts',(-1.64882174457498,-0.238627019879811,
6.59462105791838));
#52610=CARTESIAN_POINT('Ctrl Pts',(-1.6574325906907,-0.17912935560886,6.59060949005593));
#52611=CARTESIAN_POINT('Ctrl Pts',(-1.66281060799695,-0.11922099634073,
6.58659792219348));
#52612=CARTESIAN_POINT('Ctrl Pts',(-1.66494479657224,-0.0592859542136217,
6.58258635433103));
#52613=CARTESIAN_POINT('Ctrl Pts',(-1.66566597282296,-0.0390329505810895,
6.58123078177103));
#52614=CARTESIAN_POINT('Ctrl Pts',(-1.66601718561314,-0.018776894683292,
6.57987520921102));
#52615=CARTESIAN_POINT('Ctrl Pts',(-1.66599935370279,0.00146746784765552,
6.57851963665101));
#52616=CARTESIAN_POINT('Ctrl Pts',(-1.66599935370225,0.00146746846315725,
6.5785196366098));
#52617=CARTESIAN_POINT('Ctrl Pts',(-1.6659232556358,0.0878606910078806,
6.57273470356118));
#52618=CARTESIAN_POINT('Ctrl Pts',(-1.65912355325152,0.173965024338304,
6.56694977051255));
#52619=CARTESIAN_POINT('Ctrl Pts',(-1.64575458441607,0.258935991846446,
6.56116483746393));
#52620=CARTESIAN_POINT('Ctrl Pts',(-1.64151833437882,0.285860900468906,
6.55933175496188));
#52621=CARTESIAN_POINT('Ctrl Pts',(-1.63662281188489,0.312672235995731,
6.55749867245984));
#52622=CARTESIAN_POINT('Ctrl Pts',(-1.63107384411665,0.33934365330522,6.55566558995779));
#52623=CARTESIAN_POINT('Ctrl Pts',(-1.61875004980614,0.398578645220827,
6.55159446670515));
#52624=CARTESIAN_POINT('Ctrl Pts',(-1.60316934486775,0.457265793435973,
6.54752334345252));
#52625=CARTESIAN_POINT('Ctrl Pts',(-1.58439600177926,0.515019717628247,
6.54345222019989));
#52626=CARTESIAN_POINT('Ctrl Pts',(-1.57779998825323,0.535311557145502,
6.54202183116827));
#52627=CARTESIAN_POINT('Ctrl Pts',(-1.57081032106996,0.555488243876114,
6.54059144213665));
#52628=CARTESIAN_POINT('Ctrl Pts',(-1.56343130033213,0.575533291080354,
6.53916105310504));
#52629=CARTESIAN_POINT('',(-1.66802315249176,-0.000391568300512965,6.77148035500218));
#52630=CARTESIAN_POINT('Ctrl Pts',(-1.56343130033213,0.575533291080356,
6.73212871955268));
#52631=CARTESIAN_POINT('Ctrl Pts',(-1.58437359469063,0.518643726204979,
6.7361714094358));
#52632=CARTESIAN_POINT('Ctrl Pts',(-1.60219502983243,0.460641333802882,
6.74021409931893));
#52633=CARTESIAN_POINT('Ctrl Pts',(-1.61679613988877,0.401903274483785,
6.74425678920205));
#52634=CARTESIAN_POINT('Ctrl Pts',(-1.63140630364826,0.343128793484995,
6.74830198583391));
#52635=CARTESIAN_POINT('Ctrl Pts',(-1.64279207437441,0.283618247859168,
6.75234718246577));
#52636=CARTESIAN_POINT('Ctrl Pts',(-1.65090535474822,0.22375770302644,6.75639237909763));
#52637=CARTESIAN_POINT('Ctrl Pts',(-1.65903219328059,0.163797124825988,
6.76044433568537));
#52638=CARTESIAN_POINT('Ctrl Pts',(-1.66387559686924,0.103485897178399,
6.76449629227311));
#52639=CARTESIAN_POINT('Ctrl Pts',(-1.66543948648741,0.0432124617274922,
6.76854824886085));
#52640=CARTESIAN_POINT('Ctrl Pts',(-1.66581670718901,0.0286741034288136,
6.76952560806134));
#52641=CARTESIAN_POINT('Ctrl Pts',(-1.66600336108037,0.0141379256247708,
6.77050296726184));
#52642=CARTESIAN_POINT('Ctrl Pts',(-1.66599995419501,-0.000390668954461738,
6.77148032646233));
#52643=CARTESIAN_POINT('Ctrl Pts',(-1.66861778291936,-0.000391832623850849,
6.77148036339021));
#52644=CARTESIAN_POINT('Ctrl Pts',(-1.6686848074759,-0.0215969675807088,
6.77290462385233));
#52645=CARTESIAN_POINT('Ctrl Pts',(-1.6587079728118,-0.594273333106494,
6.81137325697827));
#52646=CARTESIAN_POINT('Ctrl Pts',(-1.00379156239439,-1.69403691970776,
6.88688626276814));
#52647=CARTESIAN_POINT('Ctrl Pts',(0.878789376459558,-1.76212723743541,
6.99801938075967));
#52648=CARTESIAN_POINT('Ctrl Pts',(1.95705435814059,-0.217444966801504,
7.10915249875125));
#52649=CARTESIAN_POINT('Ctrl Pts',(1.24415313987909,1.52624920138375,7.2202856167428));
#52650=CARTESIAN_POINT('Ctrl Pts',(-0.54953016239235,1.86221269474568,7.32794240943418));
#52651=CARTESIAN_POINT('Ctrl Pts',(-1.38933594127079,1.04443851451104,7.39855482946173));
#52652=CARTESIAN_POINT('Ctrl Pts',(-1.56542652693575,0.576282819883045,
7.43212287682542));
#52653=CARTESIAN_POINT('Origin',(0.,0.,11.));
#52654=CARTESIAN_POINT('',(-1.56343125288101,0.575533419980911,8.13202453882405));
#52655=CARTESIAN_POINT('',(-1.56343130037338,0.575533290968306,7.93773948050229));
#52656=CARTESIAN_POINT('',(-1.56343130033213,0.575533291080363,11.));
#52657=CARTESIAN_POINT('',(-1.66599999908997,-4.79547439094931E-5,7.2784065460554));
#52658=CARTESIAN_POINT('Ctrl Pts',(-1.56343130037338,0.575533290968306,
7.93773948050229));
#52659=CARTESIAN_POINT('Ctrl Pts',(-1.56203167958964,0.579335348948783,
7.93747628670542));
#52660=CARTESIAN_POINT('Ctrl Pts',(-1.56061816780054,0.583132360757538,
7.93721352742289));
#52661=CARTESIAN_POINT('Ctrl Pts',(-1.52941980829979,0.666012212448588,
7.93147968907109));
#52662=CARTESIAN_POINT('Ctrl Pts',(-1.49367280698885,0.742725695065311,
7.92621285832387));
#52663=CARTESIAN_POINT('Ctrl Pts',(-1.41856412868489,0.876332300525138,
7.91679788001118));
#52664=CARTESIAN_POINT('Ctrl Pts',(-1.38119752976503,0.934117609802933,
7.91263118292001));
#52665=CARTESIAN_POINT('Ctrl Pts',(-1.29770071258179,1.04722985814079,7.90398608123366));
#52666=CARTESIAN_POINT('Ctrl Pts',(-1.25134409869333,1.10220362883284,7.89951043725754));
#52667=CARTESIAN_POINT('Ctrl Pts',(-1.19356861801233,1.16236144131602,7.89405453492981));
#52668=CARTESIAN_POINT('Ctrl Pts',(-1.18545864918019,1.17063142740574,7.89329119735067));
#52669=CARTESIAN_POINT('Ctrl Pts',(-1.17271635867476,1.18335693629053,7.89209439707652));
#52670=CARTESIAN_POINT('Ctrl Pts',(-1.1681431862635,1.18787153745432,7.89166536779943));
#52671=CARTESIAN_POINT('Ctrl Pts',(-1.15965868270193,1.196150998751,7.89087004844909));
#52672=CARTESIAN_POINT('Ctrl Pts',(-1.15575492822701,1.19992333712037,7.89050434613051));
#52673=CARTESIAN_POINT('Ctrl Pts',(-1.14664122884843,1.20864449944749,7.88965114894849));
#52674=CARTESIAN_POINT('Ctrl Pts',(-1.14141765726347,1.21357874101211,7.88916258463778));
#52675=CARTESIAN_POINT('Ctrl Pts',(-1.12461588725819,1.22924543813192,7.88759300970436));
#52676=CARTESIAN_POINT('Ctrl Pts',(-1.1129173822338,1.23984680349988,7.88650303301046));
#52677=CARTESIAN_POINT('Ctrl Pts',(-1.04739204974372,1.2975522956479,7.88042200299868));
#52678=CARTESIAN_POINT('Ctrl Pts',(-0.990730009531427,1.34131431840367,
7.87525506931943));
#52679=CARTESIAN_POINT('Ctrl Pts',(-0.822406924389784,1.45481826894151,
7.86049590815139));
#52680=CARTESIAN_POINT('Ctrl Pts',(-0.705032198314378,1.515186711633,7.85091798884808));
#52681=CARTESIAN_POINT('Ctrl Pts',(-0.555783209276239,1.57080545575826,
7.83990310376356));
#52682=CARTESIAN_POINT('Ctrl Pts',(-0.52956327293834,1.57983785723202,7.83800631379048));
#52683=CARTESIAN_POINT('Ctrl Pts',(-0.491113492200113,1.59201833851759,
7.83527845449046));
#52684=CARTESIAN_POINT('Ctrl Pts',(-0.479055226254828,1.59568823952241,
7.83443050877856));
#52685=CARTESIAN_POINT('Ctrl Pts',(-0.457555813789876,1.60196584800041,
7.83293166317161));
#52686=CARTESIAN_POINT('Ctrl Pts',(-0.448131259840776,1.60462777050816,
7.83227902719695));
#52687=CARTESIAN_POINT('Ctrl Pts',(-0.428355727259881,1.61002546024071,
7.83091855409284));
#52688=CARTESIAN_POINT('Ctrl Pts',(-0.418000718261679,1.61274487141033,
7.83021127212468));
#52689=CARTESIAN_POINT('Ctrl Pts',(-0.390644924277279,1.61964781505652,
7.82835571014951));
#52690=CARTESIAN_POINT('Ctrl Pts',(-0.373602876372885,1.62366358286086,
7.82721283622368));
#52691=CARTESIAN_POINT('Ctrl Pts',(-0.28704871716064,1.64262412082784,7.82146955298152));
#52692=CARTESIAN_POINT('Ctrl Pts',(-0.216689840352994,1.65337784495494,
7.81700390013926));
#52693=CARTESIAN_POINT('Ctrl Pts',(-0.0773918888731418,1.66561984045195,
7.80836330926929));
#52694=CARTESIAN_POINT('Ctrl Pts',(-0.00862510000589039,1.66739460781424,
7.80419147471088));
#52695=CARTESIAN_POINT('Ctrl Pts',(0.0816869642174986,1.66413694338963,
7.79866064156089));
#52696=CARTESIAN_POINT('Ctrl Pts',(0.103300792882507,1.66293518957471,7.79733277290003));
#52697=CARTESIAN_POINT('Ctrl Pts',(0.18986870854935,1.65642767884693,7.79197795655623));
#52698=CARTESIAN_POINT('Ctrl Pts',(0.254502549675237,1.64773456119734,7.78789849265241));
#52699=CARTESIAN_POINT('Ctrl Pts',(0.329698051633503,1.63309107067683,7.78288596728083));
#52700=CARTESIAN_POINT('Ctrl Pts',(0.340919994515537,1.63078532917877,7.78213080168778));
#52701=CARTESIAN_POINT('Ctrl Pts',(0.35837035369613,1.6270118696835,7.78094412531749));
#52702=CARTESIAN_POINT('Ctrl Pts',(0.364615854345756,1.62562363720488,7.78051692974959));
#52703=CARTESIAN_POINT('Ctrl Pts',(0.376149827627841,1.62299008790842,7.77972313974866));
#52704=CARTESIAN_POINT('Ctrl Pts',(0.381440394439455,1.62175483369005,7.77935711257207));
#52705=CARTESIAN_POINT('Ctrl Pts',(0.393755361359132,1.61881591280597,7.7785006751061));
#52706=CARTESIAN_POINT('Ctrl Pts',(0.400774785914,1.61709239385297,7.77800916726913));
#52707=CARTESIAN_POINT('Ctrl Pts',(0.423317443318386,1.61140158034417,7.77642041243889));
#52708=CARTESIAN_POINT('Ctrl Pts',(0.438794194949957,1.60725614582408,7.77531390044416));
#52709=CARTESIAN_POINT('Ctrl Pts',(0.47585049621588,1.59675555828877,7.77263041949507));
#52710=CARTESIAN_POINT('Ctrl Pts',(0.497365469345877,1.59018536498431,7.77104429182738));
#52711=CARTESIAN_POINT('Ctrl Pts',(0.58192220943867,1.5624798083997,7.76471538870989));
#52712=CARTESIAN_POINT('Ctrl Pts',(0.643805522566909,1.53801500333623,7.75987442210042));
#52713=CARTESIAN_POINT('Ctrl Pts',(0.813236180856755,1.45901146271352,7.74626611905016));
#52714=CARTESIAN_POINT('Ctrl Pts',(0.916590094540017,1.39640257164126,7.7375695493467));
#52715=CARTESIAN_POINT('Ctrl Pts',(1.02899247990305,1.31040920176224,7.72783379107058));
#52716=CARTESIAN_POINT('Ctrl Pts',(1.04544377789134,1.29732231034052,7.72639991075937));
#52717=CARTESIAN_POINT('Ctrl Pts',(1.07133086541784,1.27591699551742,7.72412824001751));
#52718=CARTESIAN_POINT('Ctrl Pts',(1.0809273083582,1.26779737013674,7.72328262027302));
#52719=CARTESIAN_POINT('Ctrl Pts',(1.09783149118202,1.25316312828287,7.72178642395067));
#52720=CARTESIAN_POINT('Ctrl Pts',(1.10517534132402,1.24669133352132,7.72113413246839));
#52721=CARTESIAN_POINT('Ctrl Pts',(1.12044350104216,1.23299526774308,7.71977292720715));
#52722=CARTESIAN_POINT('Ctrl Pts',(1.12835598383182,1.22575843954846,7.7190645812382));
#52723=CARTESIAN_POINT('Ctrl Pts',(1.14905912024425,1.20645280386827,7.71720292230378));
#52724=CARTESIAN_POINT('Ctrl Pts',(1.16172972827058,1.19425680093639,7.71605508152727));
#52725=CARTESIAN_POINT('Ctrl Pts',(1.22554333447997,1.13085661772156,7.71022516209965));
#52726=CARTESIAN_POINT('Ctrl Pts',(1.27350709887378,1.0765568814807,7.7056831018695));
#52727=CARTESIAN_POINT('Ctrl Pts',(1.37964267794661,0.939341072402296,7.69497088398202));
#52728=CARTESIAN_POINT('Ctrl Pts',(1.4340842280218,0.853918438366526,7.6888979597863));
#52729=CARTESIAN_POINT('Ctrl Pts',(1.50505037886791,0.71641980291791,7.67928742194019));
#52730=CARTESIAN_POINT('Ctrl Pts',(1.5273352979142,0.667592407638185,7.67590022567893));
#52731=CARTESIAN_POINT('Ctrl Pts',(1.55135082598887,0.607445850336167,7.67165945351622));
#52732=CARTESIAN_POINT('Ctrl Pts',(1.55537371361498,0.597069879449797,7.67092546576335));
#52733=CARTESIAN_POINT('Ctrl Pts',(1.56151927727198,0.580735349026155,7.66976504207432));
#52734=CARTESIAN_POINT('Ctrl Pts',(1.56371256478532,0.574803453645227,7.66934262138998));
#52735=CARTESIAN_POINT('Ctrl Pts',(1.56756095812982,0.564210164745555,7.66858620995175));
#52736=CARTESIAN_POINT('Ctrl Pts',(1.5692291541367,0.559553685416715,7.66825299769306));
#52737=CARTESIAN_POINT('Ctrl Pts',(1.57322455731473,0.548242819132305,7.66744190969106));
#52738=CARTESIAN_POINT('Ctrl Pts',(1.57553027143562,0.54158107031377,7.66696280455243));
#52739=CARTESIAN_POINT('Ctrl Pts',(1.58262490038349,0.520654253127307,7.66545383506735));
#52740=CARTESIAN_POINT('Ctrl Pts',(1.58726271509061,0.506339274031315,7.66441591719923));
#52741=CARTESIAN_POINT('Ctrl Pts',(1.61071308974657,0.430467683600849,7.65889182748528));
#52742=CARTESIAN_POINT('Ctrl Pts',(1.626138663875,0.367927275960877,7.65426105383625));
#52743=CARTESIAN_POINT('Ctrl Pts',(1.65815475690377,0.195802136858974,7.64155515371738));
#52744=CARTESIAN_POINT('Ctrl Pts',(1.66750240072857,0.0851847124579617,
7.63345142371556));
#52745=CARTESIAN_POINT('Ctrl Pts',(1.66505605876994,-0.0743218353707407,
7.62219024586661));
#52746=CARTESIAN_POINT('Ctrl Pts',(1.66216627484113,-0.123042768685657,
7.61880338032627));
#52747=CARTESIAN_POINT('Ctrl Pts',(1.65548151757932,-0.18760835178785,7.61438435887574));
#52748=CARTESIAN_POINT('Ctrl Pts',(1.65358835242325,-0.203621072538078,
7.61329401414415));
#52749=CARTESIAN_POINT('Ctrl Pts',(1.65009072614499,-0.229923838817994,
7.61151166329134));
#52750=CARTESIAN_POINT('Ctrl Pts',(1.64862175570864,-0.240230496126132,
7.61081545119238));
#52751=CARTESIAN_POINT('Ctrl Pts',(1.64556620760834,-0.260319116061852,
7.60946251370362));
#52752=CARTESIAN_POINT('Ctrl Pts',(1.64398877706552,-0.270102006497136,
7.608805530402));
#52753=CARTESIAN_POINT('Ctrl Pts',(1.64004434347754,-0.293248569707283,
7.60725523623124));
#52754=CARTESIAN_POINT('Ctrl Pts',(1.63760112436008,-0.306598675356894,
7.60636437089141));
#52755=CARTESIAN_POINT('Ctrl Pts',(1.62871706348561,-0.352002201990275,
7.60334439516172));
#52756=CARTESIAN_POINT('Ctrl Pts',(1.62149578239099,-0.383896442527733,
7.60123994943381));
#52757=CARTESIAN_POINT('Ctrl Pts',(1.60144971967129,-0.461721960612977,
7.59612839119122));
#52758=CARTESIAN_POINT('Ctrl Pts',(1.58758293839445,-0.507355191672065,
7.59315215536533));
#52759=CARTESIAN_POINT('Ctrl Pts',(1.54918887881588,-0.616613273432739,
7.58599864896742));
#52760=CARTESIAN_POINT('Ctrl Pts',(1.52267861091282,-0.679446950595287,
7.5818625136953));
#52761=CARTESIAN_POINT('Ctrl Pts',(1.48307617590744,-0.759263229096041,
7.57640920392172));
#52762=CARTESIAN_POINT('Ctrl Pts',(1.47340367045259,-0.777867079452008,
7.5751230087387));
#52763=CARTESIAN_POINT('Ctrl Pts',(1.43199202029695,-0.853972038806598,
7.56978006534775));
#52764=CARTESIAN_POINT('Ctrl Pts',(1.39722107955565,-0.909747521852442,
7.56567027712554));
#52765=CARTESIAN_POINT('Ctrl Pts',(1.35262264314003,-0.972676483095749,
7.56062373859525));
#52766=CARTESIAN_POINT('Ctrl Pts',(1.34589433159103,-0.981965368933563,
7.55986771350742));
#52767=CARTESIAN_POINT('Ctrl Pts',(1.33526260974925,-0.996328628491809,
7.55867997023001));
#52768=CARTESIAN_POINT('Ctrl Pts',(1.3314247994995,-1.00145143307113,7.55825257955836));
#52769=CARTESIAN_POINT('Ctrl Pts',(1.32427542905052,-1.01088085395981,7.55745862984345));
#52770=CARTESIAN_POINT('Ctrl Pts',(1.32097220893052,-1.0151935445841,7.55709264025634));
#52771=CARTESIAN_POINT('Ctrl Pts',(1.31322769511709,-1.02520300355487,7.55623655680515));
#52772=CARTESIAN_POINT('Ctrl Pts',(1.30877040104304,-1.03088709867353,7.55574536843683));
#52773=CARTESIAN_POINT('Ctrl Pts',(1.29432353097421,-1.04906553567565,7.55415868224063));
#52774=CARTESIAN_POINT('Ctrl Pts',(1.28419125981278,-1.06144461102018,7.55305395168622));
#52775=CARTESIAN_POINT('Ctrl Pts',(1.25941632729917,-1.09083930834098,7.55037563659613));
#52776=CARTESIAN_POINT('Ctrl Pts',(1.24460515595084,-1.10770834873514,7.54879293679362));
#52777=CARTESIAN_POINT('Ctrl Pts',(1.18475603471489,-1.17315692544292,7.5424852571565));
#52778=CARTESIAN_POINT('Ctrl Pts',(1.13718010090682,-1.21932954753163,7.5376626606121));
#52779=CARTESIAN_POINT('Ctrl Pts',(0.995415658981791,-1.34138128937493,
7.52404543084659));
#52780=CARTESIAN_POINT('Ctrl Pts',(0.895525107244398,-1.41003580619472,
7.51532113868231));
#52781=CARTESIAN_POINT('Ctrl Pts',(0.770575909994075,-1.47723041668697,
7.50556181072833));
#52782=CARTESIAN_POINT('Ctrl Pts',(0.75189497190746,-1.48682579946201,7.5041293623527));
#52783=CARTESIAN_POINT('Ctrl Pts',(0.721754392967581,-1.50159396992655,
7.5018595108875));
#52784=CARTESIAN_POINT('Ctrl Pts',(0.710409497078258,-1.50699443123085,
7.5010142979853));
#52785=CARTESIAN_POINT('Ctrl Pts',(0.690120194140464,-1.51637261523005,
7.49951857380165));
#52786=CARTESIAN_POINT('Ctrl Pts',(0.681199897062275,-1.52040076882696,
7.49886635121487));
#52787=CARTESIAN_POINT('Ctrl Pts',(0.662431304005329,-1.52867779268205,
7.49750504386035));
#52788=CARTESIAN_POINT('Ctrl Pts',(0.652576405337925,-1.53291065318148,
7.49679652903752));
#52789=CARTESIAN_POINT('Ctrl Pts',(0.626445373352033,-1.54383673968681,
7.49493386521295));
#52790=CARTESIAN_POINT('Ctrl Pts',(0.610102604430971,-1.55036787089468,
7.49378519957891));
#52791=CARTESIAN_POINT('Ctrl Pts',(0.5258374232313,-1.58250427075608,7.48794043496538));
#52792=CARTESIAN_POINT('Ctrl Pts',(0.456393440769253,-1.60391137502625,
7.4833852717658));
#52793=CARTESIAN_POINT('Ctrl Pts',(0.286466541623964,-1.64435767834013,
7.47260009139512));
#52794=CARTESIAN_POINT('Ctrl Pts',(0.185208745897852,-1.65881631187453,
7.46647023069352));
#52795=CARTESIAN_POINT('Ctrl Pts',(0.0308040314928705,-1.66654328678569,
7.45686034967894));
#52796=CARTESIAN_POINT('Ctrl Pts',(-0.0217498511324031,-1.66668568808929,
7.45354073293712));
#52797=CARTESIAN_POINT('Ctrl Pts',(-0.0852748826907004,-1.66385297487849,
7.44937636382131));
#52798=CARTESIAN_POINT('Ctrl Pts',(-0.0963275598338264,-1.66324968440033,
7.4486462154374));
#52799=CARTESIAN_POINT('Ctrl Pts',(-0.113670902098468,-1.66212958416681,
7.44749055956977));
#52800=CARTESIAN_POINT('Ctrl Pts',(-0.119966275335952,-1.6616870698292,
7.44706901411883));
#52801=CARTESIAN_POINT('Ctrl Pts',(-0.131193345854335,-1.66083376527879,
7.44631331683516));
#52802=CARTESIAN_POINT('Ctrl Pts',(-0.136125941544077,-1.66043675444058,
7.44597993390369));
#52803=CARTESIAN_POINT('Ctrl Pts',(-0.148100824991372,-1.65941921293976,
7.44516729831359));
#52804=CARTESIAN_POINT('Ctrl Pts',(-0.155140955413846,-1.6587758311529,
7.44468680337489));
#52805=CARTESIAN_POINT('Ctrl Pts',(-0.177260090386513,-1.65661237110843,
7.44316897997566));
#52806=CARTESIAN_POINT('Ctrl Pts',(-0.192322080930886,-1.65493137762875,
7.44212346717845));
#52807=CARTESIAN_POINT('Ctrl Pts',(-0.272226218972042,-1.64490818447049,
7.43652062529918));
#52808=CARTESIAN_POINT('Ctrl Pts',(-0.336552692460002,-1.63296069560572,
7.43181442663552));
#52809=CARTESIAN_POINT('Ctrl Pts',(-0.510208695556801,-1.59000979200692,
7.4188280656632));
#52810=CARTESIAN_POINT('Ctrl Pts',(-0.617353601413024,-1.55155545277638,
7.41052315312256));
#52811=CARTESIAN_POINT('Ctrl Pts',(-0.760836352732686,-1.48282111383551,
7.39932123578709));
#52812=CARTESIAN_POINT('Ctrl Pts',(-0.801091048262076,-1.46146646465998,
7.39616476751244));
#52813=CARTESIAN_POINT('Ctrl Pts',(-0.854045407294286,-1.4305283428751,
7.3919920129286));
#52814=CARTESIAN_POINT('Ctrl Pts',(-0.867554072470824,-1.42237648271265,
7.39092558755175));
#52815=CARTESIAN_POINT('Ctrl Pts',(-0.889719375952903,-1.408567462375,7.38917196515257));
#52816=CARTESIAN_POINT('Ctrl Pts',(-0.898442532904366,-1.40301956058863,
7.38848082738135));
#52817=CARTESIAN_POINT('Ctrl Pts',(-0.914858132597249,-1.39236340369709,
7.38717807356309));
#52818=CARTESIAN_POINT('Ctrl Pts',(-0.922560809386965,-1.38727171439515,
7.38656587525558));
#52819=CARTESIAN_POINT('Ctrl Pts',(-0.938274947918068,-1.37669545434223,
7.38531484280078));
#52820=CARTESIAN_POINT('Ctrl Pts',(-0.946281605075904,-1.37120435473242,
7.38467628300811));
#52821=CARTESIAN_POINT('Ctrl Pts',(-0.973836879576364,-1.35195017596629,
7.38247419769189));
#52822=CARTESIAN_POINT('Ctrl Pts',(-0.993137540343235,-1.3378361131102,
7.38092398699142));
#52823=CARTESIAN_POINT('Ctrl Pts',(-1.03693124984591,-1.30434068666832,
7.37738209402012));
#52824=CARTESIAN_POINT('Ctrl Pts',(-1.06119673481312,-1.284676110951,7.3754012877494));
#52825=CARTESIAN_POINT('Ctrl Pts',(-1.14720843019216,-1.21087178791761,
7.36828392343225));
#52826=CARTESIAN_POINT('Ctrl Pts',(-1.2054854172128,-1.15286760463915,7.36328005521498));
#52827=CARTESIAN_POINT('Ctrl Pts',(-1.32204604946778,-1.01830696537451,
7.35240806219065));
#52828=CARTESIAN_POINT('Ctrl Pts',(-1.37845725767284,-0.94053472457296,
7.34655577552778));
#52829=CARTESIAN_POINT('Ctrl Pts',(-1.4358570166171,-0.845051238605321,
7.33932418678922));
#52830=CARTESIAN_POINT('Ctrl Pts',(-1.4436681553688,-0.831636448739964,
7.33830703240984));
#52831=CARTESIAN_POINT('Ctrl Pts',(-1.4547582326804,-0.811963272076779,
7.33681071336021));
#52832=CARTESIAN_POINT('Ctrl Pts',(-1.45818687081421,-0.805789622686513,
7.33634049867003));
#52833=CARTESIAN_POINT('Ctrl Pts',(-1.46420523223495,-0.794788680261306,
7.33550111699643));
#52834=CARTESIAN_POINT('Ctrl Pts',(-1.46681054641897,-0.789970143705068,
7.33513293935582));
#52835=CARTESIAN_POINT('Ctrl Pts',(-1.47243214868636,-0.779449279424317,
7.33432783787045));
#52836=CARTESIAN_POINT('Ctrl Pts',(-1.47543905303211,-0.773742340152184,
7.33389037737111));
#52837=CARTESIAN_POINT('Ctrl Pts',(-1.48395726036867,-0.757345039123737,
7.33263164860389));
#52838=CARTESIAN_POINT('Ctrl Pts',(-1.48938590554173,-0.746612524929958,
7.33180558737968));
#52839=CARTESIAN_POINT('Ctrl Pts',(-1.50152197018099,-0.7219601857328,7.32990474100212));
#52840=CARTESIAN_POINT('Ctrl Pts',(-1.50815281999854,-0.708004075085849,
7.32882619685348));
#52841=CARTESIAN_POINT('Ctrl Pts',(-1.52969675251713,-0.660983688600064,
7.32518897326475));
#52842=CARTESIAN_POINT('Ctrl Pts',(-1.54372337272971,-0.62752642248085,
7.32259547314784));
#52843=CARTESIAN_POINT('Ctrl Pts',(-1.5975735351535,-0.486320312482772,
7.3116959148403));
#52844=CARTESIAN_POINT('Ctrl Pts',(-1.62729684335138,-0.375043273491927,
7.30324382829815));
#52845=CARTESIAN_POINT('Ctrl Pts',(-1.65472558481929,-0.202525010328851,
7.29081226443812));
#52846=CARTESIAN_POINT('Ctrl Pts',(-1.66093006189091,-0.142989399614902,
7.28663378098082));
#52847=CARTESIAN_POINT('Ctrl Pts',(-1.66470165887666,-0.0675995426412908,
7.28148533229496));
#52848=CARTESIAN_POINT('Ctrl Pts',(-1.66526362916107,-0.0519459883801228,
7.28042390530268));
#52849=CARTESIAN_POINT('Ctrl Pts',(-1.66576334716281,-0.0290080946149532,
7.27887919665032));
#52850=CARTESIAN_POINT('Ctrl Pts',(-1.66587420348213,-0.0217287688149204,
7.27839055247581));
#52851=CARTESIAN_POINT('Ctrl Pts',(-1.6659786942146,-0.0096810953192746,
7.27758434923517));
#52852=CARTESIAN_POINT('Ctrl Pts',(-1.6659995782681,-0.0049131518317435,
7.2772659444449));
#52853=CARTESIAN_POINT('Ctrl Pts',(-1.66599999367699,-0.000145149081000685,
7.2769481782774));
#52854=CARTESIAN_POINT('Ctrl Pts',(-1.66599999950973,-4.04177140652074E-5,
7.2785196366098));
#52855=CARTESIAN_POINT('Ctrl Pts',(-1.66600154979607,0.0638616881954464,
7.27426975137157));
#52856=CARTESIAN_POINT('Ctrl Pts',(-1.66232218862922,0.12769579053969,7.27001986613334));
#52857=CARTESIAN_POINT('Ctrl Pts',(-1.6550110968451,0.191034733280547,7.26576998089511));
#52858=CARTESIAN_POINT('Ctrl Pts',(-1.64741960037028,0.256802935176299,
7.2613570984205));
#52859=CARTESIAN_POINT('Ctrl Pts',(-1.63591224260331,0.322036701043425,
7.25694421594588));
#52860=CARTESIAN_POINT('Ctrl Pts',(-1.62060186852973,0.38627138609784,7.25253133347127));
#52861=CARTESIAN_POINT('Ctrl Pts',(-1.60529149445616,0.450506071152247,
7.24811845099666));
#52862=CARTESIAN_POINT('Ctrl Pts',(-1.58617832364918,0.513741195306885,
7.24370556852205));
#52863=CARTESIAN_POINT('Ctrl Pts',(-1.56343130033213,0.575533291080367,
7.23929268604743));
#52864=CARTESIAN_POINT('',(-1.66554611378498,0.00151667131590039,7.47148008516546));
#52865=CARTESIAN_POINT('Ctrl Pts',(-1.56542652693575,0.576282819883045,
7.43212287682542));
#52866=CARTESIAN_POINT('Ctrl Pts',(-1.58366256406465,0.527800360715211,
7.43559920212559));
#52867=CARTESIAN_POINT('Ctrl Pts',(-1.64345104496323,0.34162213868473,7.44871827157227));
#52868=CARTESIAN_POINT('Ctrl Pts',(-1.66683094149558,0.145771637880644,
7.46183734101896));
#52869=CARTESIAN_POINT('Ctrl Pts',(-1.66554611378498,0.00151667131590039,
7.47148008516546));
#52870=CARTESIAN_POINT('Ctrl Pts',(-1.66599929579717,0.00153179741720764,
7.47174074231814));
#52871=CARTESIAN_POINT('Ctrl Pts',(-1.66606511006422,-0.0700485051244551,
7.47693011686521));
#52872=CARTESIAN_POINT('Ctrl Pts',(-1.66151769774625,-0.141566932664853,
7.48206009460744));
#52873=CARTESIAN_POINT('Ctrl Pts',(-1.64823818144976,-0.2447886730157,7.48933257774257));
#52874=CARTESIAN_POINT('Ctrl Pts',(-1.64315337568767,-0.27687150814081,
7.49157503229734));
#52875=CARTESIAN_POINT('Ctrl Pts',(-1.63482770468238,-0.321012704599486,
7.49463648679051));
#52876=CARTESIAN_POINT('Ctrl Pts',(-1.63238487073116,-0.333212288034103,
7.495480086183));
#52877=CARTESIAN_POINT('Ctrl Pts',(-1.62782711951716,-0.354719525273596,
7.49696311147657));
#52878=CARTESIAN_POINT('Ctrl Pts',(-1.62576847419785,-0.364038387434114,
7.49760429138865));
#52879=CARTESIAN_POINT('Ctrl Pts',(-1.62143651622804,-0.382877812467173,
7.49889786597761));
#52880=CARTESIAN_POINT('Ctrl Pts',(-1.61915914774067,-0.392397065168229,
7.49955010240221));
#52881=CARTESIAN_POINT('Ctrl Pts',(-1.61421016497247,-0.412306464290104,
7.5009115777872));
#52882=CARTESIAN_POINT('Ctrl Pts',(-1.61152181008147,-0.422692017796528,
7.50162024551048));
#52883=CARTESIAN_POINT('Ctrl Pts',(-1.60415669725266,-0.45005253573993,
7.5034836324523));
#52884=CARTESIAN_POINT('Ctrl Pts',(-1.59931075845737,-0.466980867530226,
7.50463286115424));
#52885=CARTESIAN_POINT('Ctrl Pts',(-1.57534973076255,-0.545931375598749,
7.50997990966618));
#52886=CARTESIAN_POINT('Ctrl Pts',(-1.5528884182984,-0.606882888538146,
7.51406792988093));
#52887=CARTESIAN_POINT('Ctrl Pts',(-1.48857539560215,-0.754249346768935,
7.52403223824845));
#52888=CARTESIAN_POINT('Ctrl Pts',(-1.44271212550968,-0.838647834028354,
7.52980624492016));
#52889=CARTESIAN_POINT('Ctrl Pts',(-1.35609292016508,-0.969698368615669,
7.53949342533846));
#52890=CARTESIAN_POINT('Ctrl Pts',(-1.31955528573769,-1.01885973066696,
7.54332040886845));
#52891=CARTESIAN_POINT('Ctrl Pts',(-1.27144415378068,-1.07665302696314,
7.54821253474785));
#52892=CARTESIAN_POINT('Ctrl Pts',(-1.26235269870898,-1.08729830740719,
7.54913118695542));
#52893=CARTESIAN_POINT('Ctrl Pts',(-1.24849314072053,-1.10311847086727,
7.55052528639408));
#52894=CARTESIAN_POINT('Ctrl Pts',(-1.24382437297918,-1.10838008278235,
7.55099385483223));
#52895=CARTESIAN_POINT('Ctrl Pts',(-1.23581725166109,-1.117289654297,7.55179601271377));
#52896=CARTESIAN_POINT('Ctrl Pts',(-1.23249575323544,-1.12095257189561,
7.55212835212134));
#52897=CARTESIAN_POINT('Ctrl Pts',(-1.22488155081081,-1.1292746874441,7.55288935121086));
#52898=CARTESIAN_POINT('Ctrl Pts',(-1.22057864391408,-1.13392411734268,
7.55331876327008));
#52899=CARTESIAN_POINT('Ctrl Pts',(-1.20861243642717,-1.14670696241178,
7.55451089892751));
#52900=CARTESIAN_POINT('Ctrl Pts',(-1.20089382329424,-1.15478781055824,
7.55527758177055));
#52901=CARTESIAN_POINT('Ctrl Pts',(-1.15487091837059,-1.20201016484932,
7.55983240784822));
#52902=CARTESIAN_POINT('Ctrl Pts',(-1.11474024097672,-1.23931763818206,
7.56373630352562));
#52903=CARTESIAN_POINT('Ctrl Pts',(-0.997439410417934,-1.33805329595476,
7.57480339429999));
#52904=CARTESIAN_POINT('Ctrl Pts',(-0.916538433098431,-1.39471535802987,
7.58204266147443));
#52905=CARTESIAN_POINT('Ctrl Pts',(-0.788758415227319,-1.46826538871721,
7.59261552521869));
#52906=CARTESIAN_POINT('Ctrl Pts',(-0.745359576585088,-1.49076588542471,
7.59607547705864));
#52907=CARTESIAN_POINT('Ctrl Pts',(-0.670850722051404,-1.52532689174123,
7.60178956246781));
#52908=CARTESIAN_POINT('Ctrl Pts',(-0.640256278989966,-1.53841963994834,
7.60407507782804));
#52909=CARTESIAN_POINT('Ctrl Pts',(-0.596573425602765,-1.5555843844099,
7.60725573063867));
#52910=CARTESIAN_POINT('Ctrl Pts',(-0.583797286906614,-1.56042410141119,
7.60817627107882));
#52911=CARTESIAN_POINT('Ctrl Pts',(-0.561639111401972,-1.56850757324789,
7.60975650491541));
#52912=CARTESIAN_POINT('Ctrl Pts',(-0.552285121072503,-1.57182557911951,
7.61041863758606));
#52913=CARTESIAN_POINT('Ctrl Pts',(-0.533086408394691,-1.57844311608841,
7.61176776878495));
#52914=CARTESIAN_POINT('Ctrl Pts',(-0.5232393606658,-1.58173460771746,7.61245447729455));
#52915=CARTESIAN_POINT('Ctrl Pts',(-0.498152223758011,-1.58986036152993,
7.61419107243432));
#52916=CARTESIAN_POINT('Ctrl Pts',(-0.482871911270453,-1.59456776387087,
7.61523678324587));
#52917=CARTESIAN_POINT('Ctrl Pts',(-0.421930410728298,-1.61238561757823,
7.61936256625576));
#52918=CARTESIAN_POINT('Ctrl Pts',(-0.375782985554731,-1.62376120063554,
7.62238689377845));
#52919=CARTESIAN_POINT('Ctrl Pts',(-0.219578268366115,-1.65524881249659,
7.63238012978473));
#52920=CARTESIAN_POINT('Ctrl Pts',(-0.108003527894205,-1.66625294721515,
7.63910055494325));
#52921=CARTESIAN_POINT('Ctrl Pts',(0.068598553793225,-1.66584655313675,
7.64996751217847));
#52922=CARTESIAN_POINT('Ctrl Pts',(0.133292675444497,-1.66192108996138,
7.65400312423229));
#52923=CARTESIAN_POINT('Ctrl Pts',(0.212570255889303,-1.65245199854183,
7.65918983361039));
#52924=CARTESIAN_POINT('Ctrl Pts',(0.227528534815957,-1.65045885981114,
7.66017923108757));
#52925=CARTESIAN_POINT('Ctrl Pts',(0.249439629064571,-1.64723577037253,
7.66164706266171));
#52926=CARTESIAN_POINT('Ctrl Pts',(0.256415476590733,-1.64616430243042,
7.6621171474832));
#52927=CARTESIAN_POINT('Ctrl Pts',(0.26826948284579,-1.64426639048574,7.66292100090787));
#52928=CARTESIAN_POINT('Ctrl Pts',(0.273151108871079,-1.64346248790184,
7.66325350468476));
#52929=CARTESIAN_POINT('Ctrl Pts',(0.28426016300007,-1.64158219318261,7.66401360070536));
#52930=CARTESIAN_POINT('Ctrl Pts',(0.290484951880989,-1.64049212940773,
7.66444193424402));
#52931=CARTESIAN_POINT('Ctrl Pts',(0.3076318398711,-1.63738877399296,7.6656282419087));
#52932=CARTESIAN_POINT('Ctrl Pts',(0.31854000686592,-1.63530168272758,7.66639011512619));
#52933=CARTESIAN_POINT('Ctrl Pts',(0.381434247155825,-1.62261480967266,
7.6708214168247));
#52934=CARTESIAN_POINT('Ctrl Pts',(0.432906395382925,-1.609646479883,7.67459951834391));
#52935=CARTESIAN_POINT('Ctrl Pts',(0.580896059449537,-1.56474901394487,
7.68575316171334));
#52936=CARTESIAN_POINT('Ctrl Pts',(0.675230307468231,-1.52641591423025,
7.69322004956054));
#52937=CARTESIAN_POINT('Ctrl Pts',(0.829844510994807,-1.4464318111034,7.70569617432575));
#52938=CARTESIAN_POINT('Ctrl Pts',(0.891971775772876,-1.40896978086581,
7.71078730172887));
#52939=CARTESIAN_POINT('Ctrl Pts',(0.96590976818101,-1.35752855430949,7.71693396908457));
#52940=CARTESIAN_POINT('Ctrl Pts',(0.980190480101765,-1.34725354701966,
7.71812579945101));
#52941=CARTESIAN_POINT('Ctrl Pts',(1.00291102710601,-1.33035351654904,7.72003022192212));
#52942=CARTESIAN_POINT('Ctrl Pts',(1.0114539635248,-1.32387004507877,7.72074821123819));
#52943=CARTESIAN_POINT('Ctrl Pts',(1.02767359117478,-1.31131186363387,7.72211535666721));
#52944=CARTESIAN_POINT('Ctrl Pts',(1.03536048002467,-1.30525112414625,7.72276502356839));
#52945=CARTESIAN_POINT('Ctrl Pts',(1.05279423744326,-1.29125452799047,7.72424275283952));
#52946=CARTESIAN_POINT('Ctrl Pts',(1.06250568992183,-1.28327535460166,7.72506903919155));
#52947=CARTESIAN_POINT('Ctrl Pts',(1.08820921005548,-1.26166486225525,7.72726524559726));
#52948=CARTESIAN_POINT('Ctrl Pts',(1.10403556524397,-1.24783935000791,7.72862725978399));
#52949=CARTESIAN_POINT('Ctrl Pts',(1.20891877081953,-1.15265801280928,7.73773260738465));
#52950=CARTESIAN_POINT('Ctrl Pts',(1.28917566899573,-1.06213701075134,7.74505952567361));
#52951=CARTESIAN_POINT('Ctrl Pts',(1.39736577450619,-0.909578346912501,
7.75648755336661));
#52952=CARTESIAN_POINT('Ctrl Pts',(1.43249730270166,-0.853178810569795,
7.76055511720956));
#52953=CARTESIAN_POINT('Ctrl Pts',(1.47489113962575,-0.775085353679222,
7.76617887338437));
#52954=CARTESIAN_POINT('Ctrl Pts',(1.48521302963107,-0.755118093401091,
7.76761627428513));
#52955=CARTESIAN_POINT('Ctrl Pts',(1.5021911859108,-0.720578963195752,7.77011222299979));
#52956=CARTESIAN_POINT('Ctrl Pts',(1.50904719011356,-0.706108301199287,
7.77116074308462));
#52957=CARTESIAN_POINT('Ctrl Pts',(1.51869291824966,-0.684967183717754,
7.77269986958501));
#52958=CARTESIAN_POINT('Ctrl Pts',(1.52164970748667,-0.678373337915016,
7.77318093290749));
#52959=CARTESIAN_POINT('Ctrl Pts',(1.5267541726125,-0.666788733680777,7.77402823585026));
#52960=CARTESIAN_POINT('Ctrl Pts',(1.52892047576051,-0.661806389022384,
7.77439334468097));
#52961=CARTESIAN_POINT('Ctrl Pts',(1.53358546406429,-0.650932085669827,
7.77519183288542));
#52962=CARTESIAN_POINT('Ctrl Pts',(1.53607454376806,-0.645036392993356,
7.7756257416792));
#52963=CARTESIAN_POINT('Ctrl Pts',(1.54292705929785,-0.628540761202718,
7.77684225581128));
#52964=CARTESIAN_POINT('Ctrl Pts',(1.54721505556059,-0.617910149206278,
7.77762907620787));
#52965=CARTESIAN_POINT('Ctrl Pts',(1.57523461865982,-0.54632461459301,7.78294241944471));
#52966=CARTESIAN_POINT('Ctrl Pts',(1.59546577626695,-0.48406790667297,7.78763367454426));
#52967=CARTESIAN_POINT('Ctrl Pts',(1.61771076303218,-0.398850927820837,
7.79401726211858));
#52968=CARTESIAN_POINT('Ctrl Pts',(1.62298943890232,-0.376796277985399,
7.79566628882188));
#52969=CARTESIAN_POINT('Ctrl Pts',(1.64308349721544,-0.284563756947635,
7.80253647332678));
#52970=CARTESIAN_POINT('Ctrl Pts',(1.65381047470781,-0.213569617150863,
7.80775806731946));
#52971=CARTESIAN_POINT('Ctrl Pts',(1.66374192572034,-0.0975577914778334,
7.81607844163075));
#52972=CARTESIAN_POINT('Ctrl Pts',(1.66576093713112,-0.0528753081618404,
7.81923371606509));
#52973=CARTESIAN_POINT('Ctrl Pts',(1.66613298995081,0.0230628265894545,
7.82450558909996));
#52974=CARTESIAN_POINT('Ctrl Pts',(1.6654080870238,0.054287794878682,7.82664754018315));
#52975=CARTESIAN_POINT('Ctrl Pts',(1.66312159779956,0.0987948085461002,
7.82966563439978));
#52976=CARTESIAN_POINT('Ctrl Pts',(1.66227743114115,0.112105410858295,7.83056380139308));
#52977=CARTESIAN_POINT('Ctrl Pts',(1.66053052740909,0.135247150480129,7.83211799397676));
#52978=CARTESIAN_POINT('Ctrl Pts',(1.65970008871767,0.1450828966386,7.83277624422192));
#52979=CARTESIAN_POINT('Ctrl Pts',(1.65780669637593,0.165357301616044,7.83412855316087));
#52980=CARTESIAN_POINT('Ctrl Pts',(1.65673244299333,0.175794483970449,7.83482222713154));
#52981=CARTESIAN_POINT('Ctrl Pts',(1.65371464562638,0.202623589199555,7.83659935453581));
#52982=CARTESIAN_POINT('Ctrl Pts',(1.65162593555921,0.218998285259902,7.83767822574861));
#52983=CARTESIAN_POINT('Ctrl Pts',(1.64190307290537,0.287137484126922,7.8421468546488));
#52984=CARTESIAN_POINT('Ctrl Pts',(1.63207552142209,0.338561595253835,7.84546780095202));
#52985=CARTESIAN_POINT('Ctrl Pts',(1.59467024787864,0.494144848548483,7.85546623960446));
#52986=CARTESIAN_POINT('Ctrl Pts',(1.55940633075307,0.596157978015871,7.86193909882742));
#52987=CARTESIAN_POINT('Ctrl Pts',(1.48818739189425,0.751569623524272,7.87246651426145));
#52988=CARTESIAN_POINT('Ctrl Pts',(1.45857869869201,0.807530210017678,7.87641345202993));
#52989=CARTESIAN_POINT('Ctrl Pts',(1.41814319337051,0.874441957315413,7.88149384781326));
#52990=CARTESIAN_POINT('Ctrl Pts',(1.41025114293976,0.887113594496471,7.88247283845108));
#52991=CARTESIAN_POINT('Ctrl Pts',(1.39839527008229,0.905591548686593,7.88392808775406));
#52992=CARTESIAN_POINT('Ctrl Pts',(1.39456301548982,0.911481966806043,7.88439619942984));
#52993=CARTESIAN_POINT('Ctrl Pts',(1.38797138181079,0.921474843121538,7.88519784878901));
#52994=CARTESIAN_POINT('Ctrl Pts',(1.38523082334428,0.925589546375507,7.88553014090408));
#52995=CARTESIAN_POINT('Ctrl Pts',(1.37893404613295,0.934952988206817,7.88629142174874));
#52996=CARTESIAN_POINT('Ctrl Pts',(1.37536623627921,0.940193547355703,7.88672116625208));
#52997=CARTESIAN_POINT('Ctrl Pts',(1.36541516301137,0.954632277652354,7.88791509622616));
#52998=CARTESIAN_POINT('Ctrl Pts',(1.35896909261153,0.963786460406188,7.88868325951374));
#52999=CARTESIAN_POINT('Ctrl Pts',(1.3201883176416,1.01769714643317,7.8932707835948));
#53000=CARTESIAN_POINT('Ctrl Pts',(1.28574005451607,1.06088449037299,7.89720777732692));
#53001=CARTESIAN_POINT('Ctrl Pts',(1.18415309445877,1.17601344225458,7.90829282629937));
#53002=CARTESIAN_POINT('Ctrl Pts',(1.11268486692914,1.24384894619304,7.91551426822696));
#53003=CARTESIAN_POINT('Ctrl Pts',(0.978225838533326,1.35055717992816,7.92782250416336));
#53004=CARTESIAN_POINT('Ctrl Pts',(0.917849439885174,1.39229507478499,7.9329753580091));
#53005=CARTESIAN_POINT('Ctrl Pts',(0.839769310743625,1.43897697519207,7.9391838343735));
#53006=CARTESIAN_POINT('Ctrl Pts',(0.824484136871119,1.44778906613068,7.9403791481222));
#53007=CARTESIAN_POINT('Ctrl Pts',(0.799677254216944,1.46157022684732,7.94228775891121));
#53008=CARTESIAN_POINT('Ctrl Pts',(0.790242805539901,1.46669272737715,7.94300649599863));
#53009=CARTESIAN_POINT('Ctrl Pts',(0.772114941154748,1.47630968064932,7.94437420442719));
#53010=CARTESIAN_POINT('Ctrl Pts',(0.763430183813212,1.48081940726994,7.94502369469331));
#53011=CARTESIAN_POINT('Ctrl Pts',(0.743520514111501,1.49093617094463,7.94649985042159));
#53012=CARTESIAN_POINT('Ctrl Pts',(0.732270896683394,1.49649349110809,7.94732475343653));
#53013=CARTESIAN_POINT('Ctrl Pts',(0.702085366697778,1.5109832713449,7.94951466886502));
#53014=CARTESIAN_POINT('Ctrl Pts',(0.683041686408396,1.51968694988088,7.95087184867256));
#53015=CARTESIAN_POINT('Ctrl Pts',(0.55201534789171,1.57661012590779,7.96005686810696));
#53016=CARTESIAN_POINT('Ctrl Pts',(0.435196273092605,1.6127704412075,7.96745771566366));
#53017=CARTESIAN_POINT('Ctrl Pts',(0.251121831622821,1.64826819860151,7.97891427079205));
#53018=CARTESIAN_POINT('Ctrl Pts',(0.186105438951403,1.65686865926942,7.98293138870828));
#53019=CARTESIAN_POINT('Ctrl Pts',(0.0985059633013611,1.66323488824296,
7.98849165973565));
#53020=CARTESIAN_POINT('Ctrl Pts',(0.0762258996552658,1.66440476794962,
7.9899187609824));
#53021=CARTESIAN_POINT('Ctrl Pts',(0.0380151033733838,1.66564234100321,
7.99239853011503));
#53022=CARTESIAN_POINT('Ctrl Pts',(0.0220941387001687,1.66592957827388,
7.99344134258725));
#53023=CARTESIAN_POINT('Ctrl Pts',(-0.00103821408095545,1.66601528003028,
7.99497359976737));
#53024=CARTESIAN_POINT('Ctrl Pts',(-0.00824858698606781,1.66599518222658,
7.99545361992826));
#53025=CARTESIAN_POINT('Ctrl Pts',(-0.0209388103681587,1.66587742745875,
7.99630306105777));
#53026=CARTESIAN_POINT('Ctrl Pts',(-0.0264186483120638,1.66579953500555,
7.99667138867874));
#53027=CARTESIAN_POINT('Ctrl Pts',(-0.0383280102897689,1.66557147011582,
7.99747528711151));
#53028=CARTESIAN_POINT('Ctrl Pts',(-0.0447569819896575,1.66541111065887,
7.99791138045322));
#53029=CARTESIAN_POINT('Ctrl Pts',(-0.062782991543381,1.66485703374347,
7.99913980107847));
#53030=CARTESIAN_POINT('Ctrl Pts',(-0.0743768143983663,1.66437937908024,
7.99993647093503));
#53031=CARTESIAN_POINT('Ctrl Pts',(-0.162800902106664,1.65981067961432,
8.00605809366056));
#53032=CARTESIAN_POINT('Ctrl Pts',(-0.239261837122403,1.65052316392243,
8.01161001941356));
#53033=CARTESIAN_POINT('Ctrl Pts',(-0.370962064885207,1.62518133251421,
8.02135846209847));
#53034=CARTESIAN_POINT('Ctrl Pts',(-0.426533862560759,1.61148885966271,
8.02553217262946));
#53035=CARTESIAN_POINT('Ctrl Pts',(-0.560594142451048,1.57103522777936,
8.03565143890614));
#53036=CARTESIAN_POINT('Ctrl Pts',(-0.638010556336312,1.54122146878622,
8.04153408754734));
#53037=CARTESIAN_POINT('Ctrl Pts',(-0.73354501441931,1.49599117479983,8.04880092474296));
#53038=CARTESIAN_POINT('Ctrl Pts',(-0.75399019036319,1.48579162938118,8.050357183041));
#53039=CARTESIAN_POINT('Ctrl Pts',(-0.784686729930373,1.46968107550826,
8.05269656218836));
#53040=CARTESIAN_POINT('Ctrl Pts',(-0.795094897195819,1.464076447723,8.05349027702771));
#53041=CARTESIAN_POINT('Ctrl Pts',(-0.813109955617594,1.45412685729342,
8.05486527134638));
#53042=CARTESIAN_POINT('Ctrl Pts',(-0.82074375191862,1.44983185774776,8.05544829606758));
#53043=CARTESIAN_POINT('Ctrl Pts',(-0.837880413007715,1.44001154025976,
8.05675813951172));
#53044=CARTESIAN_POINT('Ctrl Pts',(-0.847363243212797,1.43445193937729,
8.05748369358947));
#53045=CARTESIAN_POINT('Ctrl Pts',(-0.872949652750901,1.41910884543205,
8.05944390576916));
#53046=CARTESIAN_POINT('Ctrl Pts',(-0.888943715400256,1.40914517674267,
8.06067197870439));
#53047=CARTESIAN_POINT('Ctrl Pts',(-0.991004454565223,1.34313596899242,
8.06853426372312));
#53048=CARTESIAN_POINT('Ctrl Pts',(-1.071905481377,1.27950247797303,8.07486795667081));
#53049=CARTESIAN_POINT('Ctrl Pts',(-1.20644973377773,1.15190084610111,8.086203684078));
#53050=CARTESIAN_POINT('Ctrl Pts',(-1.26213527408976,1.09060048063982,8.09121461222647));
#53051=CARTESIAN_POINT('Ctrl Pts',(-1.33015657412914,1.00350049434024,8.098151631981));
#53052=CARTESIAN_POINT('Ctrl Pts',(-1.34672490227348,0.981153207537279,
8.09991743457312));
#53053=CARTESIAN_POINT('Ctrl Pts',(-1.37350914885983,0.943069472644633,
8.10292277046554));
#53054=CARTESIAN_POINT('Ctrl Pts',(-1.384033072597,0.927555817286041,8.10414598338264));
#53055=CARTESIAN_POINT('Ctrl Pts',(-1.39850197875305,0.905432142642013,
8.10589397763756));
#53056=CARTESIAN_POINT('Ctrl Pts',(-1.40266677839476,0.898966658189607,
8.10640524145278));
#53057=CARTESIAN_POINT('Ctrl Pts',(-1.40975526387062,0.887793223078588,
8.10728994421615));
#53058=CARTESIAN_POINT('Ctrl Pts',(-1.41270047985367,0.883099124857069,
8.10766197210237));
#53059=CARTESIAN_POINT('Ctrl Pts',(-1.4188711704967,0.8731543801116,8.10845102923716));
#53060=CARTESIAN_POINT('Ctrl Pts',(-1.42209090337137,0.867900587294937,
8.10886838032628));
#53061=CARTESIAN_POINT('Ctrl Pts',(-1.43081062880921,0.853493397511852,
8.11001394647914));
#53062=CARTESIAN_POINT('Ctrl Pts',(-1.43625176299642,0.844304976610573,
8.11074573993166));
#53063=CARTESIAN_POINT('Ctrl Pts',(-1.46350786890851,0.797251749940602,
8.11449677463402));
#53064=CARTESIAN_POINT('Ctrl Pts',(-1.48391348165602,0.758594551600372,
8.11758981484491));
#53065=CARTESIAN_POINT('Ctrl Pts',(-1.52523331491813,0.672254511327853,
8.12445572478906));
#53066=CARTESIAN_POINT('Ctrl Pts',(-1.54547257826816,0.62431799473414,8.12824032484045));
#53067=CARTESIAN_POINT('Ctrl Pts',(-1.56343125288101,0.575533419980911,
8.13202453882405));
#53068=CARTESIAN_POINT('Origin',(0.,0.,11.));
#53069=CARTESIAN_POINT('',(-1.56343130032506,0.575533291099565,8.8337599051164));
#53070=CARTESIAN_POINT('',(-1.56343135626508,0.575533139138958,8.63893242883258));
#53071=CARTESIAN_POINT('',(-1.56343130033213,0.575533291080363,11.));
#53072=CARTESIAN_POINT('Ctrl Pts',(-1.56343135626508,0.575533139138958,
8.63893242883258));
#53073=CARTESIAN_POINT('Ctrl Pts',(-1.55156188686748,0.607776461680207,
8.63643887173292));
#53074=CARTESIAN_POINT('Ctrl Pts',(-1.53869262498737,0.639658940293697,
8.63395501622995));
#53075=CARTESIAN_POINT('Ctrl Pts',(-1.49568115629646,0.737382554005722,
8.62630314241373));
#53076=CARTESIAN_POINT('Ctrl Pts',(-1.46223319859508,0.801668143669378,
8.62121791917477));
#53077=CARTESIAN_POINT('Ctrl Pts',(-1.41558849877557,0.878620774696276,
8.61507721229518));
#53078=CARTESIAN_POINT('Ctrl Pts',(-1.40623490021235,0.893514806920478,
8.61388576009589));
#53079=CARTESIAN_POINT('Ctrl Pts',(-1.39080123691318,0.917247454825696,
8.61198181784619));
#53080=CARTESIAN_POINT('Ctrl Pts',(-1.38486880752784,0.926179987484857,
8.61126393498847));
#53081=CARTESIAN_POINT('Ctrl Pts',(-1.37335674799568,0.943155899618945,
8.60989691550737));
#53082=CARTESIAN_POINT('Ctrl Pts',(-1.36779168125296,0.95120856384015,8.60924726887195));
#53083=CARTESIAN_POINT('Ctrl Pts',(-1.35491887154762,0.969488960392166,
8.60776948208694));
#53084=CARTESIAN_POINT('Ctrl Pts',(-1.34756564359279,0.979684052848258,
8.60694311895826));
#53085=CARTESIAN_POINT('Ctrl Pts',(-1.32761066880631,1.00670137271282,8.60474648013369));
#53086=CARTESIAN_POINT('Ctrl Pts',(-1.31480454461364,1.02337032129826,8.60338411588049));
#53087=CARTESIAN_POINT('Ctrl Pts',(-1.22647076150574,1.133952748546,8.59428534249608));
#53088=CARTESIAN_POINT('Ctrl Pts',(-1.14126030176033,1.21967542138474,8.58696449180771));
#53089=CARTESIAN_POINT('Ctrl Pts',(-0.974072506182121,1.35486719525386,
8.57382689287283));
#53090=CARTESIAN_POINT('Ctrl Pts',(-0.895696222676206,1.40790822641409,
8.56803879409931));
#53091=CARTESIAN_POINT('Ctrl Pts',(-0.802347439618496,1.46012019333494,
8.56105446659527));
#53092=CARTESIAN_POINT('Ctrl Pts',(-0.791364982907873,1.46610157687595,
8.56023133112747));
#53093=CARTESIAN_POINT('Ctrl Pts',(-0.774529699467277,1.47502631996908,
8.5589657402088));
#53094=CARTESIAN_POINT('Ctrl Pts',(-0.768724841268209,1.47805988198134,
8.55852868288533));
#53095=CARTESIAN_POINT('Ctrl Pts',(-0.758042120202873,1.48356261538287,
8.55772284364967));
#53096=CARTESIAN_POINT('Ctrl Pts',(-0.753169806554804,1.48604210216211,
8.55735470865122));
#53097=CARTESIAN_POINT('Ctrl Pts',(-0.741990403733578,1.49166212056432,
8.55650868917207));
#53098=CARTESIAN_POINT('Ctrl Pts',(-0.735675558886848,1.49478664319922,
8.55602985656871));
#53099=CARTESIAN_POINT('Ctrl Pts',(-0.715830891650597,1.50444938088344,
8.55452258772285));
#53100=CARTESIAN_POINT('Ctrl Pts',(-0.702232746780959,1.51084444437967,
8.55348612262694));
#53101=CARTESIAN_POINT('Ctrl Pts',(-0.593353960392721,1.56026162376179,
8.54516902877113));
#53102=CARTESIAN_POINT('Ctrl Pts',(-0.494309997480233,1.59440878562947,
8.53750885228049));
#53103=CARTESIAN_POINT('Ctrl Pts',(-0.282741951109502,1.64572841889288,
8.52168002866059));
#53104=CARTESIAN_POINT('Ctrl Pts',(-0.170303755067803,1.66113532481739,
8.51357088298754));
#53105=CARTESIAN_POINT('Ctrl Pts',(-0.037798613936452,1.66568374548627,
8.50449900090682));
#53106=CARTESIAN_POINT('Ctrl Pts',(-0.0184323687750814,1.66601061758158,
8.50318424426596));
#53107=CARTESIAN_POINT('Ctrl Pts',(0.0120391746531707,1.66599349966595,
8.50113225953731));
#53108=CARTESIAN_POINT('Ctrl Pts',(0.0231423312824171,1.66587626356018,
8.50038804384748));
#53109=CARTESIAN_POINT('Ctrl Pts',(0.0439585446219458,1.66544830721385,
8.49899904255763));
#53110=CARTESIAN_POINT('Ctrl Pts',(0.053671604258126,1.66516359057669,8.49835347481421));
#53111=CARTESIAN_POINT('Ctrl Pts',(0.0754987265250821,1.66433259149579,
8.4969082330555));
#53112=CARTESIAN_POINT('Ctrl Pts',(0.0876105185073098,1.66373899480864,
8.49611006793661));
#53113=CARTESIAN_POINT('Ctrl Pts',(0.123281745811791,1.66160013190565,8.49376970856189));
#53114=CARTESIAN_POINT('Ctrl Pts',(0.14681665651005,1.65968621924105,8.49223899015564));
#53115=CARTESIAN_POINT('Ctrl Pts',(0.270937909627736,1.64693132568469,8.48422332523232));
#53116=CARTESIAN_POINT('Ctrl Pts',(0.370425168801974,1.62744541907731,8.47801431130899));
#53117=CARTESIAN_POINT('Ctrl Pts',(0.54480232960941,1.57646006844147,8.46691723177511));
#53118=CARTESIAN_POINT('Ctrl Pts',(0.620321168007714,1.54830093285588,8.46202790150696));
#53119=CARTESIAN_POINT('Ctrl Pts',(0.71620349224181,1.50440415780349,8.45538074387492));
#53120=CARTESIAN_POINT('Ctrl Pts',(0.738666157512167,1.49350309257644,8.45378980383227));
#53121=CARTESIAN_POINT('Ctrl Pts',(0.776278412946118,1.47419390006593,8.45105418433659));
#53122=CARTESIAN_POINT('Ctrl Pts',(0.791557687843593,1.46604645171927,8.4499222827935));
#53123=CARTESIAN_POINT('Ctrl Pts',(0.813228435922316,1.45405332608714,8.44828315737086));
#53124=CARTESIAN_POINT('Ctrl Pts',(0.819725959529565,1.4504002585851,8.44778729027167));
#53125=CARTESIAN_POINT('Ctrl Pts',(0.830981437879596,1.44397236338543,8.44692022653032));
#53126=CARTESIAN_POINT('Ctrl Pts',(0.835750498100171,1.44121734664197,8.44655028431256));
#53127=CARTESIAN_POINT('Ctrl Pts',(0.845929426493821,1.43526961315458,8.44575507504796));
#53128=CARTESIAN_POINT('Ctrl Pts',(0.851334836389783,1.43206998786148,8.44532939510462));
#53129=CARTESIAN_POINT('Ctrl Pts',(0.866103180307964,1.42321499754878,8.44415731940145));
#53130=CARTESIAN_POINT('Ctrl Pts',(0.875428517629792,1.41749798688334,8.44340716944171));
#53131=CARTESIAN_POINT('Ctrl Pts',(0.927476389524408,1.38487993222596,8.43916644187511));
#53132=CARTESIAN_POINT('Ctrl Pts',(0.969011275985883,1.35614195090091,8.43557725806078));
#53133=CARTESIAN_POINT('Ctrl Pts',(1.08575340343721,1.26726445246093,8.42500978774405));
#53134=CARTESIAN_POINT('Ctrl Pts',(1.15713811807773,1.20243586642979,8.41793932531378));
#53135=CARTESIAN_POINT('Ctrl Pts',(1.26599318918323,1.08485515245093,8.40641179137648));
#53136=CARTESIAN_POINT('Ctrl Pts',(1.30672176021917,1.03543679839453,8.40187931671649));
#53137=CARTESIAN_POINT('Ctrl Pts',(1.36082250757125,0.961499435942552,8.39554419973778));
#53138=CARTESIAN_POINT('Ctrl Pts',(1.37657836831889,0.938803076366341,8.39365460294419));
#53139=CARTESIAN_POINT('Ctrl Pts',(1.39875615255915,0.905096171127229,8.39092580189108));
#53140=CARTESIAN_POINT('Ctrl Pts',(1.40562713718082,0.894388182009055,8.39006996346471));
#53141=CARTESIAN_POINT('Ctrl Pts',(1.41756205944802,0.875311063455623,8.38856425959711));
#53142=CARTESIAN_POINT('Ctrl Pts',(1.42267614401365,0.866974190192241,8.38791256703512));
#53143=CARTESIAN_POINT('Ctrl Pts',(1.43325814280668,0.849377840899167,8.38655000421158));
#53144=CARTESIAN_POINT('Ctrl Pts',(1.43871043773465,0.840109460742561,8.38583972456393));
#53145=CARTESIAN_POINT('Ctrl Pts',(1.45291230253581,0.815423852669319,8.38396698645757));
#53146=CARTESIAN_POINT('Ctrl Pts',(1.4615063546662,0.799918391391817,8.38281012114899));
#53147=CARTESIAN_POINT('Ctrl Pts',(1.50146908179505,0.725022422332459,8.37730958972848));
#53148=CARTESIAN_POINT('Ctrl Pts',(1.5294766270699,0.663904911482516,8.37308427077122));
#53149=CARTESIAN_POINT('Ctrl Pts',(1.6057657928442,0.466764629046022,8.36000058633287));
#53150=CARTESIAN_POINT('Ctrl Pts',(1.64012150314167,0.326104098013765,8.35148227773574));
#53151=CARTESIAN_POINT('Ctrl Pts',(1.65832675345838,0.161186801075403,8.3408224937926));
#53152=CARTESIAN_POINT('Ctrl Pts',(1.66028910526352,0.139530584330247,8.33940861422835));
#53153=CARTESIAN_POINT('Ctrl Pts',(1.66240306244523,0.109719583436152,8.33743537121793));
#53154=CARTESIAN_POINT('Ctrl Pts',(1.66291954880702,0.101591812845439,8.33689463102627));
#53155=CARTESIAN_POINT('Ctrl Pts',(1.66369165108474,0.0878502565845365,
8.33597526722552));
#53156=CARTESIAN_POINT('Ctrl Pts',(1.66397850041224,0.0822382307008209,
8.33559835105518));
#53157=CARTESIAN_POINT('Ctrl Pts',(1.66451203273601,0.0706502957458508,
8.33481690544078));
#53158=CARTESIAN_POINT('Ctrl Pts',(1.66475493467458,0.0646743847377087,
8.33441219077767));
#53159=CARTESIAN_POINT('Ctrl Pts',(1.66531277369112,0.0488511530677596,
8.3333362426067));
#53160=CARTESIAN_POINT('Ctrl Pts',(1.66557253759491,0.0390023021518545,
8.33266210279372));
#53161=CARTESIAN_POINT('Ctrl Pts',(1.66633511834445,-0.00457150655297279,
8.32966159127403));
#53162=CARTESIAN_POINT('Ctrl Pts',(1.66590100919347,-0.0383025707807233,
8.32729142754564));
#53163=CARTESIAN_POINT('Ctrl Pts',(1.66351732034801,-0.093411286807257,
8.32336500713657));
#53164=CARTESIAN_POINT('Ctrl Pts',(1.66217769252649,-0.114807673716851,
8.32182713011855));
#53165=CARTESIAN_POINT('Ctrl Pts',(1.65209296933613,-0.237777097563427,
8.31293036702973));
#53166=CARTESIAN_POINT('Ctrl Pts',(1.63445069092764,-0.338410797238987,
8.3054376232841));
#53167=CARTESIAN_POINT('Ctrl Pts',(1.58869943149386,-0.506806506664729,
8.29293066540681));
#53168=CARTESIAN_POINT('Ctrl Pts',(1.56512511102975,-0.575503874427037,
8.28783360743431));
#53169=CARTESIAN_POINT('Ctrl Pts',(1.53035770083746,-0.658688784506944,
8.28168103794203));
#53170=CARTESIAN_POINT('Ctrl Pts',(1.52331535685741,-0.674815509710883,
8.28048890992875));
#53171=CARTESIAN_POINT('Ctrl Pts',(1.51157147464176,-0.700587393571792,
8.27858415480886));
#53172=CARTESIAN_POINT('Ctrl Pts',(1.50703012543485,-0.710303617699735,
8.2778661266026));
#53173=CARTESIAN_POINT('Ctrl Pts',(1.49816538750638,-0.728801940612003,
8.27649899761351));
#53174=CARTESIAN_POINT('Ctrl Pts',(1.49385782508153,-0.737591080735014,
8.27584938523861));
#53175=CARTESIAN_POINT('Ctrl Pts',(1.48384391006696,-0.757575829778588,
8.27437190451116));
#53176=CARTESIAN_POINT('Ctrl Pts',(1.47808780626389,-0.768745951967338,
8.27354581053486));
#53177=CARTESIAN_POINT('Ctrl Pts',(1.46237439906771,-0.798409815685436,
8.27135039724));
#53178=CARTESIAN_POINT('Ctrl Pts',(1.45219263678725,-0.816782544906711,
8.2699889750509));
#53179=CARTESIAN_POINT('Ctrl Pts',(1.38113324543105,-0.939475939905433,
8.26087372301941));
#53180=CARTESIAN_POINT('Ctrl Pts',(1.30941412785534,-1.03710297131947,8.25353761411919));
#53181=CARTESIAN_POINT('Ctrl Pts',(1.18295665543291,-1.17497374578399,8.24210602070799));
#53182=CARTESIAN_POINT('Ctrl Pts',(1.13527908506359,-1.22110191340699,8.23804468836693));
#53183=CARTESIAN_POINT('Ctrl Pts',(1.06794430597665,-1.27888826954697,8.23242878418181));
#53184=CARTESIAN_POINT('Ctrl Pts',(1.05061063753319,-1.29316566391574,8.2309926659195));
#53185=CARTESIAN_POINT('Ctrl Pts',(1.02044054254375,-1.31700916483767,8.22849874165069));
#53186=CARTESIAN_POINT('Ctrl Pts',(1.007744747727,-1.32674885281173,8.22745094208523));
#53187=CARTESIAN_POINT('Ctrl Pts',(0.989116611891225,-1.34061796131578,
8.22591269799433));
#53188=CARTESIAN_POINT('Ctrl Pts',(0.983294133596994,-1.34489435724001,
8.22543178173831));
#53189=CARTESIAN_POINT('Ctrl Pts',(0.973044789403469,-1.35231998854345,
8.22458465863413));
#53190=CARTESIAN_POINT('Ctrl Pts',(0.968630053211665,-1.35548564448661,
8.22421958123445));
#53191=CARTESIAN_POINT('Ctrl Pts',(0.958980170915469,-1.36233402591073,
8.22342106703799));
#53192=CARTESIAN_POINT('Ctrl Pts',(0.953739345277282,-1.36600813474385,
8.2229871000141));
#53193=CARTESIAN_POINT('Ctrl Pts',(0.939049880231659,-1.37618052135733,
8.22177020817909));
#53194=CARTESIAN_POINT('Ctrl Pts',(0.929555336050126,-1.38261142913146,
8.22098306402333));
#53195=CARTESIAN_POINT('Ctrl Pts',(0.865300432886657,-1.42517199251911,
8.21565597055711));
#53196=CARTESIAN_POINT('Ctrl Pts',(0.808518968618958,-1.45813415207656,
8.21095032686179));
#53197=CARTESIAN_POINT('Ctrl Pts',(0.731110498994364,-1.49715682063077,
8.2046666923073));
#53198=CARTESIAN_POINT('Ctrl Pts',(0.712092849761228,-1.50629507818682,
8.20313269654204));
#53199=CARTESIAN_POINT('Ctrl Pts',(0.630755548887342,-1.54349415124639,
8.19662382333867));
#53200=CARTESIAN_POINT('Ctrl Pts',(0.566910725692281,-1.56806884334495,
8.19164570591671));
#53201=CARTESIAN_POINT('Ctrl Pts',(0.433540686573515,-1.61019026881979,
8.18162694175109));
#53202=CARTESIAN_POINT('Ctrl Pts',(0.36402374556907,-1.62731663855451,8.17660487566422));
#53203=CARTESIAN_POINT('Ctrl Pts',(0.276353459710387,-1.64301313830792,
8.17052754982417));
#53204=CARTESIAN_POINT('Ctrl Pts',(0.259046607574322,-1.64583058157559,
8.16933975336315));
#53205=CARTESIAN_POINT('Ctrl Pts',(0.231099985752947,-1.64992834008624,
8.16744020801134));
#53206=CARTESIAN_POINT('Ctrl Pts',(0.220487110611126,-1.65138008167619,
8.16672311109309));
#53207=CARTESIAN_POINT('Ctrl Pts',(0.200147406788656,-1.65396278250553,
8.1653566802735));
#53208=CARTESIAN_POINT('Ctrl Pts',(0.190423202524032,-1.6551105344601,8.16470684492952));
#53209=CARTESIAN_POINT('Ctrl Pts',(0.168171140269557,-1.65753824578816,
8.16322738727057));
#53210=CARTESIAN_POINT('Ctrl Pts',(0.155637657767756,-1.65876203918161,
8.16239955639886));
#53211=CARTESIAN_POINT('Ctrl Pts',(0.115531171631399,-1.66221952493399,
8.15976700409098));
#53212=CARTESIAN_POINT('Ctrl Pts',(0.0879150538168917,-1.66390873719184,
8.15797921838882));
#53213=CARTESIAN_POINT('Ctrl Pts',(-0.0712410793702744,-1.66967005678191,
8.14779416195986));
#53214=CARTESIAN_POINT('Ctrl Pts',(-0.202849170166269,-1.65883336407098,
8.13988171730874));
#53215=CARTESIAN_POINT('Ctrl Pts',(-0.401934414469848,-1.61837084025625,
8.12741818286835));
#53216=CARTESIAN_POINT('Ctrl Pts',(-0.471052639345271,-1.59961948996927,
8.12298330791998));
#53217=CARTESIAN_POINT('Ctrl Pts',(-0.5536843387361,-1.57138122825364,8.11731785579805));
#53218=CARTESIAN_POINT('Ctrl Pts',(-0.568551570314844,-1.56606333809926,
8.11628362046686));
#53219=CARTESIAN_POINT('Ctrl Pts',(-0.590071468988671,-1.55801903105587,
8.11476170574093));
#53220=CARTESIAN_POINT('Ctrl Pts',(-0.596786128560097,-1.5554594021245,
8.11428327419583));
#53221=CARTESIAN_POINT('Ctrl Pts',(-0.608543988677916,-1.55088996574776,
8.11343888331453));
#53222=CARTESIAN_POINT('Ctrl Pts',(-0.61359424009795,-1.5488988279637,8.1130740283054));
#53223=CARTESIAN_POINT('Ctrl Pts',(-0.624601301424744,-1.54449684596546,
8.1122739827093));
#53224=CARTESIAN_POINT('Ctrl Pts',(-0.630553830633365,-1.5420762484801,
8.11183824344927));
#53225=CARTESIAN_POINT('Ctrl Pts',(-0.647195288523337,-1.53519653333726,
8.11061169382127));
#53226=CARTESIAN_POINT('Ctrl Pts',(-0.657851695603722,-1.53066040170428,
8.10981656075523));
#53227=CARTESIAN_POINT('Ctrl Pts',(-0.734151124163853,-1.49723797377155,
8.10405771924946));
#53228=CARTESIAN_POINT('Ctrl Pts',(-0.797908925452065,-1.46425354522437,
8.09889652745042));
#53229=CARTESIAN_POINT('Ctrl Pts',(-0.87114283990524,-1.42016058667957,
8.09268971650659));
#53230=CARTESIAN_POINT('Ctrl Pts',(-0.882861081963212,-1.41290560375266,
8.0916874773964));
#53231=CARTESIAN_POINT('Ctrl Pts',(-0.950653911779776,-1.36976109884206,
8.08584005816142));
#53232=CARTESIAN_POINT('Ctrl Pts',(-1.00462946544215,-1.33067980954118,
8.08098920105092));
#53233=CARTESIAN_POINT('Ctrl Pts',(-1.09414974125374,-1.25730262110943,
8.07268652091806));
#53234=CARTESIAN_POINT('Ctrl Pts',(-1.13078045578505,-1.22446308427605,
8.06920371910412));
#53235=CARTESIAN_POINT('Ctrl Pts',(-1.18977844442658,-1.1666619049471,8.06345679052604));
#53236=CARTESIAN_POINT('Ctrl Pts',(-1.21294155673913,-1.14256107243737,
8.06116080325297));
#53237=CARTESIAN_POINT('Ctrl Pts',(-1.2445464679894,-1.10763140820518,8.05796837551124));
#53238=CARTESIAN_POINT('Ctrl Pts',(-1.25360230672679,-1.09737164324671,
8.05704627643156));
#53239=CARTESIAN_POINT('Ctrl Pts',(-1.26900871066669,-1.0794774018588,8.05546424558195));
#53240=CARTESIAN_POINT('Ctrl Pts',(-1.2754192050423,-1.07189571676968,8.0548018592463));
#53241=CARTESIAN_POINT('Ctrl Pts',(-1.28760122431716,-1.05722403055176,
8.05353489849969));
#53242=CARTESIAN_POINT('Ctrl Pts',(-1.29338289778619,-1.05014296598103,
8.05292992646612));
#53243=CARTESIAN_POINT('Ctrl Pts',(-1.30691522231043,-1.03328804746564,
8.05150495096485));
#53244=CARTESIAN_POINT('Ctrl Pts',(-1.31461503802747,-1.02347393864395,
8.05068698698352));
#53245=CARTESIAN_POINT('Ctrl Pts',(-1.33753643360303,-0.993573052116878,
8.048229097795));
#53246=CARTESIAN_POINT('Ctrl Pts',(-1.35241357714633,-0.973225946984257,
8.04660244422627));
#53247=CARTESIAN_POINT('Ctrl Pts',(-1.44187733165743,-0.844853229815511,
8.03659917607584));
#53248=CARTESIAN_POINT('Ctrl Pts',(-1.50393918730732,-0.728667702234672,
8.02870669459865));
#53249=CARTESIAN_POINT('Ctrl Pts',(-1.5777268343713,-0.539850463990858,
8.01626920027877));
#53250=CARTESIAN_POINT('Ctrl Pts',(-1.59942140196838,-0.471708941985083,
8.01184045526884));
#53251=CARTESIAN_POINT('Ctrl Pts',(-1.62048516886904,-0.387082422159707,
8.00618235550722));
#53252=CARTESIAN_POINT('Ctrl Pts',(-1.62407847852099,-0.371717682298452,
8.00514878485045));
#53253=CARTESIAN_POINT('Ctrl Pts',(-1.62898933120278,-0.349286947217741,
8.00362767055483));
#53254=CARTESIAN_POINT('Ctrl Pts',(-1.63048035819566,-0.34225927228254,
8.00314936111851));
#53255=CARTESIAN_POINT('Ctrl Pts',(-1.63301816922033,-0.329904727329983,
8.00230510358389));
#53256=CARTESIAN_POINT('Ctrl Pts',(-1.63408444039237,-0.3245820551392,8.00194025857179));
#53257=CARTESIAN_POINT('Ctrl Pts',(-1.63635635258896,-0.312945996847856,
8.00114013371571));
#53258=CARTESIAN_POINT('Ctrl Pts',(-1.63755146141554,-0.306630913851365,
8.00070430426921));
#53259=CARTESIAN_POINT('Ctrl Pts',(-1.64079871836077,-0.288911469363451,
7.99947726563726));
#53260=CARTESIAN_POINT('Ctrl Pts',(-1.64276842137086,-0.277492641922035,
7.9986817285183));
#53261=CARTESIAN_POINT('Ctrl Pts',(-1.65618234371281,-0.194574367272832,
7.99287458640212));
#53262=CARTESIAN_POINT('Ctrl Pts',(-1.66307219549193,-0.122424018168786,
7.98766171063302));
#53263=CARTESIAN_POINT('Ctrl Pts',(-1.66573474981424,-0.0338603643184752,
7.98122730133518));
#53264=CARTESIAN_POINT('Ctrl Pts',(-1.66598535914898,-0.017651009351957,
7.98004801819825));
#53265=CARTESIAN_POINT('Ctrl Pts',(-1.6661107565004,0.127358288344095,7.96949372028456));
#53266=CARTESIAN_POINT('Ctrl Pts',(-1.65128543468728,0.255761016431306,
7.96016710179683));
#53267=CARTESIAN_POINT('Ctrl Pts',(-1.61713992253171,0.401036344385619,
7.94991017892582));
#53268=CARTESIAN_POINT('Ctrl Pts',(-1.61211089489218,0.420797106648802,
7.94852026987872));
#53269=CARTESIAN_POINT('Ctrl Pts',(-1.60340887862091,0.45254042544968,7.94629526479896));
#53270=CARTESIAN_POINT('Ctrl Pts',(-1.59996137674876,0.464582044946932,
7.94545302892488));
#53271=CARTESIAN_POINT('Ctrl Pts',(-1.59358748337374,0.485932209161064,
7.94396259707877));
#53272=CARTESIAN_POINT('Ctrl Pts',(-1.59071453219384,0.495255957145969,
7.94331270011679));
#53273=CARTESIAN_POINT('Ctrl Pts',(-1.58447198456338,0.514900364063271,
7.94194525931866));
#53274=CARTESIAN_POINT('Ctrl Pts',(-1.58108306386391,0.525214441293306,
7.94122838224518));
#53275=CARTESIAN_POINT('Ctrl Pts',(-1.57304313111398,0.54890046792219,7.93958415920245));
#53276=CARTESIAN_POINT('Ctrl Pts',(-1.56832202215773,0.562247686748594,
7.93865916364133));
#53277=CARTESIAN_POINT('Ctrl Pts',(-1.56343130037338,0.575533290968306,
7.93773948050229));
#53278=CARTESIAN_POINT('Ctrl Pts',(-1.56343125288101,0.575533419980911,
8.13202453882405));
#53279=CARTESIAN_POINT('Ctrl Pts',(-1.57647476592086,0.540100836527222,
8.13477304034238));
#53280=CARTESIAN_POINT('Ctrl Pts',(-1.58831519947266,0.504220896311646,
8.13752158935909));
#53281=CARTESIAN_POINT('Ctrl Pts',(-1.62278062997201,0.386457854613517,
8.14639622254069));
#53282=CARTESIAN_POINT('Ctrl Pts',(-1.64036942313108,0.303246857124685,
8.1524335310521));
#53283=CARTESIAN_POINT('Ctrl Pts',(-1.65457539086693,0.196138385182223,
8.15986415733841));
#53284=CARTESIAN_POINT('Ctrl Pts',(-1.65713685274032,0.17316909209299,8.16143874830773));
#53285=CARTESIAN_POINT('Ctrl Pts',(-1.66028981546747,0.138328221684353,
8.16379976903536));
#53286=CARTESIAN_POINT('Ctrl Pts',(-1.66123349042863,0.126492178388229,
8.16459709293344));
#53287=CARTESIAN_POINT('Ctrl Pts',(-1.66265368033757,0.105903485861357,
8.16597606859828));
#53288=CARTESIAN_POINT('Ctrl Pts',(-1.66318779402146,0.0971554214281328,
8.16655949774668));
#53289=CARTESIAN_POINT('Ctrl Pts',(-1.6642341778765,0.0774636514998475,
8.16786737254177));
#53290=CARTESIAN_POINT('Ctrl Pts',(-1.66470758768369,0.0665182176389728,
8.16859057878443));
#53291=CARTESIAN_POINT('Ctrl Pts',(-1.66569572471977,0.0369094502227332,
8.17053730486913));
#53292=CARTESIAN_POINT('Ctrl Pts',(-1.66600476746025,0.0182404851654997,
8.17175439696182));
#53293=CARTESIAN_POINT('Ctrl Pts',(-1.66597468525883,-0.0982129333982162,
8.17928915711391));
#53294=CARTESIAN_POINT('Ctrl Pts',(-1.6573412001664,-0.195809012424007,
8.18533701810807));
#53295=CARTESIAN_POINT('Ctrl Pts',(-1.622980312546,-0.388754856964475,8.19732910409969));
#53296=CARTESIAN_POINT('Ctrl Pts',(-1.59725732387335,-0.483695423463917,
8.20325270540061));
#53297=CARTESIAN_POINT('Ctrl Pts',(-1.55225470669452,-0.605877913944535,
8.21150088433053));
#53298=CARTESIAN_POINT('Ctrl Pts',(-1.54031573519923,-0.635617685131605,
8.21356123459514));
#53299=CARTESIAN_POINT('Ctrl Pts',(-1.52366349205209,-0.673868895149786,
8.21630363282603));
#53300=CARTESIAN_POINT('Ctrl Pts',(-1.51972202289346,-0.682711276391223,
8.21694414380728));
#53301=CARTESIAN_POINT('Ctrl Pts',(-1.51323680997241,-0.696925880171094,
8.21798522492591));
#53302=CARTESIAN_POINT('Ctrl Pts',(-1.51074091781395,-0.702319871544494,
8.21838296128972));
#53303=CARTESIAN_POINT('Ctrl Pts',(-1.50581976664892,-0.712807588427169,
8.21916175031152));
#53304=CARTESIAN_POINT('Ctrl Pts',(-1.50339741501869,-0.717902525844541,
8.21954263007709));
#53305=CARTESIAN_POINT('Ctrl Pts',(-1.49736493318513,-0.730426230018712,
8.22048497655383));
#53306=CARTESIAN_POINT('Ctrl Pts',(-1.49372537370854,-0.737840579962083,
8.22104820089348));
#53307=CARTESIAN_POINT('Ctrl Pts',(-1.47993756403112,-0.765408358409469,
8.2231614910417));
#53308=CARTESIAN_POINT('Ctrl Pts',(-1.46943583693606,-0.785381019987932,
8.22473093530008));
#53309=CARTESIAN_POINT('Ctrl Pts',(-1.44109507755261,-0.836721501734517,
8.22885457112118));
#53310=CARTESIAN_POINT('Ctrl Pts',(-1.42263717149119,-0.867733281178739,
8.23143414725975));
#53311=CARTESIAN_POINT('Ctrl Pts',(-1.36414810505131,-0.95911442993948,
8.23925817852516));
#53312=CARTESIAN_POINT('Ctrl Pts',(-1.32117271813111,-1.01749846749838,
8.24455824763871));
#53313=CARTESIAN_POINT('Ctrl Pts',(-1.21044257897313,-1.1490385437035,8.25702146033253));
#53314=CARTESIAN_POINT('Ctrl Pts',(-1.13964737971101,-1.21929116152939,
8.2641054818042));
#53315=CARTESIAN_POINT('Ctrl Pts',(-1.04847294431203,-1.29484206897693,
8.27220144075366));
#53316=CARTESIAN_POINT('Ctrl Pts',(-1.03375127060128,-1.30662537085953,
8.27348071092021));
#53317=CARTESIAN_POINT('Ctrl Pts',(-1.01013308025676,-1.32488038834047,
8.27549018031205));
#53318=CARTESIAN_POINT('Ctrl Pts',(-1.00136744372863,-1.33151798182014,
8.27622689103781));
#53319=CARTESIAN_POINT('Ctrl Pts',(-0.985502100851652,-1.34328638778345,
8.27754436172706));
#53320=CARTESIAN_POINT('Ctrl Pts',(-0.978426496230581,-1.34844885215257,
8.27812633899214));
#53321=CARTESIAN_POINT('Ctrl Pts',(-0.961709746217389,-1.36044478039167,
8.27948847004329));
#53322=CARTESIAN_POINT('Ctrl Pts',(-0.952035872788811,-1.36723200131673,
8.28026683063976));
#53323=CARTESIAN_POINT('Ctrl Pts',(-0.923466736818148,-1.38682593928159,
8.2825374573401));
#53324=CARTESIAN_POINT('Ctrl Pts',(-0.904379063350026,-1.39934827375732,
8.28401904348867));
#53325=CARTESIAN_POINT('Ctrl Pts',(-0.814985446772792,-1.45540089210671,
8.29080667277284));
#53326=CARTESIAN_POINT('Ctrl Pts',(-0.741754629720165,-1.49405335264897,
8.29593631653938));
#53327=CARTESIAN_POINT('Ctrl Pts',(-0.613422720170676,-1.55001684498241,
8.30451966143371));
#53328=CARTESIAN_POINT('Ctrl Pts',(-0.559750394507417,-1.57019714476803,
8.30800055651609));
#53329=CARTESIAN_POINT('Ctrl Pts',(-0.431754905911915,-1.61092370584721,
8.31624369254192));
#53330=CARTESIAN_POINT('Ctrl Pts',(-0.356842673349537,-1.6291555074469,
8.32102412673696));
#53331=CARTESIAN_POINT('Ctrl Pts',(-0.269511455405308,-1.64409678387728,
8.3268193473141));
#53332=CARTESIAN_POINT('Ctrl Pts',(-0.258053626905415,-1.64593407112163,
8.327584058195));
#53333=CARTESIAN_POINT('Ctrl Pts',(-0.240217596007902,-1.64860330781699,
8.32878257245176));
#53334=CARTESIAN_POINT('Ctrl Pts',(-0.233851928842736,-1.64951830298534,
8.32921192251728));
#53335=CARTESIAN_POINT('Ctrl Pts',(-0.222051936946935,-1.65114474678727,
8.330011036413));
#53336=CARTESIAN_POINT('Ctrl Pts',(-0.216619207043025,-1.65186626380461,
8.33038023817655));
#53337=CARTESIAN_POINT('Ctrl Pts',(-0.204030903755151,-1.65347494052239,
8.33123865906529));
#53338=CARTESIAN_POINT('Ctrl Pts',(-0.196873060447458,-1.65434246208436,
8.33172893639085));
#53339=CARTESIAN_POINT('Ctrl Pts',(-0.173891085071332,-1.65697658865389,
8.33330956472752));
#53340=CARTESIAN_POINT('Ctrl Pts',(-0.158047721611828,-1.65856275015164,
8.33440905302607));
#53341=CARTESIAN_POINT('Ctrl Pts',(-0.119958442970756,-1.66182538422732,
8.33707213914044));
#53342=CARTESIAN_POINT('Ctrl Pts',(-0.0976971786070598,-1.6632825366167,
8.33864472367392));
#53343=CARTESIAN_POINT('Ctrl Pts',(-0.00996217509476534,-1.66725809757432,
8.34488988679133));
#53344=CARTESIAN_POINT('Ctrl Pts',(0.0556047338421275,-1.66636011197354,
8.34965838622301));
#53345=CARTESIAN_POINT('Ctrl Pts',(0.242542409377467,-1.6527533267283,8.36330235997769));
#53346=CARTESIAN_POINT('Ctrl Pts',(0.36282327793294,-1.63057965136885,8.37210888261677));
#53347=CARTESIAN_POINT('Ctrl Pts',(0.49967003365011,-1.58944144503542,8.38193785222053));
#53348=CARTESIAN_POINT('Ctrl Pts',(0.519603540309516,-1.58303710621968,
8.38336583231438));
#53349=CARTESIAN_POINT('Ctrl Pts',(0.551282382118694,-1.57219628107933,
8.38563006041636));
#53350=CARTESIAN_POINT('Ctrl Pts',(0.563106917524571,-1.56800000811813,
8.38647405646144));
#53351=CARTESIAN_POINT('Ctrl Pts',(0.584067590274744,-1.56029381994299,
8.38796843509581));
#53352=CARTESIAN_POINT('Ctrl Pts',(0.593222209193225,-1.55683627016599,
8.38862051758036));
#53353=CARTESIAN_POINT('Ctrl Pts',(0.612354929654905,-1.5494168849323,8.38998233798931));
#53354=CARTESIAN_POINT('Ctrl Pts',(0.622326298831967,-1.54543884708144,
8.39069149885451));
#53355=CARTESIAN_POINT('Ctrl Pts',(0.648581508597556,-1.53466911416794,
8.39255770951409));
#53356=CARTESIAN_POINT('Ctrl Pts',(0.664797393625992,-1.52771454382787,
8.3937092380412));
#53357=CARTESIAN_POINT('Ctrl Pts',(0.747824927532054,-1.49053378705425,
8.39960461243109));
#53358=CARTESIAN_POINT('Ctrl Pts',(0.812702572530906,-1.45617635501,8.40420438695232));
#53359=CARTESIAN_POINT('Ctrl Pts',(0.958675282472613,-1.36606788449267,
8.41479245417914));
#53360=CARTESIAN_POINT('Ctrl Pts',(1.0375110088575,-1.30719912777315,8.42069732865638));
#53361=CARTESIAN_POINT('Ctrl Pts',(1.13329006273765,-1.22152697997433,8.42866961566388));
#53362=CARTESIAN_POINT('Ctrl Pts',(1.15532255246585,-1.20070985214336,8.4305671629239));
#53363=CARTESIAN_POINT('Ctrl Pts',(1.19714827946132,-1.15897387662775,8.43432480645616));
#53364=CARTESIAN_POINT('Ctrl Pts',(1.21699092596074,-1.13812007301849,8.43618135541146));
#53365=CARTESIAN_POINT('Ctrl Pts',(1.24252938369635,-1.10984845335819,8.43868820408379));
#53366=CARTESIAN_POINT('Ctrl Pts',(1.24871837709632,-1.1028804393618,8.4393052807529));
#53367=CARTESIAN_POINT('Ctrl Pts',(1.25870585023804,-1.0914439853123,8.44031753452339));
#53368=CARTESIAN_POINT('Ctrl Pts',(1.26253987070088,-1.08700665255807,8.44071015743864));
#53369=CARTESIAN_POINT('Ctrl Pts',(1.27005126576689,-1.07821993232242,8.44148758170891));
#53370=CARTESIAN_POINT('Ctrl Pts',(1.27372989938261,-1.0738717708539,8.44187228507094));
#53371=CARTESIAN_POINT('Ctrl Pts',(1.28286281182262,-1.06296368177307,8.44283717214751));
#53372=CARTESIAN_POINT('Ctrl Pts',(1.28828907797353,-1.05638062575749,8.4434192982104));
#53373=CARTESIAN_POINT('Ctrl Pts',(1.30917141330941,-1.03064633665681,8.44569325331029));
#53374=CARTESIAN_POINT('Ctrl Pts',(1.3242521066046,-1.011196253096,8.44740832258734));
#53375=CARTESIAN_POINT('Ctrl Pts',(1.36326334225511,-0.958512290178814,
8.45202933435846));
#53376=CARTESIAN_POINT('Ctrl Pts',(1.38640814417708,-0.924718757234221,
8.45496807318686));
#53377=CARTESIAN_POINT('Ctrl Pts',(1.47397007662694,-0.786182986782976,
8.46682376122934));
#53378=CARTESIAN_POINT('Ctrl Pts',(1.52796041133313,-0.675288889839493,
8.47585606659958));
#53379=CARTESIAN_POINT('Ctrl Pts',(1.58509984556531,-0.515015217807913,
8.48785241306181));
#53380=CARTESIAN_POINT('Ctrl Pts',(1.59905027440103,-0.469916133318926,
8.49112542052958));
#53381=CARTESIAN_POINT('Ctrl Pts',(1.61513126941199,-0.408853887837366,
8.49542294259421));
#53382=CARTESIAN_POINT('Ctrl Pts',(1.61897250401778,-0.393368251163257,
8.49650159860911));
#53383=CARTESIAN_POINT('Ctrl Pts',(1.62494376012842,-0.367724649216032,
8.49826992902559));
#53384=CARTESIAN_POINT('Ctrl Pts',(1.62720229830606,-0.357598000581008,
8.49896367889286));
#53385=CARTESIAN_POINT('Ctrl Pts',(1.6314367977714,-0.337740363894764,8.50031540979819));
#53386=CARTESIAN_POINT('Ctrl Pts',(1.63342065183233,-0.328011524121865,
8.500973617056));
#53387=CARTESIAN_POINT('Ctrl Pts',(1.6379316408381,-0.304833069161371,8.50253247658616));
#53388=CARTESIAN_POINT('Ctrl Pts',(1.64038029659371,-0.291368771715381,
8.50343060775144));
#53389=CARTESIAN_POINT('Ctrl Pts',(1.64823671670308,-0.244925491507286,
8.50650460064613));
#53390=CARTESIAN_POINT('Ctrl Pts',(1.65281820004663,-0.211813622389608,
8.50865454970477));
#53391=CARTESIAN_POINT('Ctrl Pts',(1.66167140356726,-0.1296986704086,8.51390372066582));
#53392=CARTESIAN_POINT('Ctrl Pts',(1.66477553413735,-0.0806012339867121,
8.51696970605745));
#53393=CARTESIAN_POINT('Ctrl Pts',(1.66695948734626,0.035122304287747,8.52411129432649));
#53394=CARTESIAN_POINT('Ctrl Pts',(1.66422524699041,0.101695572042797,8.528152580872));
#53395=CARTESIAN_POINT('Ctrl Pts',(1.65608437628265,0.182049508679997,8.53309681936171));
#53396=CARTESIAN_POINT('Ctrl Pts',(1.65447319944977,0.196152772534445,8.53396722491075));
#53397=CARTESIAN_POINT('Ctrl Pts',(1.64368205888767,0.280983762683923,8.53922673288243));
#53398=CARTESIAN_POINT('Ctrl Pts',(1.63014931032971,0.35107440394229,8.543671425714));
#53399=CARTESIAN_POINT('Ctrl Pts',(1.60925145291554,0.431276959934603,8.54909285122589));
#53400=CARTESIAN_POINT('Ctrl Pts',(1.60621545229925,0.442449948900418,8.54985587867052));
#53401=CARTESIAN_POINT('Ctrl Pts',(1.60131396227464,0.459772639037495,8.55105230811356));
#53402=CARTESIAN_POINT('Ctrl Pts',(1.59952885613828,0.465944975617436,8.55148128132113));
#53403=CARTESIAN_POINT('Ctrl Pts',(1.59616958556057,0.477313452032107,8.55227657763063));
#53404=CARTESIAN_POINT('Ctrl Pts',(1.59460567107145,0.482512412327739,8.55264231380213));
#53405=CARTESIAN_POINT('Ctrl Pts',(1.59091220213775,0.494576617973036,8.55349569892178));
#53406=CARTESIAN_POINT('Ctrl Pts',(1.58876361104147,0.501435787905343,8.55398441865805));
#53407=CARTESIAN_POINT('Ctrl Pts',(1.58175079549993,0.523325913759013,8.55555491547915));
#53408=CARTESIAN_POINT('Ctrl Pts',(1.57671728990582,0.538301155009011,8.55664567246056));
#53409=CARTESIAN_POINT('Ctrl Pts',(1.54768511648739,0.620772394225589,8.5627351340626));
#53410=CARTESIAN_POINT('Ctrl Pts',(1.51956728163363,0.686732002454029,8.56791020903149));
#53411=CARTESIAN_POINT('Ctrl Pts',(1.42788868427538,0.868373897026183,8.5827023901046));
#53412=CARTESIAN_POINT('Ctrl Pts',(1.35470673340794,0.978632185031502,8.59230420308492));
#53413=CARTESIAN_POINT('Ctrl Pts',(1.2515199717874,1.10000241085572,8.6033172295377));
#53414=CARTESIAN_POINT('Ctrl Pts',(1.23324927163831,1.12044809431157,8.6051921927104));
#53415=CARTESIAN_POINT('Ctrl Pts',(1.20589098823588,1.14958270926931,8.60789490363158));
#53416=CARTESIAN_POINT('Ctrl Pts',(1.19719738179014,1.15863364570196,8.60873909157199));
#53417=CARTESIAN_POINT('Ctrl Pts',(1.18154392371254,1.17456618303465,8.61023368833256));
#53418=CARTESIAN_POINT('Ctrl Pts',(1.17462422783988,1.18148622183495,8.61088579879288));
#53419=CARTESIAN_POINT('Ctrl Pts',(1.15998754313556,1.19586793283096,8.61224755647325));
#53420=CARTESIAN_POINT('Ctrl Pts',(1.15225858334036,1.20331682412339,8.61295662769277));
#53421=CARTESIAN_POINT('Ctrl Pts',(1.13164177113739,1.2228057629931,8.61482232467038));
#53422=CARTESIAN_POINT('Ctrl Pts',(1.11863357924766,1.23471696604904,8.61597343476391));
#53423=CARTESIAN_POINT('Ctrl Pts',(1.05066066614992,1.29500152160799,8.62186123004472));
#53424=CARTESIAN_POINT('Ctrl Pts',(0.992736350951805,1.33992285693488,8.62645431707515));
#53425=CARTESIAN_POINT('Ctrl Pts',(0.849088366953883,1.43687860847934,8.63715171826821));
#53426=CARTESIAN_POINT('Ctrl Pts',(0.761266730042087,1.48527535553097,8.64316550830717));
#53427=CARTESIAN_POINT('Ctrl Pts',(0.62045662220063,1.5470857425111,8.65271642471071));
#53428=CARTESIAN_POINT('Ctrl Pts',(0.570266633662561,1.56628076522474,8.65610741869753));
#53429=CARTESIAN_POINT('Ctrl Pts',(0.508666407649397,1.58648617841625,8.66035245457467));
#53430=CARTESIAN_POINT('Ctrl Pts',(0.498055284321168,1.5898493091763,8.66108662295507));
#53431=CARTESIAN_POINT('Ctrl Pts',(0.481363079497813,1.59495629877267,8.66224728353454));
#53432=CARTESIAN_POINT('Ctrl Pts',(0.475304181533148,1.59677235102676,8.66266975806586));
#53433=CARTESIAN_POINT('Ctrl Pts',(0.464488884128356,1.59994704451508,8.66342623188712));
#53434=CARTESIAN_POINT('Ctrl Pts',(0.459736568115057,1.60131906697927,8.66375945222289));
#53435=CARTESIAN_POINT('Ctrl Pts',(0.44819707652217,1.60459498655572,8.66457051801326));
#53436=CARTESIAN_POINT('Ctrl Pts',(0.441403907649292,1.60647697651082,8.66504959249903));
#53437=CARTESIAN_POINT('Ctrl Pts',(0.420075782227149,1.61224026353008,8.66655831031604));
#53438=CARTESIAN_POINT('Ctrl Pts',(0.405500538857981,1.61596769884155,8.66759600333793));
#53439=CARTESIAN_POINT('Ctrl Pts',(0.328338507959011,1.63459131952331,8.67311761376156));
#53440=CARTESIAN_POINT('Ctrl Pts',(0.264983670729051,1.6460488947685,8.67774600013249));
#53441=CARTESIAN_POINT('Ctrl Pts',(0.0913068380318652,1.66717097982994,
8.69044302900279));
#53442=CARTESIAN_POINT('Ctrl Pts',(-0.019589679162119,1.6695560050994,8.6985403900644));
#53443=CARTESIAN_POINT('Ctrl Pts',(-0.178644586390325,1.6571154786613,8.70980358869952));
#53444=CARTESIAN_POINT('Ctrl Pts',(-0.227191696465896,1.65116031026339,
8.71319790034189));
#53445=CARTESIAN_POINT('Ctrl Pts',(-0.291323627982365,1.64041057867587,
8.71762489934705));
#53446=CARTESIAN_POINT('Ctrl Pts',(-0.307197039254748,1.63751223926375,
8.71871604486558));
#53447=CARTESIAN_POINT('Ctrl Pts',(-0.333241859470873,1.63236463342919,
8.72049937769125));
#53448=CARTESIAN_POINT('Ctrl Pts',(-0.343438420736708,1.63024982534615,
8.72119577983131));
#53449=CARTESIAN_POINT('Ctrl Pts',(-0.363297034196302,1.62593647955193,
8.7225488597867));
#53450=CARTESIAN_POINT('Ctrl Pts',(-0.372960601221663,1.62374707628679,
8.72320579754822));
#53451=CARTESIAN_POINT('Ctrl Pts',(-0.395806258911788,1.61835638933508,
8.72475562897965));
#53452=CARTESIAN_POINT('Ctrl Pts',(-0.408970049457145,1.61508003335612,
8.7256460815658));
#53453=CARTESIAN_POINT('Ctrl Pts',(-0.453677157490325,1.60337114924446,
8.72866286307849));
#53454=CARTESIAN_POINT('Ctrl Pts',(-0.485013163240443,1.59417203083503,
8.73076460066791));
#53455=CARTESIAN_POINT('Ctrl Pts',(-0.56130059777619,1.56931881607465,8.73586798607704));
#53456=CARTESIAN_POINT('Ctrl Pts',(-0.605890847325255,1.55264828270955,
8.73883889454781));
#53457=CARTESIAN_POINT('Ctrl Pts',(-0.712264135150214,1.50759770288853,
8.74597509660745));
#53458=CARTESIAN_POINT('Ctrl Pts',(-0.773140527237406,1.47730327343718,
8.75009950125815));
#53459=CARTESIAN_POINT('Ctrl Pts',(-0.901620421702202,1.4032442704519,8.75917505766934));
#53460=CARTESIAN_POINT('Ctrl Pts',(-0.968239763119025,1.35813198581288,
8.76412748864292));
#53461=CARTESIAN_POINT('Ctrl Pts',(-1.04372586745412,1.29863051006517,8.77036363760252));
#53462=CARTESIAN_POINT('Ctrl Pts',(-1.05597583350396,1.28868921109926,8.77139701313872));
#53463=CARTESIAN_POINT('Ctrl Pts',(-1.07353696164069,1.2740191951908,8.77291285363845));
#53464=CARTESIAN_POINT('Ctrl Pts',(-1.07896235349659,1.2694277265242,8.77338603804226));
#53465=CARTESIAN_POINT('Ctrl Pts',(-1.08852024776686,1.26123341501842,8.77422867354346));
#53466=CARTESIAN_POINT('Ctrl Pts',(-1.09266458954541,1.25764468370361,8.77459710561739));
#53467=CARTESIAN_POINT('Ctrl Pts',(-1.10121634701381,1.25016523600842,8.77536382144691));
#53468=CARTESIAN_POINT('Ctrl Pts',(-1.10562084751053,1.2462716795018,8.77576228694144));
#53469=CARTESIAN_POINT('Ctrl Pts',(-1.11769482871709,1.23548396217376,8.77686426278881));
#53470=CARTESIAN_POINT('Ctrl Pts',(-1.12532089136046,1.22854191179195,8.77757113776083));
#53471=CARTESIAN_POINT('Ctrl Pts',(-1.14261038103281,1.21250714230473,8.77919777042599));
#53472=CARTESIAN_POINT('Ctrl Pts',(-1.15223051403372,1.20336896688996,8.78012040401094));
#53473=CARTESIAN_POINT('Ctrl Pts',(-1.18243774780598,1.1739807664499,8.7830709971131));
#53474=CARTESIAN_POINT('Ctrl Pts',(-1.20260717994132,1.15331073258552,8.78512179536587));
#53475=CARTESIAN_POINT('Ctrl Pts',(-1.29003666671746,1.05892322041055,8.79434198015223));
#53476=CARTESIAN_POINT('Ctrl Pts',(-1.35113093004777,0.979774794346314,
8.80168058502672));
#53477=CARTESIAN_POINT('Ctrl Pts',(-1.45006038387843,0.824606839956776,
8.81494968166443));
#53478=CARTESIAN_POINT('Ctrl Pts',(-1.48989844303489,0.75023871510445,8.82090514340464));
#53479=CARTESIAN_POINT('Ctrl Pts',(-1.53147013550008,0.656126636541299,
8.82793727613864));
#53480=CARTESIAN_POINT('Ctrl Pts',(-1.53871027605076,0.638962967915996,
8.82920073070951));
#53481=CARTESIAN_POINT('Ctrl Pts',(-1.54974587564725,0.611525579507465,
8.8311912210077));
#53482=CARTESIAN_POINT('Ctrl Pts',(-1.55373033580632,0.601330081544555,
8.83192456056937));
#53483=CARTESIAN_POINT('Ctrl Pts',(-1.5595790154709,0.585918053014193,8.83302386221438));
#53484=CARTESIAN_POINT('Ctrl Pts',(-1.56151810396754,0.580730472766154,
8.8333923134209));
#53485=CARTESIAN_POINT('Ctrl Pts',(-1.5634313003251,0.575533291099453,8.8337599051164));
#53486=CARTESIAN_POINT('Origin',(0.,0.,11.));
#53487=CARTESIAN_POINT('',(-1.56343129957118,0.575533293147481,9.53174555314795));
#53488=CARTESIAN_POINT('',(-1.56343130066142,0.575533290185854,9.34073387093129));
#53489=CARTESIAN_POINT('',(-1.56343130033213,0.575533291080363,11.));
#53490=CARTESIAN_POINT('',(-1.66599968073865,0.00103139649387118,8.67968830643497));
#53491=CARTESIAN_POINT('Ctrl Pts',(-1.56343130066142,0.575533290185854,
9.34073387093129));
#53492=CARTESIAN_POINT('Ctrl Pts',(-1.56097552924839,0.582204372397549,
9.34027245229963));
#53493=CARTESIAN_POINT('Ctrl Pts',(-1.55847696309133,0.588860000088225,
9.33980899614486));
#53494=CARTESIAN_POINT('Ctrl Pts',(-1.55200027408469,0.605782445108938,
9.33862218896235));
#53495=CARTESIAN_POINT('Ctrl Pts',(-1.54796309817374,0.616025528943391,
9.33789586382596));
#53496=CARTESIAN_POINT('Ctrl Pts',(-1.54145760786735,0.63206337039196,9.33674494641135));
#53497=CARTESIAN_POINT('Ctrl Pts',(-1.53905736201547,0.637885643511393,
9.33632426318373));
#53498=CARTESIAN_POINT('Ctrl Pts',(-1.53449753828293,0.648770839018133,
9.33553213366531));
#53499=CARTESIAN_POINT('Ctrl Pts',(-1.53234581057166,0.653836837337789,
9.33516115112599));
#53500=CARTESIAN_POINT('Ctrl Pts',(-1.52723243813707,0.665711809482304,
9.33428615771948));
#53501=CARTESIAN_POINT('Ctrl Pts',(-1.52425033589358,0.67251174090141,9.33378094558348));
#53502=CARTESIAN_POINT('Ctrl Pts',(-1.51423183143901,0.694947443890996,
9.33210076031209));
#53503=CARTESIAN_POINT('Ctrl Pts',(-1.50699976831262,0.710493934059471,
9.33091502970169));
#53504=CARTESIAN_POINT('Ctrl Pts',(-1.48879447707084,0.748100243127719,
9.32799888777758));
#53505=CARTESIAN_POINT('Ctrl Pts',(-1.47756951776062,0.770033219713634,
9.32625724334489));
#53506=CARTESIAN_POINT('Ctrl Pts',(-1.42856753016359,0.860761366010843,
9.31890259846772));
#53507=CARTESIAN_POINT('Ctrl Pts',(-1.38644076361716,0.927090318123248,
9.31316267056956));
#53508=CARTESIAN_POINT('Ctrl Pts',(-1.2781069325487,1.0736721897975,9.29991373636214));
#53509=CARTESIAN_POINT('Ctrl Pts',(-1.20874123586981,1.15120830842992,9.29247029469186));
#53510=CARTESIAN_POINT('Ctrl Pts',(-1.11530646220642,1.23782205251341,9.28369987138508));
#53511=CARTESIAN_POINT('Ctrl Pts',(-1.09767577778892,1.25348311669719,9.28209193535454));
#53512=CARTESIAN_POINT('Ctrl Pts',(-1.07048807889734,1.2766198152194,9.27968102249366));
#53513=CARTESIAN_POINT('Ctrl Pts',(-1.06117275153837,1.28437349884273,9.27886671592648));
#53514=CARTESIAN_POINT('Ctrl Pts',(-1.04423812922288,1.29815913411964,9.27740700976256));
#53515=CARTESIAN_POINT('Ctrl Pts',(-1.0366491803215,1.30422731600888,9.27676016691537));
#53516=CARTESIAN_POINT('Ctrl Pts',(-1.02027179096743,1.31708953866069,9.27537952859756));
#53517=CARTESIAN_POINT('Ctrl Pts',(-1.01146757718169,1.32386280658285,9.27464657710427));
#53518=CARTESIAN_POINT('Ctrl Pts',(-0.987112222542235,1.34221508688822,
9.27264364842932));
#53519=CARTESIAN_POINT('Ctrl Pts',(-0.971425365535203,1.35361172035039,
9.27138076641554));
#53520=CARTESIAN_POINT('Ctrl Pts',(-0.862298646727868,1.43001881210667,
9.26277053203902));
#53521=CARTESIAN_POINT('Ctrl Pts',(-0.762606194274532,1.4855803412894,9.25579963404698));
#53522=CARTESIAN_POINT('Ctrl Pts',(-0.562636883398401,1.57155153941522,
9.24250794712151));
#53523=CARTESIAN_POINT('Ctrl Pts',(-0.463647047354229,1.60354606590308,
9.23620333847865));
#53524=CARTESIAN_POINT('Ctrl Pts',(-0.347639635208347,1.62939544992755,
9.22848191372836));
#53525=CARTESIAN_POINT('Ctrl Pts',(-0.332895574326801,1.63247154521253,
9.22749437401704));
#53526=CARTESIAN_POINT('Ctrl Pts',(-0.311190102548794,1.63669375650073,
9.22602880201785));
#53527=CARTESIAN_POINT('Ctrl Pts',(-0.304259404611052,1.63799631950061,
9.22555908285078));
#53528=CARTESIAN_POINT('Ctrl Pts',(-0.291941038471274,1.64023057038641,
9.224720775648));
#53529=CARTESIAN_POINT('Ctrl Pts',(-0.286556757568334,1.64117979425906,
9.22435317613292));
#53530=CARTESIAN_POINT('Ctrl Pts',(-0.274716889527764,1.64320706691254,
9.22354217336283));
#53531=CARTESIAN_POINT('Ctrl Pts',(-0.268259674255998,1.6442735714106,9.22309816606549));
#53532=CARTESIAN_POINT('Ctrl Pts',(-0.249470187993634,1.64726330914392,
9.22180155440096));
#53533=CARTESIAN_POINT('Ctrl Pts',(-0.237122695424326,1.64908598576885,
9.22094371396321));
#53534=CARTESIAN_POINT('Ctrl Pts',(-0.131572455557443,1.66345691086724,
9.21356796444791));
#53535=CARTESIAN_POINT('Ctrl Pts',(-0.0374912177045608,1.66822988847935,
9.20672016951786));
#53536=CARTESIAN_POINT('Ctrl Pts',(0.177434499990076,1.66093951644877,9.19106593409819));
#53537=CARTESIAN_POINT('Ctrl Pts',(0.297604498869452,1.64366808734118,9.18232697768861));
#53538=CARTESIAN_POINT('Ctrl Pts',(0.435184276323533,1.6082944760408,9.17255518598844));
#53539=CARTESIAN_POINT('Ctrl Pts',(0.455410875248718,1.60268446061466,9.17112350317226));
#53540=CARTESIAN_POINT('Ctrl Pts',(0.487565367210759,1.59310821726686,9.16885461237128));
#53541=CARTESIAN_POINT('Ctrl Pts',(0.499563186286021,1.58938680538606,9.16800960530725));
#53542=CARTESIAN_POINT('Ctrl Pts',(0.520832334594986,1.58252502810981,9.16651410555765));
#53543=CARTESIAN_POINT('Ctrl Pts',(0.530120115213247,1.57943801898851,9.16586190354779));
#53544=CARTESIAN_POINT('Ctrl Pts',(0.549529416410091,1.57279639036083,9.16450049985308));
#53545=CARTESIAN_POINT('Ctrl Pts',(0.55964492280403,1.56922548873373,9.16379186934133));
#53546=CARTESIAN_POINT('Ctrl Pts',(0.586269681980587,1.55953641197448,9.16192858206297));
#53547=CARTESIAN_POINT('Ctrl Pts',(0.602717939829225,1.55325370875977,9.16077941518731));
#53548=CARTESIAN_POINT('Ctrl Pts',(0.686571720539284,1.5196916199843,9.15492592019439));
#53549=CARTESIAN_POINT('Ctrl Pts',(0.752242731717066,1.48827958963831,9.15036306338987));
#53550=CARTESIAN_POINT('Ctrl Pts',(0.904948374433367,1.40253730246508,9.13955036651063));
#53551=CARTESIAN_POINT('Ctrl Pts',(0.989422249527681,1.34427846541188,9.13340146475944));
#53552=CARTESIAN_POINT('Ctrl Pts',(1.10803223265887,1.24520675335075,9.1237919664712));
#53553=CARTESIAN_POINT('Ctrl Pts',(1.14645856650726,1.20992019887443,9.12049540293726));
#53554=CARTESIAN_POINT('Ctrl Pts',(1.1909214241194,1.16506806868546,9.11635886649541));
#53555=CARTESIAN_POINT('Ctrl Pts',(1.19860169207671,1.15716524786349,9.11563189137821));
#53556=CARTESIAN_POINT('Ctrl Pts',(1.21054838922388,1.14462582839083,9.11448016752217));
#53557=CARTESIAN_POINT('Ctrl Pts',(1.21486803951332,1.14004005761475,9.11405933679653));
#53558=CARTESIAN_POINT('Ctrl Pts',(1.22291244692144,1.13140242097695,9.11326709535505));
#53559=CARTESIAN_POINT('Ctrl Pts',(1.22664326107979,1.12735646428281,9.11289615010343));
#53560=CARTESIAN_POINT('Ctrl Pts',(1.23535760088315,1.11781155471716,9.11202146971247));
#53561=CARTESIAN_POINT('Ctrl Pts',(1.24032450030819,1.11229771311548,9.11151653596295));
#53562=CARTESIAN_POINT('Ctrl Pts',(1.25662920186507,1.09395257563365,9.10983824466035));
#53563=CARTESIAN_POINT('Ctrl Pts',(1.26780560005384,1.08098015352847,9.10865416169138));
#53564=CARTESIAN_POINT('Ctrl Pts',(1.29454165676154,1.04896264896547,9.10574291328339));
#53565=CARTESIAN_POINT('Ctrl Pts',(1.30988310620379,1.02974116128939,9.10400456056646));
#53566=CARTESIAN_POINT('Ctrl Pts',(1.37221485467599,0.94799734478871,9.09667301017118));
#53567=CARTESIAN_POINT('Ctrl Pts',(1.41519706964186,0.882546856674632,9.09095354822708));
#53568=CARTESIAN_POINT('Ctrl Pts',(1.5043302913488,0.72345979222794,9.07769768776108));
#53569=CARTESIAN_POINT('Ctrl Pts',(1.54661363699716,0.628010079243398,9.0702274884415));
#53570=CARTESIAN_POINT('Ctrl Pts',(1.58719767665577,0.506868136226347,9.06143270608923));
#53571=CARTESIAN_POINT('Ctrl Pts',(1.59421145315137,0.484357010439733,9.05982501537455));
#53572=CARTESIAN_POINT('Ctrl Pts',(1.60410387652259,0.450059568730554,9.05741439375198));
#53573=CARTESIAN_POINT('Ctrl Pts',(1.60733528397174,0.438379014601159,9.05660013720136));
#53574=CARTESIAN_POINT('Ctrl Pts',(1.61292738480809,0.417271683984568,9.05514048515498));
#53575=CARTESIAN_POINT('Ctrl Pts',(1.61533357395156,0.407857645076977,9.05449364687));
#53576=CARTESIAN_POINT('Ctrl Pts',(1.62031382454423,0.387637074500956,9.05311298040351));
#53577=CARTESIAN_POINT('Ctrl Pts',(1.6228624509457,0.376824716411446,9.05237999654675));
#53578=CARTESIAN_POINT('Ctrl Pts',(1.62956239874507,0.347071117380833,9.05037688107808));
#53579=CARTESIAN_POINT('Ctrl Pts',(1.63349157147053,0.328081253334003,9.0491138468986));
#53580=CARTESIAN_POINT('Ctrl Pts',(1.6583326146526,0.196484154927194,9.04045811069591));
#53581=CARTESIAN_POINT('Ctrl Pts',(1.66791659486275,0.082047197763266,9.03344709681004));
#53582=CARTESIAN_POINT('Ctrl Pts',(1.66367544293997,-0.135452022568592,
9.02016332853214));
#53583=CARTESIAN_POINT('Ctrl Pts',(1.65212362194959,-0.238002012864326,
9.013906030819));
#53584=CARTESIAN_POINT('Ctrl Pts',(1.62810468208955,-0.35363882288545,9.00623432632791));
#53585=CARTESIAN_POINT('Ctrl Pts',(1.62482347168012,-0.368420845372653,
9.00524163515093));
#53586=CARTESIAN_POINT('Ctrl Pts',(1.61971606279495,-0.390033100788841,
9.00376983753511));
#53587=CARTESIAN_POINT('Ctrl Pts',(1.61804702711595,-0.396900185563143,
9.00329914500659));
#53588=CARTESIAN_POINT('Ctrl Pts',(1.61500908333953,-0.409061811656605,
9.00245980126052));
#53589=CARTESIAN_POINT('Ctrl Pts',(1.61365772586271,-0.41436052808787,9.00209214850982));
#53590=CARTESIAN_POINT('Ctrl Pts',(1.6106345928296,-0.425975224798329,9.00128188432054));
#53591=CARTESIAN_POINT('Ctrl Pts',(1.60895176718415,-0.432287972285607,
9.00083867698818));
#53592=CARTESIAN_POINT('Ctrl Pts',(1.60396070169457,-0.450577924351016,
8.99954670646235));
#53593=CARTESIAN_POINT('Ctrl Pts',(1.60055562333102,-0.462527915054894,
8.99869276232351));
#53594=CARTESIAN_POINT('Ctrl Pts',(1.59242801200662,-0.489886451504286,
8.99671684147853));
#53595=CARTESIAN_POINT('Ctrl Pts',(1.58761497161418,-0.50526663081294,8.99559069233664));
#53596=CARTESIAN_POINT('Ctrl Pts',(1.5704945262345,-0.557313937750623,8.99173274178863));
#53597=CARTESIAN_POINT('Ctrl Pts',(1.55713426522695,-0.593619729288246,
8.98896183238573));
#53598=CARTESIAN_POINT('Ctrl Pts',(1.51578073043222,-0.694964263678368,
8.98105453118276));
#53599=CARTESIAN_POINT('Ctrl Pts',(1.48488803090735,-0.758731929874797,
8.97587514990361));
#53600=CARTESIAN_POINT('Ctrl Pts',(1.40234665327102,-0.904631813293935,
8.9637327054364));
#53601=CARTESIAN_POINT('Ctrl Pts',(1.34739485235949,-0.984615545305077,
8.9568459518891));
#53602=CARTESIAN_POINT('Ctrl Pts',(1.27385239428416,-1.07387557405443,8.9489366458727));
#53603=CARTESIAN_POINT('Ctrl Pts',(1.26166618345012,-1.08816688177825,8.94766214835548));
#53604=CARTESIAN_POINT('Ctrl Pts',(1.24190729945677,-1.11056071863938,8.94565115738551));
#53605=CARTESIAN_POINT('Ctrl Pts',(1.23449120327357,-1.1187986099156,8.94490828831998));
#53606=CARTESIAN_POINT('Ctrl Pts',(1.22048140781736,-1.13405194073626,8.94352667464085));
#53607=CARTESIAN_POINT('Ctrl Pts',(1.21390808395396,-1.14108537869739,8.94288711041903));
#53608=CARTESIAN_POINT('Ctrl Pts',(1.19893033492005,-1.1568356207399,8.9414489773473));
#53609=CARTESIAN_POINT('Ctrl Pts',(1.19049104403098,-1.16551863494706,8.94065195376826));
#53610=CARTESIAN_POINT('Ctrl Pts',(1.16482402121885,-1.19135723447147,8.93826663298664));
#53611=CARTESIAN_POINT('Ctrl Pts',(1.14731423111349,-1.20822895739783,8.93669076915745));
#53612=CARTESIAN_POINT('Ctrl Pts',(1.10597504261343,-1.24635233389343,8.93308005135195));
#53613=CARTESIAN_POINT('Ctrl Pts',(1.08189133964565,-1.26731458250074,8.93105670413246));
#53614=CARTESIAN_POINT('Ctrl Pts',(0.99116420409578,-1.34181013541919,8.92369102213435));
#53615=CARTESIAN_POINT('Ctrl Pts',(0.921032512604105,-1.39088502280146,
8.91849267303895));
#53616=CARTESIAN_POINT('Ctrl Pts',(0.769104541649145,-1.4806461231887,8.90771212627441));
#53617=CARTESIAN_POINT('Ctrl Pts',(0.687117499168477,-1.52042757835009,
8.90214308745717));
#53618=CARTESIAN_POINT('Ctrl Pts',(0.587693485241293,-1.55897979432685,
8.89522313080932));
#53619=CARTESIAN_POINT('Ctrl Pts',(0.573002340018647,-1.56443916677728,
8.89419639204224));
#53620=CARTESIAN_POINT('Ctrl Pts',(0.551558033299664,-1.57206551606703,
8.89268854670433));
#53621=CARTESIAN_POINT('Ctrl Pts',(0.544864100988161,-1.57439809381273,
8.89221658495496));
#53622=CARTESIAN_POINT('Ctrl Pts',(0.532969141386325,-1.57845808556889,
8.89137530998448));
#53623=CARTESIAN_POINT('Ctrl Pts',(0.527774180112019,-1.58020266012999,
8.89100700374369));
#53624=CARTESIAN_POINT('Ctrl Pts',(0.51646427182502,-1.58393876516903,8.89020314012698));
#53625=CARTESIAN_POINT('Ctrl Pts',(0.51034646557059,-1.5859205016214,8.88976706016531));
#53626=CARTESIAN_POINT('Ctrl Pts',(0.492842449315931,-1.5914787960523,8.88851610672083));
#53627=CARTESIAN_POINT('Ctrl Pts',(0.481429346634263,-1.59496840153855,
8.88769652774585));
#53628=CARTESIAN_POINT('Ctrl Pts',(0.378905464045456,-1.6251148923719,8.8803052397185));
#53629=CARTESIAN_POINT('Ctrl Pts',(0.285718067041004,-1.64405874460856,
8.87339291019169));
#53630=CARTESIAN_POINT('Ctrl Pts',(0.0711743520457735,-1.66887587811384,
8.85767133657317));
#53631=CARTESIAN_POINT('Ctrl Pts',(-0.0502672840653522,-1.66963943239142,
8.84892944568429));
#53632=CARTESIAN_POINT('Ctrl Pts',(-0.1916103146031,-1.65507760227345,8.83915516420808));
#53633=CARTESIAN_POINT('Ctrl Pts',(-0.212443391405547,-1.65253267961743,
8.83772363724082));
#53634=CARTESIAN_POINT('Ctrl Pts',(-0.245660378469093,-1.64783638199264,
8.83545494364769));
#53635=CARTESIAN_POINT('Ctrl Pts',(-0.258077087228843,-1.6459374214758,
8.83460998008349));
#53636=CARTESIAN_POINT('Ctrl Pts',(-0.280128509403378,-1.64230928934702,
8.83311452982333));
#53637=CARTESIAN_POINT('Ctrl Pts',(-0.289771568967215,-1.64063531246301,
8.83246233419867));
#53638=CARTESIAN_POINT('Ctrl Pts',(-0.309952005264837,-1.63694863274541,
8.83110091649332));
#53639=CARTESIAN_POINT('Ctrl Pts',(-0.320485850233733,-1.63491892786626,
8.83039226582443));
#53640=CARTESIAN_POINT('Ctrl Pts',(-0.348255723880426,-1.62928940429542,
8.82852886300906));
#53641=CARTESIAN_POINT('Ctrl Pts',(-0.365455850017631,-1.6255177859212,
8.82737960201135));
#53642=CARTESIAN_POINT('Ctrl Pts',(-0.453388308813637,-1.60476975934026,
8.82152442476425));
#53643=CARTESIAN_POINT('Ctrl Pts',(-0.523018036583001,-1.58344592300441,
8.81696008384436));
#53644=CARTESIAN_POINT('Ctrl Pts',(-0.686813788657039,-1.52129436653,8.80614379945562));
#53645=CARTESIAN_POINT('Ctrl Pts',(-0.779028959680981,-1.47619854320018,
8.79999284016884));
#53646=CARTESIAN_POINT('Ctrl Pts',(-0.910950862107429,-1.39586219744732,
8.79038821181619));
#53647=CARTESIAN_POINT('Ctrl Pts',(-0.954089843793724,-1.36673851579903,
8.78709917020588));
#53648=CARTESIAN_POINT('Ctrl Pts',(-1.00465158155621,-1.32904226666063,
8.78296873720241));
#53649=CARTESIAN_POINT('Ctrl Pts',(-1.01344583747821,-1.32234854152571,
8.78223970117197));
#53650=CARTESIAN_POINT('Ctrl Pts',(-1.02715305800251,-1.31169827929561,
8.78108542045471));
#53651=CARTESIAN_POINT('Ctrl Pts',(-1.03211144346079,-1.30780034617788,
8.78066412225704));
#53652=CARTESIAN_POINT('Ctrl Pts',(-1.04120919514806,-1.3005643730182,8.77988391453783));
#53653=CARTESIAN_POINT('Ctrl Pts',(-1.04535486635163,-1.29723454960941,
8.77952557802632));
#53654=CARTESIAN_POINT('Ctrl Pts',(-1.04953501971799,-1.29384398078787,
8.77916143284886));
#53655=CARTESIAN_POINT('Ctrl Pts',(-1.0495855613694,-1.29380298098293,8.77915702960156));
#53656=CARTESIAN_POINT('Ctrl Pts',(-1.04968630994534,-1.29372124311757,
8.7791482514342));
#53657=CARTESIAN_POINT('Ctrl Pts',(-1.04973651691065,-1.29368050508796,
8.77914387651603));
#53658=CARTESIAN_POINT('Ctrl Pts',(-1.04983661266962,-1.2935992775302,8.77913515358076));
#53659=CARTESIAN_POINT('Ctrl Pts',(-1.04988650148876,-1.29355878804173,
8.77913080556657));
#53660=CARTESIAN_POINT('Ctrl Pts',(-1.04998597705971,-1.29347804467536,
8.77912213505119));
#53661=CARTESIAN_POINT('Ctrl Pts',(-1.0500355638331,-1.29343779083686,8.77911781255297));
#53662=CARTESIAN_POINT('Ctrl Pts',(-1.05013445099716,-1.29335750620696,
8.7791091917169));
#53663=CARTESIAN_POINT('Ctrl Pts',(-1.05018375141232,-1.2933174754493,8.77910489338149));
#53664=CARTESIAN_POINT('Ctrl Pts',(-1.05028208112494,-1.29323762474549,
8.77909631955391));
#53665=CARTESIAN_POINT('Ctrl Pts',(-1.05033111046096,-1.29319780481849,
8.77909204406267));
#53666=CARTESIAN_POINT('Ctrl Pts',(-1.05042891297235,-1.29311836377819,
8.77908351463211));
#53667=CARTESIAN_POINT('Ctrl Pts',(-1.05047768616211,-1.2930787427006,8.77907926069557));
#53668=CARTESIAN_POINT('Ctrl Pts',(-1.05057499093478,-1.29299968767697,
8.7790707731172));
#53669=CARTESIAN_POINT('Ctrl Pts',(-1.05062352254225,-1.29296025375542,
8.77906653947701));
#53670=CARTESIAN_POINT('Ctrl Pts',(-1.05072035841133,-1.2928815615881,8.77905809125873));
#53671=CARTESIAN_POINT('Ctrl Pts',(-1.05076866268573,-1.29284230337352,
8.77905387668305));
#53672=CARTESIAN_POINT('Ctrl Pts',(-1.0508650577971,-1.29276395143976,8.77904546539097));
#53673=CARTESIAN_POINT('Ctrl Pts',(-1.05091314866018,-1.29272485773818,
8.77904126867559));
#53674=CARTESIAN_POINT('Ctrl Pts',(-1.05642564804173,-1.28824316284837,
8.77856016936964));
#53675=CARTESIAN_POINT('Ctrl Pts',(-1.06186171174713,-1.28376606011976,
8.7780808458362));
#53676=CARTESIAN_POINT('Ctrl Pts',(-1.07368732762639,-1.27390007005085,
8.77702767044892));
#53677=CARTESIAN_POINT('Ctrl Pts',(-1.08006500553454,-1.26849731685145,
8.77645291152172));
#53678=CARTESIAN_POINT('Ctrl Pts',(-1.0975202940165,-1.25348326413653,8.77486169912587));
#53679=CARTESIAN_POINT('Ctrl Pts',(-1.10851180189213,-1.24377354908376,
8.77383932311324));
#53680=CARTESIAN_POINT('Ctrl Pts',(-1.14420401343289,-1.21139471165152,
8.77045556758337));
#53681=CARTESIAN_POINT('Ctrl Pts',(-1.1683477020553,-1.18812597995056,8.76806402850452));
#53682=CARTESIAN_POINT('Ctrl Pts',(-1.27431055831504,-1.07964862868766,
8.75715023320554));
#53683=CARTESIAN_POINT('Ctrl Pts',(-1.34763812731492,-0.986602201158724,
8.7484466510455));
#53684=CARTESIAN_POINT('Ctrl Pts',(-1.44289449031585,-0.835054252666842,
8.73569995999773));
#53685=CARTESIAN_POINT('Ctrl Pts',(-1.47243781013309,-0.781785511323394,
8.73144593816837));
#53686=CARTESIAN_POINT('Ctrl Pts',(-1.50654843293209,-0.711454037462047,
8.7261142363581));
#53687=CARTESIAN_POINT('Ctrl Pts',(-1.51385207947257,-0.695777945047683,
8.72494307836006));
#53688=CARTESIAN_POINT('Ctrl Pts',(-1.52526138858008,-0.67025914716124,
8.72306354635118));
#53689=CARTESIAN_POINT('Ctrl Pts',(-1.5295187879798,-0.660486119609003,
8.72235002634016));
#53690=CARTESIAN_POINT('Ctrl Pts',(-1.53751230917677,-0.641644817431444,
8.72098621082228));
#53691=CARTESIAN_POINT('Ctrl Pts',(-1.54126271775386,-0.632583128515173,
8.72033545332679));
#53692=CARTESIAN_POINT('Ctrl Pts',(-1.54976800137927,-0.611508017821998,
8.71883359915874));
#53693=CARTESIAN_POINT('Ctrl Pts',(-1.55446362358281,-0.599471244126243,
8.71798452042175));
#53694=CARTESIAN_POINT('Ctrl Pts',(-1.56915415568843,-0.56047981383675,
8.71526082019183));
#53695=CARTESIAN_POINT('Ctrl Pts',(-1.57859193186306,-0.533319844770116,
8.71340460488623));
#53696=CARTESIAN_POINT('Ctrl Pts',(-1.61546779329547,-0.417623734153171,
8.70564836649682));
#53697=CARTESIAN_POINT('Ctrl Pts',(-1.63619676418024,-0.327121366869854,
8.69996022469041));
#53698=CARTESIAN_POINT('Ctrl Pts',(-1.66046624743968,-0.157049875223947,
8.68946586476894));
#53699=CARTESIAN_POINT('Ctrl Pts',(-1.66604864137761,-0.0780540079694674,
8.6846626029166));
#53700=CARTESIAN_POINT('Ctrl Pts',(-1.66599968073865,0.00103139649387118,
8.67968830643497));
#53701=CARTESIAN_POINT('Ctrl Pts',(-1.66599967925263,0.00103379404400243,
8.67968815563433));
#53702=CARTESIAN_POINT('Ctrl Pts',(-1.66597648224291,0.0384166857153259,
8.67733685306753));
#53703=CARTESIAN_POINT('Ctrl Pts',(-1.6646950543706,0.0757857438253784,
8.6749486588933));
#53704=CARTESIAN_POINT('Ctrl Pts',(-1.66161369494957,0.121079560033358,
8.6719742140175));
#53705=CARTESIAN_POINT('Ctrl Pts',(-1.66101153588352,0.129077506502333,
8.67144595417797));
#53706=CARTESIAN_POINT('Ctrl Pts',(-1.65988110049662,0.142770597757506,
8.67053585219587));
#53707=CARTESIAN_POINT('Ctrl Pts',(-1.65938119599999,0.148468028065719,
8.67015548892855));
#53708=CARTESIAN_POINT('Ctrl Pts',(-1.65837961712452,0.159245417429015,
8.66943259787395));
#53709=CARTESIAN_POINT('Ctrl Pts',(-1.65788390923652,0.164325893963225,
8.66909039944385));
#53710=CARTESIAN_POINT('Ctrl Pts',(-1.65684510346844,0.1744890590459,8.66840285312853));
#53711=CARTESIAN_POINT('Ctrl Pts',(-1.65630194728617,0.179571674368825,
8.66805750879186));
#53712=CARTESIAN_POINT('Ctrl Pts',(-1.65495319390699,0.1916656853521,8.66723231936529));
#53713=CARTESIAN_POINT('Ctrl Pts',(-1.65412642417294,0.198674551342065,
8.66675133369868));
#53714=CARTESIAN_POINT('Ctrl Pts',(-1.65102180449209,0.223629741822775,
8.66502942676835));
#53715=CARTESIAN_POINT('Ctrl Pts',(-1.64849630276128,0.241543234602649,
8.66377615091533));
#53716=CARTESIAN_POINT('Ctrl Pts',(-1.63808689301534,0.307579550393764,
8.659100681074));
#53717=CARTESIAN_POINT('Ctrl Pts',(-1.62838346383068,0.355387628171913,
8.65560720346379));
#53718=CARTESIAN_POINT('Ctrl Pts',(-1.60201257983422,0.461251642266212,
8.64771584932469));
#53719=CARTESIAN_POINT('Ctrl Pts',(-1.58426157560517,0.518948008136952,
8.64330847460035));
#53720=CARTESIAN_POINT('Ctrl Pts',(-1.56343135626508,0.575533139138958,
8.63893242883258));
#53721=CARTESIAN_POINT('',(-1.66599975036832,-0.00128669572401095,8.8706297405923));
#53722=CARTESIAN_POINT('Ctrl Pts',(-1.5634313003251,0.575533291099453,8.8337599051164));
#53723=CARTESIAN_POINT('Ctrl Pts',(-1.56488277523164,0.571590371835501,
8.8340387840301));
#53724=CARTESIAN_POINT('Ctrl Pts',(-1.56631934733467,0.567641926262001,
8.83431716827669));
#53725=CARTESIAN_POINT('Ctrl Pts',(-1.57192654351643,0.55204707472868,8.83541323209833));
#53726=CARTESIAN_POINT('Ctrl Pts',(-1.57598240674274,0.540359600935614,
8.83622710063096));
#53727=CARTESIAN_POINT('Ctrl Pts',(-1.58806055678282,0.504261679637931,
8.83871852670838));
#53728=CARTESIAN_POINT('Ctrl Pts',(-1.5956488675341,0.479709265922574,8.84038190946538));
#53729=CARTESIAN_POINT('Ctrl Pts',(-1.61204382517528,0.421959319299,8.84422996185352));
#53730=CARTESIAN_POINT('Ctrl Pts',(-1.62039813340751,0.388645180678364,
8.84640078825903));
#53731=CARTESIAN_POINT('Ctrl Pts',(-1.65325862731819,0.23801619464825,8.85604619456224));
#53732=CARTESIAN_POINT('Ctrl Pts',(-1.66609189323001,0.118533972871092,
8.86321239120117));
#53733=CARTESIAN_POINT('Ctrl Pts',(-1.66599950474116,-0.00128460196485134,
8.8706291825431));
#53734=CARTESIAN_POINT('Ctrl Pts',(-1.66599950310516,-0.00128672194783298,
8.87062931377045));
#53735=CARTESIAN_POINT('Ctrl Pts',(-1.66596827752896,-0.041716431351172,
8.87313192108214));
#53736=CARTESIAN_POINT('Ctrl Pts',(-1.66446536543592,-0.0821296462730489,
8.87566262957749));
#53737=CARTESIAN_POINT('Ctrl Pts',(-1.66002256804847,-0.142414878799788,
8.8795327181488));
#53738=CARTESIAN_POINT('Ctrl Pts',(-1.65819112512869,-0.162354659756153,
8.88082843616167));
#53739=CARTESIAN_POINT('Ctrl Pts',(-1.65515491289895,-0.189942131585233,
8.8826488498797));
#53740=CARTESIAN_POINT('Ctrl Pts',(-1.65425545900996,-0.197622543984168,
8.88315864842651));
#53741=CARTESIAN_POINT('Ctrl Pts',(-1.65261124523688,-0.210863813782305,
8.88404315577053));
#53742=CARTESIAN_POINT('Ctrl Pts',(-1.65189179360435,-0.21642776119652,
8.88441653300406));
#53743=CARTESIAN_POINT('Ctrl Pts',(-1.65040124799167,-0.227514429378216,
8.8851641229737));
#53744=CARTESIAN_POINT('Ctrl Pts',(-1.64963049834339,-0.233037149421823,
8.88553831843663));
#53745=CARTESIAN_POINT('Ctrl Pts',(-1.64796278557865,-0.2445639165712,8.88632323048602));
#53746=CARTESIAN_POINT('Ctrl Pts',(-1.64706072011261,-0.250567023437197,
8.88673420589282));
#53747=CARTESIAN_POINT('Ctrl Pts',(-1.64454581597392,-0.266702699382268,
8.88784453008086));
#53748=CARTESIAN_POINT('Ctrl Pts',(-1.6428721790373,-0.276825325393903,
8.88854710997405));
#53749=CARTESIAN_POINT('Ctrl Pts',(-1.63452887836497,-0.32454484399152,
8.8918856384151));
#53750=CARTESIAN_POINT('Ctrl Pts',(-1.62666192085239,-0.361917804472079,
8.89457787022709));
#53751=CARTESIAN_POINT('Ctrl Pts',(-1.60236290832557,-0.46042828696624,
8.90182702534621));
#53752=CARTESIAN_POINT('Ctrl Pts',(-1.58371867614595,-0.520956425430241,
8.9064386797093));
#53753=CARTESIAN_POINT('Ctrl Pts',(-1.54265689778955,-0.63146491765145,
8.9150194758297));
#53754=CARTESIAN_POINT('Ctrl Pts',(-1.52112975916639,-0.681691295193066,
8.91898544338394));
#53755=CARTESIAN_POINT('Ctrl Pts',(-1.46526640162141,-0.796141765248175,
8.92811444013505));
#53756=CARTESIAN_POINT('Ctrl Pts',(-1.42910869966066,-0.859359230160901,
8.93322584024351));
#53757=CARTESIAN_POINT('Ctrl Pts',(-1.37920481484813,-0.934697876844317,
8.93939281986397));
#53758=CARTESIAN_POINT('Ctrl Pts',(-1.3692486848802,-0.94922290456683,8.9405858022141));
#53759=CARTESIAN_POINT('Ctrl Pts',(-1.35285907409059,-0.972339143184272,
8.94249160935605));
#53760=CARTESIAN_POINT('Ctrl Pts',(-1.34656983465826,-0.981030465081007,
8.94320984552036));
#53761=CARTESIAN_POINT('Ctrl Pts',(-1.3343828779837,-0.997534024008357,
8.94457717549616));
#53762=CARTESIAN_POINT('Ctrl Pts',(-1.32849942968826,-1.0053561888223,8.94522678279268));
#53763=CARTESIAN_POINT('Ctrl Pts',(-1.31490861998533,-1.02309779741006,
8.94670398731371));
#53764=CARTESIAN_POINT('Ctrl Pts',(-1.30715726093793,-1.03298290959966,
8.94752981303348));
#53765=CARTESIAN_POINT('Ctrl Pts',(-1.28615868963339,-1.05914695290626,
8.9497239253404));
#53766=CARTESIAN_POINT('Ctrl Pts',(-1.27271417548612,-1.07526514558967,
8.95108433046532));
#53767=CARTESIAN_POINT('Ctrl Pts',(-1.17967520622907,-1.18261585190103,
8.96021730129166));
#53768=CARTESIAN_POINT('Ctrl Pts',(-1.09064493160751,-1.2651922104763,8.96756981279484));
#53769=CARTESIAN_POINT('Ctrl Pts',(-0.91714083881409,-1.3940742640748,8.98077707195054));
#53770=CARTESIAN_POINT('Ctrl Pts',(-0.836139311024954,-1.44411086642029,
8.9866020385928));
#53771=CARTESIAN_POINT('Ctrl Pts',(-0.740733417825566,-1.4923173029462,
8.99359176309791));
#53772=CARTESIAN_POINT('Ctrl Pts',(-0.730081271344885,-1.49755742674096,
8.99437396919977));
#53773=CARTESIAN_POINT('Ctrl Pts',(-0.713585826375973,-1.50545423557928,
8.99558941361581));
#53774=CARTESIAN_POINT('Ctrl Pts',(-0.70778139567752,-1.50819185765991,
8.99601788941611));
#53775=CARTESIAN_POINT('Ctrl Pts',(-0.696989250214719,-1.5132058828545,
8.99681626862363));
#53776=CARTESIAN_POINT('Ctrl Pts',(-0.692005941441851,-1.51549128423895,
8.99718561972599));
#53777=CARTESIAN_POINT('Ctrl Pts',(-0.680535372881636,-1.52068344485008,
8.99803733820598));
#53778=CARTESIAN_POINT('Ctrl Pts',(-0.674040715602689,-1.52357331371274,
8.99852069139764));
#53779=CARTESIAN_POINT('Ctrl Pts',(-0.653067894642985,-1.53274505543102,
9.00008465279578));
#53780=CARTESIAN_POINT('Ctrl Pts',(-0.638519394461202,-1.53886257270924,
9.00117427039388));
#53781=CARTESIAN_POINT('Ctrl Pts',(-0.55055313685452,-1.57438948868897,
9.00778155852132));
#53782=CARTESIAN_POINT('Ctrl Pts',(-0.475210441366305,-1.5987443886253,
9.01351478732295));
#53783=CARTESIAN_POINT('Ctrl Pts',(-0.334183109827049,-1.63347970724582,
9.02408374086524));
#53784=CARTESIAN_POINT('Ctrl Pts',(-0.269045756079804,-1.64546329554329,
9.02890492484022));
#53785=CARTESIAN_POINT('Ctrl Pts',(-0.154346706218855,-1.65956992508093,
9.03719564964192));
#53786=CARTESIAN_POINT('Ctrl Pts',(-0.105080082227951,-1.66341641620293,
9.04069465968755));
#53787=CARTESIAN_POINT('Ctrl Pts',(-0.0222065774932575,-1.66618927387045,
9.04646489783672));
#53788=CARTESIAN_POINT('Ctrl Pts',(0.011326341424732,-1.66629883936254,
9.04876832701811));
#53789=CARTESIAN_POINT('Ctrl Pts',(0.0585375289211347,-1.66502764647522,
9.05196916792454));
#53790=CARTESIAN_POINT('Ctrl Pts',(0.0722284151591141,-1.66448994630165,
9.05289242005591));
#53791=CARTESIAN_POINT('Ctrl Pts',(0.0958297647904633,-1.66327126199123,
9.05447582700435));
#53792=CARTESIAN_POINT('Ctrl Pts',(0.105743457963293,-1.66267043133611,
9.05513844733031));
#53793=CARTESIAN_POINT('Ctrl Pts',(0.125996365850009,-1.66126110316037,
9.05648728401805));
#53794=CARTESIAN_POINT('Ctrl Pts',(0.136334603932253,-1.66044464559428,
9.05717322129421));
#53795=CARTESIAN_POINT('Ctrl Pts',(0.162532665486372,-1.65812933456241,
9.05890529161773));
#53796=CARTESIAN_POINT('Ctrl Pts',(0.178380085756071,-1.65649942084418,
9.05994729348267));
#53797=CARTESIAN_POINT('Ctrl Pts',(0.24084040071879,-1.64916857553735,9.06403424964974));
#53798=CARTESIAN_POINT('Ctrl Pts',(0.287229185158592,-1.64172503859499,
9.0670248555627));
#53799=CARTESIAN_POINT('Ctrl Pts',(0.443283019040145,-1.60986620198611,
9.07701773753384));
#53800=CARTESIAN_POINT('Ctrl Pts',(0.550765196775811,-1.57633345343412,
9.08376637265435));
#53801=CARTESIAN_POINT('Ctrl Pts',(0.713778368484908,-1.50674910042821,
9.09467185701371));
#53802=CARTESIAN_POINT('Ctrl Pts',(0.771951086832096,-1.4777895876209,9.09871745373136));
#53803=CARTESIAN_POINT('Ctrl Pts',(0.841387873409657,-1.43800233467586,
9.10391613433313));
#53804=CARTESIAN_POINT('Ctrl Pts',(0.854393533742128,-1.4303132238541,9.10490669395065));
#53805=CARTESIAN_POINT('Ctrl Pts',(0.873321126875506,-1.418772733341,9.10637593050457));
#53806=CARTESIAN_POINT('Ctrl Pts',(0.879326425696656,-1.41505861789301,
9.10684623545486));
#53807=CARTESIAN_POINT('Ctrl Pts',(0.889499328596857,-1.40867719040407,
9.10765033560148));
#53808=CARTESIAN_POINT('Ctrl Pts',(0.893678954296769,-1.40602930556266,
9.10798286382665));
#53809=CARTESIAN_POINT('Ctrl Pts',(0.903168283078739,-1.39995819994274,
9.10874283107237));
#53810=CARTESIAN_POINT('Ctrl Pts',(0.908470229525741,-1.39652345053351,
9.10917100979413));
#53811=CARTESIAN_POINT('Ctrl Pts',(0.923030779722948,-1.38697271322956,
9.11035648323831));
#53812=CARTESIAN_POINT('Ctrl Pts',(0.932247814456555,-1.38079438130641,
9.11111766848605));
#53813=CARTESIAN_POINT('Ctrl Pts',(0.984964663819151,-1.34468898717841,
9.11553055201172));
#53814=CARTESIAN_POINT('Ctrl Pts',(1.02707989540479,-1.31280219196893,9.11928988104042));
#53815=CARTESIAN_POINT('Ctrl Pts',(1.1452619041665,-1.21415138715253,9.13039123268855));
#53816=CARTESIAN_POINT('Ctrl Pts',(1.21685824025075,-1.14238617258293,9.13782495381783));
#53817=CARTESIAN_POINT('Ctrl Pts',(1.32821983473003,-1.00833197065608,9.1503196514515));
#53818=CARTESIAN_POINT('Ctrl Pts',(1.37119046048659,-0.949073587826089,
9.15545798478568));
#53819=CARTESIAN_POINT('Ctrl Pts',(1.41952163983021,-0.87225290491955,9.16165193191844));
#53820=CARTESIAN_POINT('Ctrl Pts',(1.42867276334667,-0.857182006831354,
9.16284643317738));
#53821=CARTESIAN_POINT('Ctrl Pts',(1.44300723280871,-0.832707217998786,
9.1647540669951));
#53822=CARTESIAN_POINT('Ctrl Pts',(1.4483417072764,-0.823393886990113,9.16547262959952));
#53823=CARTESIAN_POINT('Ctrl Pts',(1.45836756766491,-0.805491034420518,
9.16684020614021));
#53824=CARTESIAN_POINT('Ctrl Pts',(1.46307397370014,-0.796910486442735,
9.16748973710673));
#53825=CARTESIAN_POINT('Ctrl Pts',(1.47364360378934,-0.777231030880079,
9.16896625766983));
#53826=CARTESIAN_POINT('Ctrl Pts',(1.47945759650534,-0.766106246439847,
9.16979148166983));
#53827=CARTESIAN_POINT('Ctrl Pts',(1.49464013563545,-0.736237675511792,
9.17198285646175));
#53828=CARTESIAN_POINT('Ctrl Pts',(1.5037819132853,-0.71738070082642,9.17334115767906));
#53829=CARTESIAN_POINT('Ctrl Pts',(1.56355141408682,-0.587926153673739,
9.18250854084999));
#53830=CARTESIAN_POINT('Ctrl Pts',(1.60229199090032,-0.472244024635995,
9.18989299383956));
#53831=CARTESIAN_POINT('Ctrl Pts',(1.6481244794471,-0.261075211193354,9.20309809971954));
#53832=CARTESIAN_POINT('Ctrl Pts',(1.66026885543512,-0.167262528521581,
9.20888764052188));
#53833=CARTESIAN_POINT('Ctrl Pts',(1.66492499714733,-0.0610181047416712,
9.21584062516424));
#53834=CARTESIAN_POINT('Ctrl Pts',(1.66531939335526,-0.0490892375292942,
9.21662696999309));
#53835=CARTESIAN_POINT('Ctrl Pts',(1.6657290151657,-0.0307279760604022,
9.21784749257201));
#53836=CARTESIAN_POINT('Ctrl Pts',(1.6658352192432,-0.0242977228723366,
9.21827684516681));
#53837=CARTESIAN_POINT('Ctrl Pts',(1.66596296602662,-0.012386820105187,
9.21907596119453));
#53838=CARTESIAN_POINT('Ctrl Pts',(1.66599469829919,-0.00690648494370706,
9.21944516253258));
#53839=CARTESIAN_POINT('Ctrl Pts',(1.66600545811108,0.00566307078343564,
9.22029539091038));
#53840=CARTESIAN_POINT('Ctrl Pts',(1.66596627718651,0.0127520784019295,
9.22077739101599));
#53841=CARTESIAN_POINT('Ctrl Pts',(1.66569519640985,0.0355130745999442,
9.22233249587555));
#53842=CARTESIAN_POINT('Ctrl Pts',(1.66528738272876,0.0511815829638037,
9.22341447316345));
#53843=CARTESIAN_POINT('Ctrl Pts',(1.66100514156942,0.15782929327989,9.23084673964826));
#53844=CARTESIAN_POINT('Ctrl Pts',(1.64989827418297,0.248356240164162,9.23748291685502));
#53845=CARTESIAN_POINT('Ctrl Pts',(1.61415134764611,0.421147951123315,9.25032683511329));
#53846=CARTESIAN_POINT('Ctrl Pts',(1.59044183670801,0.50333658274887,9.25651678434946));
#53847=CARTESIAN_POINT('Ctrl Pts',(1.54935820118495,0.613240047714823,9.26478690489164));
#53848=CARTESIAN_POINT('Ctrl Pts',(1.53732823011057,0.64280349490545,9.26701196158952));
#53849=CARTESIAN_POINT('Ctrl Pts',(1.51465189834327,0.694245183325159,9.27088403957266));
#53850=CARTESIAN_POINT('Ctrl Pts',(1.50436206658491,0.716269242928525,9.27254199350692));
#53851=CARTESIAN_POINT('Ctrl Pts',(1.48822989608377,0.748915454057452,9.2750010974797));
#53852=CARTESIAN_POINT('Ctrl Pts',(1.48274802130399,0.759711063277453,9.27581455352803));
#53853=CARTESIAN_POINT('Ctrl Pts',(1.4726968004174,0.778981907827375,9.27726742712968));
#53854=CARTESIAN_POINT('Ctrl Pts',(1.46817079921307,0.787479009051319,9.27790832869274));
#53855=CARTESIAN_POINT('Ctrl Pts',(1.45827522156715,0.805675036706466,9.27928163848624));
#53856=CARTESIAN_POINT('Ctrl Pts',(1.45288195594977,0.815360606526759,9.2800131685031));
#53857=CARTESIAN_POINT('Ctrl Pts',(1.43808997055515,0.841312143543874,9.28197521661461));
#53858=CARTESIAN_POINT('Ctrl Pts',(1.42851197624656,0.857474469820867,9.28319927027255));
#53859=CARTESIAN_POINT('Ctrl Pts',(1.3678818172197,0.955947843273953,9.29067774583326));
#53860=CARTESIAN_POINT('Ctrl Pts',(1.31000320731597,1.03384333305896,9.29666871022893));
#53861=CARTESIAN_POINT('Ctrl Pts',(1.1986497301295,1.15922830839413,9.30693048243229));
#53862=CARTESIAN_POINT('Ctrl Pts',(1.1482962230191,1.20912637986913,9.31122428115046));
#53863=CARTESIAN_POINT('Ctrl Pts',(1.06579495785619,1.28106620524842,9.31800975750277));
#53864=CARTESIAN_POINT('Ctrl Pts',(1.03579429938842,1.3054421821606,9.32043256191278));
#53865=CARTESIAN_POINT('Ctrl Pts',(0.992128740573799,1.33846778368993,9.32394018100295));
#53866=CARTESIAN_POINT('Ctrl Pts',(0.9791423008097,1.34799694326833,9.32498115635007));
#53867=CARTESIAN_POINT('Ctrl Pts',(0.955900562946801,1.36453816158531,9.32684429467267));
#53868=CARTESIAN_POINT('Ctrl Pts',(0.945700992093933,1.37162673191366,9.32766196584529));
#53869=CARTESIAN_POINT('Ctrl Pts',(0.930017899544425,1.38226820125471,9.32892088185917));
#53870=CARTESIAN_POINT('Ctrl Pts',(0.924590894567865,1.3859041625341,9.32935681560543));
#53871=CARTESIAN_POINT('Ctrl Pts',(0.914581413095402,1.39252531348341,9.33016166536108));
#53872=CARTESIAN_POINT('Ctrl Pts',(0.910005449860086,1.39551997054404,9.33052994684436));
#53873=CARTESIAN_POINT('Ctrl Pts',(0.899480896795459,1.40233380014066,9.33137771980889));
#53874=CARTESIAN_POINT('Ctrl Pts',(0.893522705263631,1.40613766798398,9.33185817494019));
#53875=CARTESIAN_POINT('Ctrl Pts',(0.874718789433595,1.41797481868144,9.33337563686172));
#53876=CARTESIAN_POINT('Ctrl Pts',(0.861788001082651,1.42587059298853,9.33442082193067));
#53877=CARTESIAN_POINT('Ctrl Pts',(0.760188292474761,1.48602240282723,9.3426354482507));
#53878=CARTESIAN_POINT('Ctrl Pts',(0.666964112237238,1.53013209657131,9.35017212228367));
#53879=CARTESIAN_POINT('Ctrl Pts',(0.462629659926865,1.60457330099689,9.36598732243035));
#53880=CARTESIAN_POINT('Ctrl Pts',(0.351206968569368,1.63258829555905,9.37420138646117));
#53881=CARTESIAN_POINT('Ctrl Pts',(0.218580504684241,1.65171261501591,9.38337040615611));
#53882=CARTESIAN_POINT('Ctrl Pts',(0.199340775993966,1.65414488778328,9.3846868157456));
#53883=CARTESIAN_POINT('Ctrl Pts',(0.169018615241091,1.65744143513433,9.38674080516317));
#53884=CARTESIAN_POINT('Ctrl Pts',(0.157963032168888,1.65853160778333,9.38748539486287));
#53885=CARTESIAN_POINT('Ctrl Pts',(0.137218127792181,1.66036791183671,9.38887477288967));
#53886=CARTESIAN_POINT('Ctrl Pts',(0.127531638575733,1.6611400017016,9.38952034674685));
#53887=CARTESIAN_POINT('Ctrl Pts',(0.105749685260113,1.66268454160339,9.39096518903091));
#53888=CARTESIAN_POINT('Ctrl Pts',(0.0936513480057222,1.66340984690926,
9.39176295281699));
#53889=CARTESIAN_POINT('Ctrl Pts',(0.0579973689619847,1.66515710078907,
9.39410082797416));
#53890=CARTESIAN_POINT('Ctrl Pts',(0.0344261075203546,1.66581115305704,
9.39562950151584));
#53891=CARTESIAN_POINT('Ctrl Pts',(-0.0931665243769141,1.666641971733,9.40382669167687));
#53892=CARTESIAN_POINT('Ctrl Pts',(-0.197019943145331,1.65757714399507,
9.41020115579815));
#53893=CARTESIAN_POINT('Ctrl Pts',(-0.376404831263378,1.62481058165997,
9.42133739974519));
#53894=CARTESIAN_POINT('Ctrl Pts',(-0.452356424515242,1.60532301222424,
9.42610032771416));
#53895=CARTESIAN_POINT('Ctrl Pts',(-0.549997666377681,1.57278867310622,
9.43259134415604));
#53896=CARTESIAN_POINT('Ctrl Pts',(-0.573169050380657,1.56449313046206,
9.43416035289995));
#53897=CARTESIAN_POINT('Ctrl Pts',(-0.612144930537602,1.54955738932823,
9.43686191641999));
#53898=CARTESIAN_POINT('Ctrl Pts',(-0.628046645861519,1.54318076501461,
9.43798210704558));
#53899=CARTESIAN_POINT('Ctrl Pts',(-0.650692765361467,1.53369163361736,
9.43960723724647));
#53900=CARTESIAN_POINT('Ctrl Pts',(-0.657519686942117,1.53077723983599,
9.44010108410668));
#53901=CARTESIAN_POINT('Ctrl Pts',(-0.669374350513616,1.52562258582735,
9.4409658846489));
#53902=CARTESIAN_POINT('Ctrl Pts',(-0.674410829330468,1.52340287769807,
9.4413356045612));
#53903=CARTESIAN_POINT('Ctrl Pts',(-0.685188176393028,1.51858909737181,
9.44213183274501));
#53904=CARTESIAN_POINT('Ctrl Pts',(-0.690925264065114,1.51598745374315,
9.4425587671352));
#53905=CARTESIAN_POINT('Ctrl Pts',(-0.706655043245815,1.50874650864917,
9.44373753369747));
#53906=CARTESIAN_POINT('Ctrl Pts',(-0.716616472934998,1.50404062179375,
9.44449318776226));
#53907=CARTESIAN_POINT('Ctrl Pts',(-0.773410038662576,1.47651845310577,
9.44885111666423));
#53908=CARTESIAN_POINT('Ctrl Pts',(-0.819193944520505,1.4516163380312,9.45255833517449));
#53909=CARTESIAN_POINT('Ctrl Pts',(-0.951108913733647,1.37163740928306,
9.46367847866774));
#53910=CARTESIAN_POINT('Ctrl Pts',(-1.03343357253797,1.31073039215437,9.47118957482571));
#53911=CARTESIAN_POINT('Ctrl Pts',(-1.16407225991808,1.19407440973592,9.48374538986823));
#53912=CARTESIAN_POINT('Ctrl Pts',(-1.21524228771502,1.14195742025453,9.4888720729303));
#53913=CARTESIAN_POINT('Ctrl Pts',(-1.27432957321312,1.07328962588066,9.49505435778117));
#53914=CARTESIAN_POINT('Ctrl Pts',(-1.28561026739359,1.05975127457879,9.49624820385952));
#53915=CARTESIAN_POINT('Ctrl Pts',(-1.30341175859014,1.03768440712373,9.49815504974702));
#53916=CARTESIAN_POINT('Ctrl Pts',(-1.31006836520651,1.02926771494205,9.49887347154413));
#53917=CARTESIAN_POINT('Ctrl Pts',(-1.32263981563531,1.01305266292917,9.50024094163243));
#53918=CARTESIAN_POINT('Ctrl Pts',(-1.32856814245789,1.00526537669971,9.50089050542535));
#53919=CARTESIAN_POINT('Ctrl Pts',(-1.34194470406696,0.987369261748859,
9.50236732053446));
#53920=CARTESIAN_POINT('Ctrl Pts',(-1.34934802866682,0.977227486159524,
9.50319280370947));
#53921=CARTESIAN_POINT('Ctrl Pts',(-1.36880659635929,0.949928497954312,
9.50538535745504));
#53922=CARTESIAN_POINT('Ctrl Pts',(-1.38065401681838,0.932625432944944,
9.50674456472587));
#53923=CARTESIAN_POINT('Ctrl Pts',(-1.4588509010499,0.813662260537325,9.515897348041));
#53924=CARTESIAN_POINT('Ctrl Pts',(-1.51424471650612,0.705236852634478,
9.52326824179325));
#53925=CARTESIAN_POINT('Ctrl Pts',(-1.55941714307736,0.586350974627343,
9.53103998379564));
#53926=CARTESIAN_POINT('Ctrl Pts',(-1.56143835103431,0.580947120910484,
9.53139267944501));
#53927=CARTESIAN_POINT('Ctrl Pts',(-1.56343129957118,0.575533293147481,
9.53174555314795));
#53928=CARTESIAN_POINT('Origin',(0.,0.,11.));
#53929=CARTESIAN_POINT('',(-1.56343128570986,0.575533330801617,10.2310772794004));
#53930=CARTESIAN_POINT('',(-1.56343130417499,0.575533280641269,10.0383108307813));
#53931=CARTESIAN_POINT('',(-1.56343130033213,0.575533291080363,11.));
#53932=CARTESIAN_POINT('Ctrl Pts',(-1.56343130417499,0.575533280641269,
10.0383108307813));
#53933=CARTESIAN_POINT('Ctrl Pts',(-1.53523060277161,0.652140248225498,
10.0332234667563));
#53934=CARTESIAN_POINT('Ctrl Pts',(-1.50143364965884,0.726581757822608,
10.0282692374323));
#53935=CARTESIAN_POINT('Ctrl Pts',(-1.43399751588061,0.850116516093578,
10.0196617533966));
#53936=CARTESIAN_POINT('Ctrl Pts',(-1.40295051330593,0.900430953212348,
10.016032026659));
#53937=CARTESIAN_POINT('Ctrl Pts',(-1.34951857765154,0.977528270062683,
10.0101044793621));
#53938=CARTESIAN_POINT('Ctrl Pts',(-1.32885187559289,1.00544229460194,10.0078755641635));
#53939=CARTESIAN_POINT('Ctrl Pts',(-1.30135426628126,1.04025285934982,10.0049591657919));
#53940=CARTESIAN_POINT('Ctrl Pts',(-1.29531317288898,1.04776558014819,10.0043212960743));
#53941=CARTESIAN_POINT('Ctrl Pts',(-1.28544862983115,1.05981745454892,10.0032834797046));
#53942=CARTESIAN_POINT('Ctrl Pts',(-1.28166542414749,1.06438947508603,10.0028863348848));
#53943=CARTESIAN_POINT('Ctrl Pts',(-1.27427723331173,1.07322163470143,10.002112218223));
#53944=CARTESIAN_POINT('Ctrl Pts',(-1.27067514265848,1.07748402440607,10.0017354490756));
#53945=CARTESIAN_POINT('Ctrl Pts',(-1.26256192767033,1.08698721046191,10.0008884182401));
#53946=CARTESIAN_POINT('Ctrl Pts',(-1.25803945541209,1.09221817478157,10.000417352455));
#53947=CARTESIAN_POINT('Ctrl Pts',(-1.24213630585236,1.11038290737068,9.99876508867047));
#53948=CARTESIAN_POINT('Ctrl Pts',(-1.2305881219801,1.12316767219214,9.99757275236365));
#53949=CARTESIAN_POINT('Ctrl Pts',(-1.11986467331639,1.24198979119828,9.98622853174259));
#53950=CARTESIAN_POINT('Ctrl Pts',(-1.00742779980078,1.33481321196356,9.97542540082165));
#53951=CARTESIAN_POINT('Ctrl Pts',(-0.823273821872255,1.45016389535073,
9.9598547236061));
#53952=CARTESIAN_POINT('Ctrl Pts',(-0.759740027865684,1.48443684902757,
9.95478966692114));
#53953=CARTESIAN_POINT('Ctrl Pts',(-0.678205154310113,1.52180893794462,
9.94866918414366));
#53954=CARTESIAN_POINT('Ctrl Pts',(-0.662118495821922,1.52887665083948,
9.94747889008192));
#53955=CARTESIAN_POINT('Ctrl Pts',(-0.636041914962719,1.53984466078429,
9.94557634071355));
#53956=CARTESIAN_POINT('Ctrl Pts',(-0.626121262975809,1.54390513642291,
9.94485870680185));
#53957=CARTESIAN_POINT('Ctrl Pts',(-0.607066858659145,1.55149014076746,
9.94349187424011));
#53958=CARTESIAN_POINT('Ctrl Pts',(-0.597939913649682,1.5550304480697,9.94284216828926));
#53959=CARTESIAN_POINT('Ctrl Pts',(-0.577016984100031,1.56293492329162,
9.94136385453368));
#53960=CARTESIAN_POINT('Ctrl Pts',(-0.565201630303103,1.56724640880432,
9.94053702829906));
#53961=CARTESIAN_POINT('Ctrl Pts',(-0.52733045803624,1.58058181247636,9.93791123280812));
#53962=CARTESIAN_POINT('Ctrl Pts',(-0.501098149736979,1.58909315731782,
9.93612907350848));
#53963=CARTESIAN_POINT('Ctrl Pts',(-0.348436678416387,1.63446910767721,
9.92594284870366));
#53964=CARTESIAN_POINT('Ctrl Pts',(-0.218207106765685,1.65689033470997,
9.91802481707132));
#53965=CARTESIAN_POINT('Ctrl Pts',(-0.0151991641739799,1.66746804601808,
9.90555361358077));
#53966=CARTESIAN_POINT('Ctrl Pts',(0.056448756214413,1.66658089685919,9.90111659037635));
#53967=CARTESIAN_POINT('Ctrl Pts',(0.143555110290162,1.65987871743349,9.89544856154274));
#53968=CARTESIAN_POINT('Ctrl Pts',(0.159283079482503,1.65844333108409,9.8944140932327));
#53969=CARTESIAN_POINT('Ctrl Pts',(0.182134536644928,1.65602978828887,9.89289189779298));
#53970=CARTESIAN_POINT('Ctrl Pts',(0.189276393771199,1.65522871264101,9.89241342329013));
#53971=CARTESIAN_POINT('Ctrl Pts',(0.201803699051694,1.65374143679908,9.89156898514514));
#53972=CARTESIAN_POINT('Ctrl Pts',(0.207191311404195,1.65307508357983,9.89120412626254));
#53973=CARTESIAN_POINT('Ctrl Pts',(0.218948698080024,1.65156251921965,9.89040410712124));
#53974=CARTESIAN_POINT('Ctrl Pts',(0.22531676469835,1.65070580036019,9.88996839850992));
#53975=CARTESIAN_POINT('Ctrl Pts',(0.243146848625318,1.64820196013231,9.88874201690379));
#53976=CARTESIAN_POINT('Ctrl Pts',(0.254596620620649,1.64647217815995,9.88794702302528));
#53977=CARTESIAN_POINT('Ctrl Pts',(0.336624969883425,1.63320363307294,9.88220231437036));
#53978=CARTESIAN_POINT('Ctrl Pts',(0.406406724201536,1.61725129170012,9.87705621534536));
#53979=CARTESIAN_POINT('Ctrl Pts',(0.488368702671291,1.59287423059785,9.87084774580007));
#53980=CARTESIAN_POINT('Ctrl Pts',(0.501747179166583,1.58871081946642,9.86982886028981));
#53981=CARTESIAN_POINT('Ctrl Pts',(0.578125058137468,1.56388086303582,9.86398469475561));
#53982=CARTESIAN_POINT('Ctrl Pts',(0.639901731610865,1.53963582958029,9.85915380254484));
#53983=CARTESIAN_POINT('Ctrl Pts',(0.74482431550036,1.49104831719172,9.85085900013973));
#53984=CARTESIAN_POINT('Ctrl Pts',(0.788638338862812,1.46834555478519,9.84736513427056));
#53985=CARTESIAN_POINT('Ctrl Pts',(0.860405631944635,1.42701776981962,9.84160230737337));
#53986=CARTESIAN_POINT('Ctrl Pts',(0.888918517919397,1.40943311801642,9.83930125306193));
#53987=CARTESIAN_POINT('Ctrl Pts',(0.928318136329917,1.38346268087776,9.83610311658611));
#53988=CARTESIAN_POINT('Ctrl Pts',(0.939659428771498,1.37578476841183,9.83518025184924));
#53989=CARTESIAN_POINT('Ctrl Pts',(0.959058769966445,1.36229985063522,9.83359732503261));
#53990=CARTESIAN_POINT('Ctrl Pts',(0.967161792476038,1.35655913318124,9.83293480097407));
#53991=CARTESIAN_POINT('Ctrl Pts',(0.983621630902639,1.34467544179991,9.83158600103814));
#53992=CARTESIAN_POINT('Ctrl Pts',(0.991973392292757,1.3385261871834,9.83090000556373));
#53993=CARTESIAN_POINT('Ctrl Pts',(1.01301137498834,1.3227312315117,9.82916747226311));
#53994=CARTESIAN_POINT('Ctrl Pts',(1.02561780625701,1.31298061712983,9.82812507063503));
#53995=CARTESIAN_POINT('Ctrl Pts',(1.07486057412706,1.27375107487701,9.82403362848397));
#53996=CARTESIAN_POINT('Ctrl Pts',(1.11038370858937,1.24290614872212,9.82103909834878));
#53997=CARTESIAN_POINT('Ctrl Pts',(1.23402523487795,1.12600949522512,9.81036410464119));
#53998=CARTESIAN_POINT('Ctrl Pts',(1.31383727533622,1.03176869387582,9.80300445802751));
#53999=CARTESIAN_POINT('Ctrl Pts',(1.40539899037475,0.895593910871602,9.79285348558973));
#54000=CARTESIAN_POINT('Ctrl Pts',(1.42699744694836,0.86076280754317,9.79029084338165));
#54001=CARTESIAN_POINT('Ctrl Pts',(1.45557544645789,0.810639276917036,9.78659919426446));
#54002=CARTESIAN_POINT('Ctrl Pts',(1.4636424704079,0.79598152641481,9.78551915654964));
#54003=CARTESIAN_POINT('Ctrl Pts',(1.477484620222,0.769908301111194,9.78359269159236));
#54004=CARTESIAN_POINT('Ctrl Pts',(1.48335167129145,0.758542938744251,9.7827512020552));
#54005=CARTESIAN_POINT('Ctrl Pts',(1.49205050349164,0.741205075418628,9.78146316294614));
#54006=CARTESIAN_POINT('Ctrl Pts',(1.49497871081137,0.735281115813086,9.78102230807849));
#54007=CARTESIAN_POINT('Ctrl Pts',(1.50026312052961,0.724428335657685,9.78021298350743));
#54008=CARTESIAN_POINT('Ctrl Pts',(1.5026304193599,0.719505152479736,9.77984520163599));
#54009=CARTESIAN_POINT('Ctrl Pts',(1.50796428221539,0.708271378946464,9.77900453633642));
#54010=CARTESIAN_POINT('Ctrl Pts',(1.51091545316733,0.701953781708727,9.77853075372782));
#54011=CARTESIAN_POINT('Ctrl Pts',(1.51994010725099,0.682314031831669,9.77705517760469));
#54012=CARTESIAN_POINT('Ctrl Pts',(1.5258775024823,0.668930623127372,9.77604581226147));
#54013=CARTESIAN_POINT('Ctrl Pts',(1.57510776346683,0.553894442801432,9.767347732446));
#54014=CARTESIAN_POINT('Ctrl Pts',(1.60836208156626,0.448253648302818,9.75923338228561));
#54015=CARTESIAN_POINT('Ctrl Pts',(1.64985693769546,0.24927449376688,9.74446825980225));
#54016=CARTESIAN_POINT('Ctrl Pts',(1.66118021813261,0.157005041596671,9.73781377185635));
#54017=CARTESIAN_POINT('Ctrl Pts',(1.66586796274518,0.0355629830142027,
9.72939964313074));
#54018=CARTESIAN_POINT('Ctrl Pts',(1.66623353372136,0.00683983295146041,
9.72743338258102));
#54019=CARTESIAN_POINT('Ctrl Pts',(1.66568670311698,-0.0347936409229971,
9.72461621330597));
#54020=CARTESIAN_POINT('Ctrl Pts',(1.66536693390361,-0.0477051585925001,
9.72374710724748));
#54021=CARTESIAN_POINT('Ctrl Pts',(1.66454028782187,-0.0704115730776858,
9.72222635029701));
#54022=CARTESIAN_POINT('Ctrl Pts',(1.66409700506371,-0.0802080059171749,
9.72157274859218));
#54023=CARTESIAN_POINT('Ctrl Pts',(1.66299127661127,-0.100646348550529,
9.72021414130691));
#54024=CARTESIAN_POINT('Ctrl Pts',(1.66231311388042,-0.111286988923718,
9.7195096572032));
#54025=CARTESIAN_POINT('Ctrl Pts',(1.66026661568557,-0.139176648228174,
9.71767014843599));
#54026=CARTESIAN_POINT('Ctrl Pts',(1.65873161288151,-0.156412427857145,
9.71654035719821));
#54027=CARTESIAN_POINT('Ctrl Pts',(1.65056980147356,-0.234303243945644,
9.71146235049359));
#54028=CARTESIAN_POINT('Ctrl Pts',(1.64088221572044,-0.294593729542408,
9.70761018691498));
#54029=CARTESIAN_POINT('Ctrl Pts',(1.60288466518596,-0.469219931848416,
9.6965091751641));
#54030=CARTESIAN_POINT('Ctrl Pts',(1.5657489940434,-0.581235370587503,9.68947837433791));
#54031=CARTESIAN_POINT('Ctrl Pts',(1.5031989080091,-0.719085969304435,9.68004642642688));
#54032=CARTESIAN_POINT('Ctrl Pts',(1.4883475129231,-0.749341702362119,9.67792243242184));
#54033=CARTESIAN_POINT('Ctrl Pts',(1.46253066189549,-0.798137040348437,
9.67437449457909));
#54034=CARTESIAN_POINT('Ctrl Pts',(1.45210464902936,-0.816952051602266,
9.67297548035268));
#54035=CARTESIAN_POINT('Ctrl Pts',(1.43725012043614,-0.842575738476188,
9.67101970995689));
#54036=CARTESIAN_POINT('Ctrl Pts',(1.43313121993803,-0.849562642484641,
9.67048115002742));
#54037=CARTESIAN_POINT('Ctrl Pts',(1.42607575830524,-0.86133352367105,9.66956438463691));
#54038=CARTESIAN_POINT('Ctrl Pts',(1.4231656650753,-0.866133359340258,9.66918786368616));
#54039=CARTESIAN_POINT('Ctrl Pts',(1.41748758901722,-0.875392759554953,
9.66845612499556));
#54040=CARTESIAN_POINT('Ctrl Pts',(1.41472271411045,-0.879854072417098,
9.66810113523642));
#54041=CARTESIAN_POINT('Ctrl Pts',(1.40708157093585,-0.892054440173599,
9.66712382615363));
#54042=CARTESIAN_POINT('Ctrl Pts',(1.40216266246531,-0.899766375198331,
9.66649882393458));
#54043=CARTESIAN_POINT('Ctrl Pts',(1.3822831231997,-0.930374893007171,9.66399038474938));
#54044=CARTESIAN_POINT('Ctrl Pts',(1.36682401083448,-0.952940706376796,
9.66207844084234));
#54045=CARTESIAN_POINT('Ctrl Pts',(1.33203063542401,-1.00113968310678,9.65787318211656));
#54046=CARTESIAN_POINT('Ctrl Pts',(1.312496332161,-1.02661553015282,9.65557217242202));
#54047=CARTESIAN_POINT('Ctrl Pts',(1.23026319599558,-1.12767488032464,9.64616521533027));
#54048=CARTESIAN_POINT('Ctrl Pts',(1.16166999925484,-1.19821643404209,9.63895449798669));
#54049=CARTESIAN_POINT('Ctrl Pts',(1.03171010310813,-1.31015493586151,9.62665584009421));
#54050=CARTESIAN_POINT('Ctrl Pts',(0.973053079221091,-1.3542902498476,9.62150239099507));
#54051=CARTESIAN_POINT('Ctrl Pts',(0.896904712187983,-1.40407591118448,
9.61529335958614));
#54052=CARTESIAN_POINT('Ctrl Pts',(0.881986000110136,-1.41349494667739,
9.61409805207719));
#54053=CARTESIAN_POINT('Ctrl Pts',(0.85775324022666,-1.42826139397155,9.6121894733294));
#54054=CARTESIAN_POINT('Ctrl Pts',(0.848532548751569,-1.43375861066889,
9.61147076190123));
#54055=CARTESIAN_POINT('Ctrl Pts',(0.830806538715489,-1.44409564762368,
9.61010311701836));
#54056=CARTESIAN_POINT('Ctrl Pts',(0.822310486501808,-1.44895038390453,
9.6094536645505));
#54057=CARTESIAN_POINT('Ctrl Pts',(0.802824801480943,-1.45985812056773,
9.60797761581559));
#54058=CARTESIAN_POINT('Ctrl Pts',(0.791808492673642,-1.46586244897312,
9.60715278155812));
#54059=CARTESIAN_POINT('Ctrl Pts',(0.762232743133817,-1.48155170234157,
9.6049630988651));
#54060=CARTESIAN_POINT('Ctrl Pts',(0.743556462428251,-1.49101242488798,
9.60360608081827));
#54061=CARTESIAN_POINT('Ctrl Pts',(0.614893823103221,-1.55316923111023,
9.59441891342092));
#54062=CARTESIAN_POINT('Ctrl Pts',(0.49958722395514,-1.59400299213205,9.58701604869924));
#54063=CARTESIAN_POINT('Ctrl Pts',(0.317072268125654,-1.63686056433288,
9.57555863192214));
#54064=CARTESIAN_POINT('Ctrl Pts',(0.252475363236973,-1.64806015717417,
9.57154280796395));
#54065=CARTESIAN_POINT('Ctrl Pts',(0.165228744745377,-1.65793636090247,
9.56598418066398));
#54066=CARTESIAN_POINT('Ctrl Pts',(0.143018188975949,-1.65999976314588,
9.56455736076963));
#54067=CARTESIAN_POINT('Ctrl Pts',(0.104895083261007,-1.66277072833362,
9.56207804377577));
#54068=CARTESIAN_POINT('Ctrl Pts',(0.0890011028865264,-1.66369715744989,
9.56103539762414));
#54069=CARTESIAN_POINT('Ctrl Pts',(0.0658941561173299,-1.66471196949202,
9.55950335552001));
#54070=CARTESIAN_POINT('Ctrl Pts',(0.0586894901106203,-1.66498153747689,
9.55902338082443));
#54071=CARTESIAN_POINT('Ctrl Pts',(0.0460057995549087,-1.66537368177267,
9.55817400703662));
#54072=CARTESIAN_POINT('Ctrl Pts',(0.0405275813848081,-1.66551600033975,
9.55780570097485));
#54073=CARTESIAN_POINT('Ctrl Pts',(0.0286191739297413,-1.66576657999992,
9.55700183601556));
#54074=CARTESIAN_POINT('Ctrl Pts',(0.0221891271735024,-1.66586463894967,
9.55656575451637));
#54075=CARTESIAN_POINT('Ctrl Pts',(0.00415546885231957,-1.66603522822074,
9.55533733756193));
#54076=CARTESIAN_POINT('Ctrl Pts',(-0.00744830262296705,-1.66602375540589,
9.55454065930492));
#54077=CARTESIAN_POINT('Ctrl Pts',(-0.0961155783210517,-1.6650097849429,
9.54840997492033));
#54078=CARTESIAN_POINT('Ctrl Pts',(-0.173018129402188,-1.65878202958086,
9.54284823106372));
#54079=CARTESIAN_POINT('Ctrl Pts',(-0.305936075797573,-1.63867365071669,
9.53307672794286));
#54080=CARTESIAN_POINT('Ctrl Pts',(-0.362188474146878,-1.62716563251421,
9.52888968303591));
#54081=CARTESIAN_POINT('Ctrl Pts',(-0.490021991707802,-1.59405468337534,
9.51934805735818));
#54082=CARTESIAN_POINT('Ctrl Pts',(-0.56097530831822,-1.57049073589869,
9.51403492647141));
#54083=CARTESIAN_POINT('Ctrl Pts',(-0.655937280379037,-1.53169197867999,
9.50693938659011));
#54084=CARTESIAN_POINT('Ctrl Pts',(-0.681490725202018,-1.52049484948237,
9.50503092937275));
#54085=CARTESIAN_POINT('Ctrl Pts',(-0.718316354431279,-1.50324338975327,
9.50228034772167));
#54086=CARTESIAN_POINT('Ctrl Pts',(-0.72981797471069,-1.49769316397992,
9.50142121058435));
#54087=CARTESIAN_POINT('Ctrl Pts',(-0.750019230915707,-1.48765685753566,
9.49991177753699));
#54088=CARTESIAN_POINT('Ctrl Pts',(-0.758745156572715,-1.48322539316136,
9.49925962382293));
#54089=CARTESIAN_POINT('Ctrl Pts',(-0.776954801381172,-1.47377486512518,
9.4978981137786));
#54090=CARTESIAN_POINT('Ctrl Pts',(-0.786430128919887,-1.46874054137442,
9.49718933043051));
#54091=CARTESIAN_POINT('Ctrl Pts',(-0.811333121270085,-1.45519927159909,
9.49532516718411));
#54092=CARTESIAN_POINT('Ctrl Pts',(-0.826675890298681,-1.4465384076084,
9.49417528671567));
#54093=CARTESIAN_POINT('Ctrl Pts',(-0.898058342427392,-1.40473686752708,
9.48881439695062));
#54094=CARTESIAN_POINT('Ctrl Pts',(-0.952264945552204,-1.36857129055036,
9.48471394691546));
#54095=CARTESIAN_POINT('Ctrl Pts',(-1.12038435284886,-1.24156746197831,
9.4716581067006));
#54096=CARTESIAN_POINT('Ctrl Pts',(-1.22452743782071,-1.13897885349182,
9.46306590274078));
#54097=CARTESIAN_POINT('Ctrl Pts',(-1.32341529378525,-1.01210786367338,
9.45274176381477));
#54098=CARTESIAN_POINT('Ctrl Pts',(-1.33265938474566,-0.999904643240284,
9.45175089442855));
#54099=CARTESIAN_POINT('Ctrl Pts',(-1.34881228980712,-0.977959101265534,
9.44996934556504));
#54100=CARTESIAN_POINT('Ctrl Pts',(-1.3557870899869,-0.96826646300144,9.44918261784184));
#54101=CARTESIAN_POINT('Ctrl Pts',(-1.36635751749659,-0.95323895653241,
9.44796163927423));
#54102=CARTESIAN_POINT('Ctrl Pts',(-1.37002760883425,-0.947956603136958,
9.44753221952318));
#54103=CARTESIAN_POINT('Ctrl Pts',(-1.37676771134362,-0.938134692382204,
9.44673307075046));
#54104=CARTESIAN_POINT('Ctrl Pts',(-1.37984602430724,-0.933601080798416,
9.44636390477225));
#54105=CARTESIAN_POINT('Ctrl Pts',(-1.38685387262408,-0.923169842751786,
9.4455138779107));
#54106=CARTESIAN_POINT('Ctrl Pts',(-1.39076818773196,-0.917262266734908,
9.44503204539511));
#54107=CARTESIAN_POINT('Ctrl Pts',(-1.40321172423004,-0.898219427833956,
9.44347795171718));
#54108=CARTESIAN_POINT('Ctrl Pts',(-1.41159316629549,-0.88498924977661,
9.44239683318875));
#54109=CARTESIAN_POINT('Ctrl Pts',(-1.46767532093192,-0.793639191331975,
9.43493282635992));
#54110=CARTESIAN_POINT('Ctrl Pts',(-1.50904991793798,-0.711828145844744,
9.42826106152325));
#54111=CARTESIAN_POINT('Ctrl Pts',(-1.57551671441283,-0.548217120506717,
9.41540670471501));
#54112=CARTESIAN_POINT('Ctrl Pts',(-1.60145715012973,-0.467046769708951,
9.40924127323501));
#54113=CARTESIAN_POINT('Ctrl Pts',(-1.6320556844945,-0.337954494045842,
9.39989084826688));
#54114=CARTESIAN_POINT('Ctrl Pts',(-1.64104061152726,-0.291213815799972,
9.39659266222447));
#54115=CARTESIAN_POINT('Ctrl Pts',(-1.65028934074554,-0.228784444790369,
9.39230056887076));
#54116=CARTESIAN_POINT('Ctrl Pts',(-1.65235056278314,-0.213389025977572,
9.39125104775207));
#54117=CARTESIAN_POINT('Ctrl Pts',(-1.65541857727395,-0.187752889084874,
9.38951769821789));
#54118=CARTESIAN_POINT('Ctrl Pts',(-1.65654630510596,-0.17752791492329,
9.38883011315607));
#54119=CARTESIAN_POINT('Ctrl Pts',(-1.65857026742687,-0.157474003506889,
9.38748869313677));
#54120=CARTESIAN_POINT('Ctrl Pts',(-1.65947400696748,-0.147646270185248,
9.38683464948917));
#54121=CARTESIAN_POINT('Ctrl Pts',(-1.66144079941945,-0.123951145187176,
9.3852654417029));
#54122=CARTESIAN_POINT('Ctrl Pts',(-1.66241765143314,-0.11007719080431,
9.38435300365112));
#54123=CARTESIAN_POINT('Ctrl Pts',(-1.66508787822284,-0.0639074084529993,
9.38133625781657));
#54124=CARTESIAN_POINT('Ctrl Pts',(-1.66601474697079,-0.0315734630314515,
9.37925566578851));
#54125=CARTESIAN_POINT('Ctrl Pts',(-1.6659775013047,0.04914121364185,9.37412372009076));
#54126=CARTESIAN_POINT('Ctrl Pts',(-1.66384846670606,0.0974920269668017,
9.37110538969817));
#54127=CARTESIAN_POINT('Ctrl Pts',(-1.6506564845205,0.24777324822732,9.36179169531954));
#54128=CARTESIAN_POINT('Ctrl Pts',(-1.63229499545893,0.34881223821726,9.35563829044878));
#54129=CARTESIAN_POINT('Ctrl Pts',(-1.59271662237536,0.490736904679573,
9.34647552258277));
#54130=CARTESIAN_POINT('Ctrl Pts',(-1.57892576694212,0.533442703970636,
9.34364514980345));
#54131=CARTESIAN_POINT('Ctrl Pts',(-1.56343130066142,0.575533290185854,
9.34073387093129));
#54132=CARTESIAN_POINT('Ctrl Pts',(-1.56343129957118,0.575533293147481,
9.53174555314795));
#54133=CARTESIAN_POINT('Ctrl Pts',(-1.58419289085892,0.519134606860111,
9.53542162378452));
#54134=CARTESIAN_POINT('Ctrl Pts',(-1.60188765055432,0.461653412997373,
9.53911575611647));
#54135=CARTESIAN_POINT('Ctrl Pts',(-1.62185532032787,0.381630777066599,
9.54433646674948));
#54136=CARTESIAN_POINT('Ctrl Pts',(-1.62683459671384,0.359813598003652,
9.54576773531309));
#54137=CARTESIAN_POINT('Ctrl Pts',(-1.63460968963582,0.322276075362092,
9.54825405230925));
#54138=CARTESIAN_POINT('Ctrl Pts',(-1.63762178126171,0.306603264746934,
9.54929917577935));
#54139=CARTESIAN_POINT('Ctrl Pts',(-1.64166824217043,0.283784191892934,
9.55083421448561));
#54140=CARTESIAN_POINT('Ctrl Pts',(-1.64288214023067,0.276670116609555,
9.55131465725133));
#54141=CARTESIAN_POINT('Ctrl Pts',(-1.64492863877413,0.264187966370889,
9.55216127572685));
#54142=CARTESIAN_POINT('Ctrl Pts',(-1.64578126493858,0.25882336639988,9.55252632691499));
#54143=CARTESIAN_POINT('Ctrl Pts',(-1.64758221701498,0.247123196194553,
9.55332518876194));
#54144=CARTESIAN_POINT('Ctrl Pts',(-1.64852022836828,0.240786397304346,
9.55375953339173));
#54145=CARTESIAN_POINT('Ctrl Pts',(-1.65103869681518,0.223067846765733,
9.55497841988917));
#54146=CARTESIAN_POINT('Ctrl Pts',(-1.65253794025133,0.211675176587708,
9.55576720208956));
#54147=CARTESIAN_POINT('Ctrl Pts',(-1.66191605512822,0.134225859657009,
9.56115974042736));
#54148=CARTESIAN_POINT('Ctrl Pts',(-1.6659491898134,0.0677707496558123,
9.56593378901129));
#54149=CARTESIAN_POINT('Ctrl Pts',(-1.66611356037785,-0.149427585103849,
9.58168203907383));
#54150=CARTESIAN_POINT('Ctrl Pts',(-1.6457815380196,-0.29947360437319,9.59270913271564));
#54151=CARTESIAN_POINT('Ctrl Pts',(-1.60002946606151,-0.464636920357443,
9.60449250556361));
#54152=CARTESIAN_POINT('Ctrl Pts',(-1.59415191821658,-0.48441871125564,
9.60589954043457));
#54153=CARTESIAN_POINT('Ctrl Pts',(-1.58413773354867,-0.515964070477924,
9.60813723806045));
#54154=CARTESIAN_POINT('Ctrl Pts',(-1.58023409313649,-0.527798736651318,
9.60897536426683));
#54155=CARTESIAN_POINT('Ctrl Pts',(-1.57303228967165,-0.548835993771317,
9.6104630867351));
#54156=CARTESIAN_POINT('Ctrl Pts',(-1.56978526461057,-0.558055339923406,
9.61111432958306));
#54157=CARTESIAN_POINT('Ctrl Pts',(-1.56278710066076,-0.577380869580575,
9.61247815168184));
#54158=CARTESIAN_POINT('Ctrl Pts',(-1.55901862204584,-0.587480328073059,
9.61319012095391));
#54159=CARTESIAN_POINT('Ctrl Pts',(-1.54875083651637,-0.614203054840307,
9.61507242382464));
#54160=CARTESIAN_POINT('Ctrl Pts',(-1.54208185885704,-0.630759959740643,
9.61623705948122));
#54161=CARTESIAN_POINT('Ctrl Pts',(-1.50523746668701,-0.718153309609106,
9.62238126117852));
#54162=CARTESIAN_POINT('Ctrl Pts',(-1.47044301419912,-0.78694570376569,
9.62720069765186));
#54163=CARTESIAN_POINT('Ctrl Pts',(-1.37983173973436,-0.938940741423909,
9.63810383654603));
#54164=CARTESIAN_POINT('Ctrl Pts',(-1.32103430896475,-1.02000593080992,
9.6441101105277));
#54165=CARTESIAN_POINT('Ctrl Pts',(-1.22242884563063,-1.13301723109962,
9.65345061340903));
#54166=CARTESIAN_POINT('Ctrl Pts',(-1.18784898071334,-1.16921943639785,
9.65661942741841));
#54167=CARTESIAN_POINT('Ctrl Pts',(-1.14380791337771,-1.21135405531006,
9.66061248257686));
#54168=CARTESIAN_POINT('Ctrl Pts',(-1.13584554207816,-1.21882323533717,
9.66133281881186));
#54169=CARTESIAN_POINT('Ctrl Pts',(-1.12319063377697,-1.23046259600355,
9.66247631809722));
#54170=CARTESIAN_POINT('Ctrl Pts',(-1.11854678303275,-1.23468558382038,
9.66289565438378));
#54171=CARTESIAN_POINT('Ctrl Pts',(-1.10978235844957,-1.24256568038021,
9.66368679984777));
#54172=CARTESIAN_POINT('Ctrl Pts',(-1.10566737330146,-1.24622871465662,
9.66405816120041));
#54173=CARTESIAN_POINT('Ctrl Pts',(-1.09593511349671,-1.25480593320086,
9.66493616700633));
#54174=CARTESIAN_POINT('Ctrl Pts',(-1.09030290399817,-1.25970285194015,
9.66544403797978));
#54175=CARTESIAN_POINT('Ctrl Pts',(-1.07145436670136,-1.27586959409184,
9.66714229833874));
#54176=CARTESIAN_POINT('Ctrl Pts',(-1.05809521873624,-1.28697013560504,
9.66834375313866));
#54177=CARTESIAN_POINT('Ctrl Pts',(-1.02503542702626,-1.3135778922235,9.67130669037306));
#54178=CARTESIAN_POINT('Ctrl Pts',(-1.00515391109514,-1.32885288324915,
9.67307984866249));
#54179=CARTESIAN_POINT('Ctrl Pts',(-0.919496277229146,-1.39164148562462,
9.68065890495535));
#54180=CARTESIAN_POINT('Ctrl Pts',(-0.850641653369231,-1.43476388016848,
9.6865982002319));
#54181=CARTESIAN_POINT('Ctrl Pts',(-0.690278589420767,-1.51958128412775,
9.69977672845188));
#54182=CARTESIAN_POINT('Ctrl Pts',(-0.597570605812225,-1.55837326176305,
9.70695788300536));
#54183=CARTESIAN_POINT('Ctrl Pts',(-0.479379413053165,-1.59571623279424,
9.71549117644586));
#54184=CARTESIAN_POINT('Ctrl Pts',(-0.45668642165241,-1.60235842712725,
9.71710350824116));
#54185=CARTESIAN_POINT('Ctrl Pts',(-0.422144563164161,-1.61167526870591,
9.71951966447463));
#54186=CARTESIAN_POINT('Ctrl Pts',(-0.410396007002416,-1.61470688823499,
9.72033489186031));
#54187=CARTESIAN_POINT('Ctrl Pts',(-0.389179464835656,-1.61993511654294,
9.72179562592394));
#54188=CARTESIAN_POINT('Ctrl Pts',(-0.379723492865078,-1.62217770712472,
9.72244258409009));
#54189=CARTESIAN_POINT('Ctrl Pts',(-0.359426392473754,-1.62680418797331,
9.72382280665389));
#54190=CARTESIAN_POINT('Ctrl Pts',(-0.348579925351779,-1.62916274303221,
9.72455523304445));
#54191=CARTESIAN_POINT('Ctrl Pts',(-0.318765045895209,-1.63533456980239,
9.72655501467582));
#54192=CARTESIAN_POINT('Ctrl Pts',(-0.299752135064599,-1.63892617826557,
9.72781531336956));
#54193=CARTESIAN_POINT('Ctrl Pts',(-0.161307539077506,-1.66258895126955,
9.7368937428627));
#54194=CARTESIAN_POINT('Ctrl Pts',(-0.0400629299417626,-1.66991668446338,
9.74427886431592));
#54195=CARTESIAN_POINT('Ctrl Pts',(0.176728174425355,-1.65937476916281,
9.75753389347799));
#54196=CARTESIAN_POINT('Ctrl Pts',(0.271945605355837,-1.64645018288157,
9.76338695716254));
#54197=CARTESIAN_POINT('Ctrl Pts',(0.380652660388352,-1.62200508794904,
9.7706194104116));
#54198=CARTESIAN_POINT('Ctrl Pts',(0.395748144568305,-1.61838818487052,
9.77163653388678));
#54199=CARTESIAN_POINT('Ctrl Pts',(0.417634142804322,-1.61281976493946,
9.77313282492087));
#54200=CARTESIAN_POINT('Ctrl Pts',(0.424466773500164,-1.61103501672081,
9.77360304298463));
#54201=CARTESIAN_POINT('Ctrl Pts',(0.436578935510371,-1.60778880495735,
9.77444242779257));
#54202=CARTESIAN_POINT('Ctrl Pts',(0.441862903541104,-1.60634466457602,
9.77481060509767));
#54203=CARTESIAN_POINT('Ctrl Pts',(0.453353598785978,-1.60314320110716,
9.77561569180437));
#54204=CARTESIAN_POINT('Ctrl Pts',(0.459557179861626,-1.60137590955471,
9.7760531377531));
#54205=CARTESIAN_POINT('Ctrl Pts',(0.477297898498818,-1.5962103153045,9.77731184140587));
#54206=CARTESIAN_POINT('Ctrl Pts',(0.488808427020847,-1.59272312577864,
9.77813789254889));
#54207=CARTESIAN_POINT('Ctrl Pts',(0.593983063841548,-1.55961233732092,
9.7857657102244));
#54208=CARTESIAN_POINT('Ctrl Pts',(0.684883904509433,-1.52188587723097,
9.79293049503105));
#54209=CARTESIAN_POINT('Ctrl Pts',(0.875841767945102,-1.42204385587322,
9.80861482788145));
#54210=CARTESIAN_POINT('Ctrl Pts',(0.973752164077067,-1.35688007668907,
9.81707010185451));
#54211=CARTESIAN_POINT('Ctrl Pts',(1.08030742321903,-1.26843999805208,9.82659818715554));
#54212=CARTESIAN_POINT('Ctrl Pts',(1.09633862057704,-1.25460984283107,9.82804257648998));
#54213=CARTESIAN_POINT('Ctrl Pts',(1.12149376283654,-1.23205796169355,9.83032756153957));
#54214=CARTESIAN_POINT('Ctrl Pts',(1.13078930922861,-1.22353203242732,9.83117613150749));
#54215=CARTESIAN_POINT('Ctrl Pts',(1.14712991819355,-1.20819902558158,9.83267571876962));
#54216=CARTESIAN_POINT('Ctrl Pts',(1.15421335904524,-1.20143391972935,9.83332847758013));
#54217=CARTESIAN_POINT('Ctrl Pts',(1.16891088844057,-1.18714694635202,9.83468885029143));
#54218=CARTESIAN_POINT('Ctrl Pts',(1.17651300667199,-1.17961336525955,9.8353959120697));
#54219=CARTESIAN_POINT('Ctrl Pts',(1.19634556427573,-1.15957714856435,9.83725009029404));
#54220=CARTESIAN_POINT('Ctrl Pts',(1.20845284692679,-1.14695406496431,9.83839181613675));
#54221=CARTESIAN_POINT('Ctrl Pts',(1.26855777960162,-1.08227996958015,9.84411482428737));
#54222=CARTESIAN_POINT('Ctrl Pts',(1.31340442751963,-1.02739446222141,9.84856256765901));
#54223=CARTESIAN_POINT('Ctrl Pts',(1.39478704717676,-0.913720233845686,
9.85720253928365));
#54224=CARTESIAN_POINT('Ctrl Pts',(1.43142444823527,-0.855184097794034,
9.8613904458194));
#54225=CARTESIAN_POINT('Ctrl Pts',(1.47477745111027,-0.775285479383363,
9.86695373920112));
#54226=CARTESIAN_POINT('Ctrl Pts',(1.48484621669684,-0.755822590656976,
9.86829792002095));
#54227=CARTESIAN_POINT('Ctrl Pts',(1.52323941239803,-0.677878728364892,
9.87365786097997));
#54228=CARTESIAN_POINT('Ctrl Pts',(1.54851289668559,-0.617967355228113,
9.8777259195766));
#54229=CARTESIAN_POINT('Ctrl Pts',(1.57404819299209,-0.545948193219906,
9.882725677946));
#54230=CARTESIAN_POINT('Ctrl Pts',(1.57776361754512,-0.535115962071062,
9.88348054244917));
#54231=CARTESIAN_POINT('Ctrl Pts',(1.58337997721785,-0.518174460621776,
9.88466685992084));
#54232=CARTESIAN_POINT('Ctrl Pts',(1.58535796896452,-0.512090842250893,
9.88509400215145));
#54233=CARTESIAN_POINT('Ctrl Pts',(1.58895111626634,-0.500819202829908,
9.88588777399612));
#54234=CARTESIAN_POINT('Ctrl Pts',(1.59057598861679,-0.495634487372464,
9.88625383716857));
#54235=CARTESIAN_POINT('Ctrl Pts',(1.59430393741137,-0.483532038852569,
9.88711046885706));
#54236=CARTESIAN_POINT('Ctrl Pts',(1.59638736377652,-0.476608494826912,
9.88760213628928));
#54237=CARTESIAN_POINT('Ctrl Pts',(1.60294575600934,-0.454288434898384,
9.88919184426562));
#54238=CARTESIAN_POINT('Ctrl Pts',(1.60724338808575,-0.438841341498262,
9.89029916431186));
#54239=CARTESIAN_POINT('Ctrl Pts',(1.61703854665122,-0.401558588527275,
9.89298496994333));
#54240=CARTESIAN_POINT('Ctrl Pts',(1.62231753936912,-0.379669145462246,
9.89457263350263));
#54241=CARTESIAN_POINT('Ctrl Pts',(1.6414489827899,-0.292636895273826,9.90091097752498));
#54242=CARTESIAN_POINT('Ctrl Pts',(1.65183322335965,-0.226797726728758,
9.90576010235927));
#54243=CARTESIAN_POINT('Ctrl Pts',(1.6698397421027,-0.040779018369514,9.91936424862656));
#54244=CARTESIAN_POINT('Ctrl Pts',(1.668429260666,0.079884076545479,9.92804832284216));
#54245=CARTESIAN_POINT('Ctrl Pts',(1.65151268583907,0.22023631857544,9.93777345061942));
#54246=CARTESIAN_POINT('Ctrl Pts',(1.64860123931839,0.241064744818895,9.93920797397614));
#54247=CARTESIAN_POINT('Ctrl Pts',(1.64332013023371,0.274249934266454,9.94148048195015));
#54248=CARTESIAN_POINT('Ctrl Pts',(1.64120360382886,0.286644069708899,9.94232630446582));
#54249=CARTESIAN_POINT('Ctrl Pts',(1.63718998237085,0.308643463200404,9.94382276076907));
#54250=CARTESIAN_POINT('Ctrl Pts',(1.63534816936109,0.318258067847762,9.94447511106323));
#54251=CARTESIAN_POINT('Ctrl Pts',(1.63131170833158,0.338368243603977,9.94583634188096));
#54252=CARTESIAN_POINT('Ctrl Pts',(1.62910025988252,0.348860015389673,9.94654465537609));
#54253=CARTESIAN_POINT('Ctrl Pts',(1.6229957505092,0.376496846832748,9.94840600944377));
#54254=CARTESIAN_POINT('Ctrl Pts',(1.61893225685895,0.393603185801709,9.94955358163528));
#54255=CARTESIAN_POINT('Ctrl Pts',(1.59678063806785,0.480700768755718,9.95537810683076));
#54256=CARTESIAN_POINT('Ctrl Pts',(1.57442066810132,0.549529876782667,9.95991537558045));
#54257=CARTESIAN_POINT('Ctrl Pts',(1.51040557830855,0.710181914892721,9.97059487075951));
#54258=CARTESIAN_POINT('Ctrl Pts',(1.46476198713227,0.800096519125323,9.97664129069514));
#54259=CARTESIAN_POINT('Ctrl Pts',(1.38250698943556,0.931216017803965,9.98625169062259));
#54260=CARTESIAN_POINT('Ctrl Pts',(1.3515109451724,0.975656568627253,9.98966969220912));
#54261=CARTESIAN_POINT('Ctrl Pts',(1.31159441334511,1.02732681714753,9.99394489749943));
#54262=CARTESIAN_POINT('Ctrl Pts',(1.30469050269491,1.03608058084558,9.99468018475039));
#54263=CARTESIAN_POINT('Ctrl Pts',(1.29373039560431,1.04969410884822,9.99584223304506));
#54264=CARTESIAN_POINT('Ctrl Pts',(1.28973332146283,1.05460135352278,9.99626496080528));
#54265=CARTESIAN_POINT('Ctrl Pts',(1.2825631425793,1.06330251914205,9.99702163908297));
#54266=CARTESIAN_POINT('Ctrl Pts',(1.27940096817029,1.06710525355877,9.99735480784343));
#54267=CARTESIAN_POINT('Ctrl Pts',(1.27169456170755,1.07628924989468,9.9981654185625));
#54268=CARTESIAN_POINT('Ctrl Pts',(1.26713312439175,1.08165579010145,9.99864408580436));
#54269=CARTESIAN_POINT('Ctrl Pts',(1.2527426071593,1.09837031483181,10.0001502305882));
#54270=CARTESIAN_POINT('Ctrl Pts',(1.24279439408224,1.10961409648543,10.0011857201749));
#54271=CARTESIAN_POINT('Ctrl Pts',(1.18961316946802,1.16810881660869,10.0066846736551));
#54272=CARTESIAN_POINT('Ctrl Pts',(1.14383771951679,1.21296798751377,10.0112913918291));
#54273=CARTESIAN_POINT('Ctrl Pts',(1.01285855911909,1.32730419149547,10.0239079553979));
#54274=CARTESIAN_POINT('Ctrl Pts',(0.923167634812829,1.39118122265691,10.031947513982));
#54275=CARTESIAN_POINT('Ctrl Pts',(0.78461644643187,1.4705146830061,10.0432271204965));
#54276=CARTESIAN_POINT('Ctrl Pts',(0.740305098230693,1.49331364696042,10.0466871884885));
#54277=CARTESIAN_POINT('Ctrl Pts',(0.680274488975569,1.52087027175961,10.051184893164));
#54278=CARTESIAN_POINT('Ctrl Pts',(0.66541579010376,1.5274297439159,10.05228337898));
#54279=CARTESIAN_POINT('Ctrl Pts',(0.640855737489063,1.53784551422447,10.05407553266));
#54280=CARTESIAN_POINT('Ctrl Pts',(0.631210141182511,1.5418296495147,10.0547734980039));
#54281=CARTESIAN_POINT('Ctrl Pts',(0.612345332118319,1.54941509583786,10.0561274201735));
#54282=CARTESIAN_POINT('Ctrl Pts',(0.603130229953526,1.55302539512075,10.0567836564511));
#54283=CARTESIAN_POINT('Ctrl Pts',(0.581273040672289,1.56136473004009,10.0583284057609));
#54284=CARTESIAN_POINT('Ctrl Pts',(0.56860445181398,1.56602272114599,10.0592145226758));
#54285=CARTESIAN_POINT('Ctrl Pts',(0.525504637368104,1.58127769562196,10.0621994089584));
#54286=CARTESIAN_POINT('Ctrl Pts',(0.494821960615776,1.59114603997098,10.0642743072812));
#54287=CARTESIAN_POINT('Ctrl Pts',(0.419009090516657,1.61312401207268,10.0692972662629));
#54288=CARTESIAN_POINT('Ctrl Pts',(0.373618344532987,1.6242375162892,10.0722159149512));
#54289=CARTESIAN_POINT('Ctrl Pts',(0.26025489865599,1.64698876606478,10.0793634043344));
#54290=CARTESIAN_POINT('Ctrl Pts',(0.191914593555625,1.65634345175939,10.0835470828311));
#54291=CARTESIAN_POINT('Ctrl Pts',(0.0998712587242807,1.6631682269327,10.089194858098));
#54292=CARTESIAN_POINT('Ctrl Pts',(0.0765176552312613,1.66440615004458,
10.0906292818935));
#54293=CARTESIAN_POINT('Ctrl Pts',(-0.0109887161014974,1.66719906392807,
10.0960325048454));
#54294=CARTESIAN_POINT('Ctrl Pts',(-0.0751808909474305,1.66553875170138,
10.1000523508879));
#54295=CARTESIAN_POINT('Ctrl Pts',(-0.150499097483795,1.65922773188982,
10.1049980510783));
#54296=CARTESIAN_POINT('Ctrl Pts',(-0.161878660853386,1.6581561826447,10.1057515074042));
#54297=CARTESIAN_POINT('Ctrl Pts',(-0.179603557902194,1.65630293834261,
10.1069360800195));
#54298=CARTESIAN_POINT('Ctrl Pts',(-0.185957196213266,1.6556016366683,10.1073629057951));
#54299=CARTESIAN_POINT('Ctrl Pts',(-0.19720946095798,1.65429404643678,10.1081229750402));
#54300=CARTESIAN_POINT('Ctrl Pts',(-0.20210965055095,1.65370252780854,10.1084553917751));
#54301=CARTESIAN_POINT('Ctrl Pts',(-0.213905823672248,1.65222535902512,
10.109259004576));
#54302=CARTESIAN_POINT('Ctrl Pts',(-0.220798896967757,1.65131831611712,
10.1097313678525));
#54303=CARTESIAN_POINT('Ctrl Pts',(-0.242082486150913,1.64838201744531,
10.1111980349608));
#54304=CARTESIAN_POINT('Ctrl Pts',(-0.256451832644973,1.64620765011811,
10.1121997841692));
#54305=CARTESIAN_POINT('Ctrl Pts',(-0.329716481184864,1.63413878354507,
10.1173603502247));
#54306=CARTESIAN_POINT('Ctrl Pts',(-0.388072555233054,1.62127135312826,
10.1216448258449));
#54307=CARTESIAN_POINT('Ctrl Pts',(-0.547978501957975,1.57688404350042,
10.1336697971635));
#54308=CARTESIAN_POINT('Ctrl Pts',(-0.647409003187102,1.53873615273816,
10.1414590855755));
#54309=CARTESIAN_POINT('Ctrl Pts',(-0.793482994309661,1.46600827584074,
10.15304878776));
#54310=CARTESIAN_POINT('Ctrl Pts',(-0.843105101802522,1.43804402387369,
10.1570190139605));
#54311=CARTESIAN_POINT('Ctrl Pts',(-0.905563333304984,1.3984991670277,10.1620589542337));
#54312=CARTESIAN_POINT('Ctrl Pts',(-0.919783767187433,1.38918779493509,
10.1632096327131));
#54313=CARTESIAN_POINT('Ctrl Pts',(-0.942634971547567,1.37372034890518,
10.1650645529685));
#54314=CARTESIAN_POINT('Ctrl Pts',(-0.951353553816348,1.36769686377908,
10.1657736958843));
#54315=CARTESIAN_POINT('Ctrl Pts',(-0.967488583018499,1.35632056660546,
10.1670889837075));
#54316=CARTESIAN_POINT('Ctrl Pts',(-0.974919520667993,1.3509891086082,10.1676959085347));
#54317=CARTESIAN_POINT('Ctrl Pts',(-0.98273468800006,1.34528391587296,10.1683355724489));
#54318=CARTESIAN_POINT('Ctrl Pts',(-0.983162918554376,1.34497098737698,
10.1683706270508));
#54319=CARTESIAN_POINT('Ctrl Pts',(-0.983986378641286,1.34436864238054,
10.1684380432185));
#54320=CARTESIAN_POINT('Ctrl Pts',(-0.9843816300402,1.34407925599942,10.1684704059325));
#54321=CARTESIAN_POINT('Ctrl Pts',(-0.985149338739101,1.34351665183348,
10.168533272283));
#54322=CARTESIAN_POINT('Ctrl Pts',(-0.985521810118118,1.34324345341943,
10.1685637766573));
#54323=CARTESIAN_POINT('Ctrl Pts',(-0.986251615317336,1.34270769265317,
10.1686235522407));
#54324=CARTESIAN_POINT('Ctrl Pts',(-0.986608958005362,1.34244514249569,
10.1686528239135));
#54325=CARTESIAN_POINT('Ctrl Pts',(-0.987314584874487,1.34192626380884,
10.1687106313533));
#54326=CARTESIAN_POINT('Ctrl Pts',(-0.987662874143681,1.34166994229008,
10.1687391673855));
#54327=CARTESIAN_POINT('Ctrl Pts',(-0.988355495524049,1.34115979564662,
10.1687959211219));
#54328=CARTESIAN_POINT('Ctrl Pts',(-0.988699829745768,1.34090597345702,
10.1688241389353));
#54329=CARTESIAN_POINT('Ctrl Pts',(-0.989389061443817,1.34039750406156,
10.1688806265481));
#54330=CARTESIAN_POINT('Ctrl Pts',(-0.989733958462559,1.34014285629023,
10.1689088963228));
#54331=CARTESIAN_POINT('Ctrl Pts',(-0.990428537942846,1.33962961313098,
10.1689658340318));
#54332=CARTESIAN_POINT('Ctrl Pts',(-0.990778217524352,1.33937101388261,
10.1689945018154));
#54333=CARTESIAN_POINT('Ctrl Pts',(-0.99940569619487,1.3329854896335,10.1697018834107));
#54334=CARTESIAN_POINT('Ctrl Pts',(-1.00762675740504,1.3267819665612,10.1703776433778));
#54335=CARTESIAN_POINT('Ctrl Pts',(-1.02728463730618,1.31166024102058,10.1719980522675));
#54336=CARTESIAN_POINT('Ctrl Pts',(-1.03866368408487,1.30266806451372,10.1729398084153));
#54337=CARTESIAN_POINT('Ctrl Pts',(-1.06935368047912,1.27775777032562,10.1754917784745));
#54338=CARTESIAN_POINT('Ctrl Pts',(-1.08842611848111,1.26155098800991,10.1770909060809));
#54339=CARTESIAN_POINT('Ctrl Pts',(-1.14953064317724,1.20720977262236,10.1822702198343));
#54340=CARTESIAN_POINT('Ctrl Pts',(-1.18998215605509,1.16735570037742,10.1857874385844));
#54341=CARTESIAN_POINT('Ctrl Pts',(-1.27182548869574,1.07803635798541,10.1932270069303));
#54342=CARTESIAN_POINT('Ctrl Pts',(-1.31253845308454,1.02807839318132,10.1971334290981));
#54343=CARTESIAN_POINT('Ctrl Pts',(-1.39439776626126,0.914816476774274,
10.2057147958404));
#54344=CARTESIAN_POINT('Ctrl Pts',(-1.43433810898828,0.850826391364902,
10.2103975638657));
#54345=CARTESIAN_POINT('Ctrl Pts',(-1.47526709663119,0.774130174487371,
10.2160838642322));
#54346=CARTESIAN_POINT('Ctrl Pts',(-1.48062070941544,0.763840840631683,
10.2168482248152));
#54347=CARTESIAN_POINT('Ctrl Pts',(-1.48877440603304,0.747762069374777,
10.2180463052736));
#54348=CARTESIAN_POINT('Ctrl Pts',(-1.49164925891114,0.742010666619104,
10.218475576946));
#54349=CARTESIAN_POINT('Ctrl Pts',(-1.49688972861089,0.731373099462795,
10.2192711245895));
#54350=CARTESIAN_POINT('Ctrl Pts',(-1.49926484533613,0.726491838009372,
10.2196368103054));
#54351=CARTESIAN_POINT('Ctrl Pts',(-1.50472643158455,0.715126516610433,
10.2204896788759));
#54352=CARTESIAN_POINT('Ctrl Pts',(-1.50779486180267,0.708634051262194,
10.2209779280245));
#54353=CARTESIAN_POINT('Ctrl Pts',(-1.51746354186941,0.687829056989506,
10.222545372486));
#54354=CARTESIAN_POINT('Ctrl Pts',(-1.52390247370742,0.673443106853239,
10.2236335005455));
#54355=CARTESIAN_POINT('Ctrl Pts',(-1.54198585812882,0.631453190263509,
10.2268174900613));
#54356=CARTESIAN_POINT('Ctrl Pts',(-1.55308786246816,0.603631150045019,
10.2289369329063));
#54357=CARTESIAN_POINT('Ctrl Pts',(-1.56343128570986,0.575533330801617,
10.2310772794004));
#54358=CARTESIAN_POINT('Origin',(0.,0.,11.));
#54359=CARTESIAN_POINT('',(-1.5634312473966,0.575533434879242,10.9335682035678));
#54360=CARTESIAN_POINT('',(-1.56343131785294,0.575533243485219,10.7380842620731));
#54361=CARTESIAN_POINT('',(-1.56343130033213,0.575533291080363,11.));
#54362=CARTESIAN_POINT('',(-1.66599935349477,-0.0014677039958931,10.0778956387897));
#54363=CARTESIAN_POINT('Ctrl Pts',(-1.56343131785294,0.575533243485219,
10.7380842620731));
#54364=CARTESIAN_POINT('Ctrl Pts',(-1.54669125760662,0.621007479331894,
10.7346561303571));
#54365=CARTESIAN_POINT('Ctrl Pts',(-1.52797002107001,0.665743709967646,
10.7312816482152));
#54366=CARTESIAN_POINT('Ctrl Pts',(-1.49964821480684,0.725903166842574,
10.7267411743421));
#54367=CARTESIAN_POINT('Ctrl Pts',(-1.49171542647364,0.742068262625956,
10.7255207355039));
#54368=CARTESIAN_POINT('Ctrl Pts',(-1.47860171470767,0.767730342795993,
10.7235819413168));
#54369=CARTESIAN_POINT('Ctrl Pts',(-1.47358784994133,0.777310599456636,
10.722857833018));
#54370=CARTESIAN_POINT('Ctrl Pts',(-1.46386878823258,0.795449266508267,
10.7214859929087));
#54371=CARTESIAN_POINT('Ctrl Pts',(-1.45918093310503,0.804016402907594,
10.7208376842958));
#54372=CARTESIAN_POINT('Ctrl Pts',(-1.44827002431254,0.823546497044163,
10.7193586301703));
#54373=CARTESIAN_POINT('Ctrl Pts',(-1.44199728264548,0.834481124707548,
10.7185297001952));
#54374=CARTESIAN_POINT('Ctrl Pts',(-1.42191432600201,0.868586907288862,
10.7159406018878));
#54375=CARTESIAN_POINT('Ctrl Pts',(-1.40766472694261,0.891495212758521,
10.7141963174113));
#54376=CARTESIAN_POINT('Ctrl Pts',(-1.34317483435546,0.989767548629385,
10.7066731886934));
#54377=CARTESIAN_POINT('Ctrl Pts',(-1.28739151468958,1.06131240460098,10.7011000723651));
#54378=CARTESIAN_POINT('Ctrl Pts',(-1.15153669320075,1.20898122959927,10.6888358693497));
#54379=CARTESIAN_POINT('Ctrl Pts',(-1.06917509285037,1.28239258027238,10.682193434787));
#54380=CARTESIAN_POINT('Ctrl Pts',(-0.965807212193965,1.35760409028809,
10.6739346038279));
#54381=CARTESIAN_POINT('Ctrl Pts',(-0.951257169435558,1.36783850397806,
10.6727733757274));
#54382=CARTESIAN_POINT('Ctrl Pts',(-0.930750785230871,1.38177714926392,
10.6711342925756));
#54383=CARTESIAN_POINT('Ctrl Pts',(-0.924930122562201,1.38568011405303,
10.6706687709231));
#54384=CARTESIAN_POINT('Ctrl Pts',(-0.914410206921661,1.39263828388022,
10.6698265874857));
#54385=CARTESIAN_POINT('Ctrl Pts',(-0.909719759761508,1.39570676489599,
10.6694507946015));
#54386=CARTESIAN_POINT('Ctrl Pts',(-0.900064069009622,1.40195414694521,
10.6686764014897));
#54387=CARTESIAN_POINT('Ctrl Pts',(-0.895097307360368,1.40513044450681,
10.6682776514722));
#54388=CARTESIAN_POINT('Ctrl Pts',(-0.882114152632687,1.41333654294391,
10.6672344602678));
#54389=CARTESIAN_POINT('Ctrl Pts',(-0.874071710082956,1.41832443291388,
10.6665874103323));
#54390=CARTESIAN_POINT('Ctrl Pts',(-0.837715798585621,1.44044557072019,
10.6636601581778));
#54391=CARTESIAN_POINT('Ctrl Pts',(-0.80894004755658,1.45680020939396,10.6613372308029));
#54392=CARTESIAN_POINT('Ctrl Pts',(-0.721885077965701,1.50290311988185,
10.6543325201173));
#54393=CARTESIAN_POINT('Ctrl Pts',(-0.66232106785631,1.53008684651151,10.6495714266148));
#54394=CARTESIAN_POINT('Ctrl Pts',(-0.487473540033794,1.5977569027983,10.635923552115));
#54395=CARTESIAN_POINT('Ctrl Pts',(-0.369111921603434,1.6291790415787,10.6271055177121));
#54396=CARTESIAN_POINT('Ctrl Pts',(-0.22767123015447,1.65050284664622,10.6172668745934));
#54397=CARTESIAN_POINT('Ctrl Pts',(-0.206922819459439,1.65323224368624,
10.6158395840411));
#54398=CARTESIAN_POINT('Ctrl Pts',(-0.173662958595634,1.65697148712657,
10.6135762519264));
#54399=CARTESIAN_POINT('Ctrl Pts',(-0.161182550992097,1.6582320502666,10.6127324715235));
#54400=CARTESIAN_POINT('Ctrl Pts',(-0.138943276844838,1.66022483523352,
10.6112383666309));
#54401=CARTESIAN_POINT('Ctrl Pts',(-0.129190080884934,1.661012241896,10.6105863439705));
#54402=CARTESIAN_POINT('Ctrl Pts',(-0.108722158101178,1.66248330807813,
10.6092245416772));
#54403=CARTESIAN_POINT('Ctrl Pts',(-0.0980065896434857,1.66314941445107,
10.6085153399706));
#54404=CARTESIAN_POINT('Ctrl Pts',(-0.0696619185256244,1.66463649156229,
10.6066487790653));
#54405=CARTESIAN_POINT('Ctrl Pts',(-0.0520246211011804,1.66528103018159,
10.6054969454387));
#54406=CARTESIAN_POINT('Ctrl Pts',(0.0390245101569303,1.66716033507488,
10.5995953880143));
#54407=CARTESIAN_POINT('Ctrl Pts',(0.112453783752614,1.66382168613298,10.5949901253429));
#54408=CARTESIAN_POINT('Ctrl Pts',(0.280956841043332,1.64494952259849,10.5845252302558));
#54409=CARTESIAN_POINT('Ctrl Pts',(0.375374010994471,1.62600402554265,10.5787414599683));
#54410=CARTESIAN_POINT('Ctrl Pts',(0.522473207396021,1.58298546039346,10.5692448169471));
#54411=CARTESIAN_POINT('Ctrl Pts',(0.576450684788773,1.56413693994342,10.5656467251638));
#54412=CARTESIAN_POINT('Ctrl Pts',(0.639804332264874,1.53828930197729,10.5611680420818));
#54413=CARTESIAN_POINT('Ctrl Pts',(0.650217718205162,1.53391670632844,10.5604233531644));
#54414=CARTESIAN_POINT('Ctrl Pts',(0.666425727905554,1.52691624539809,10.5592496604774));
#54415=CARTESIAN_POINT('Ctrl Pts',(0.672251347977826,1.52436038817974,10.5588248223568));
#54416=CARTESIAN_POINT('Ctrl Pts',(0.682574558086989,1.51976063179552,10.5580664390523));
#54417=CARTESIAN_POINT('Ctrl Pts',(0.6870778965152,1.51773000468157,10.5577336990412));
#54418=CARTESIAN_POINT('Ctrl Pts',(0.697935688195287,1.51277582639699,10.5569268622724));
#54419=CARTESIAN_POINT('Ctrl Pts',(0.704280772177505,1.50983228051747,10.5564515712062));
#54420=CARTESIAN_POINT('Ctrl Pts',(0.723953201491947,1.50055506273643,10.5549665725276));
#54421=CARTESIAN_POINT('Ctrl Pts',(0.737214645381597,1.49408442316629,10.553949158589));
#54422=CARTESIAN_POINT('Ctrl Pts',(0.805477781673791,1.45964682060626,10.5486332539399));
#54423=CARTESIAN_POINT('Ctrl Pts',(0.858975985885196,1.4288184068559,10.5442011523411));
#54424=CARTESIAN_POINT('Ctrl Pts',(1.03647726335709,1.31295630494219,10.5288309553361));
#54425=CARTESIAN_POINT('Ctrl Pts',(1.15065778877938,1.21414339287638,10.517835120579));
#54426=CARTESIAN_POINT('Ctrl Pts',(1.26373953107352,1.08579360466303,10.5060725850247));
#54427=CARTESIAN_POINT('Ctrl Pts',(1.27714671317399,1.06999144591394,10.5046594923316));
#54428=CARTESIAN_POINT('Ctrl Pts',(1.29815471631044,1.0442730585435,10.5024141405338));
#54429=CARTESIAN_POINT('Ctrl Pts',(1.30594452139081,1.03451477034371,10.5015743359043));
#54430=CARTESIAN_POINT('Ctrl Pts',(1.3196372919869,1.01696066979632,10.5000847423281));
#54431=CARTESIAN_POINT('Ctrl Pts',(1.32558263846188,1.00919882180214,10.499433291326));
#54432=CARTESIAN_POINT('Ctrl Pts',(1.33793021902309,0.992781256683607,10.4980701482177));
#54433=CARTESIAN_POINT('Ctrl Pts',(1.34431759315388,0.984114887860952,10.4973590562378));
#54434=CARTESIAN_POINT('Ctrl Pts',(1.36103348963873,0.960968348136668,10.4954816637705));
#54435=CARTESIAN_POINT('Ctrl Pts',(1.3712150868309,0.946383406090704,10.4943210075649));
#54436=CARTESIAN_POINT('Ctrl Pts',(1.42357907714352,0.868753310221009,10.4882541323983));
#54437=CARTESIAN_POINT('Ctrl Pts',(1.46165546770604,0.803041165726937,10.483502946441));
#54438=CARTESIAN_POINT('Ctrl Pts',(1.54149128500431,0.640630693427758,10.4723464447573));
#54439=CARTESIAN_POINT('Ctrl Pts',(1.57882549497222,0.542135612906083,10.4660408722851));
#54440=CARTESIAN_POINT('Ctrl Pts',(1.61892963417412,0.395958991533776,10.4565743676173));
#54441=CARTESIAN_POINT('Ctrl Pts',(1.62934537289206,0.350641533556574,10.4536226759825));
#54442=CARTESIAN_POINT('Ctrl Pts',(1.63984025591783,0.294275207549444,10.4498648335958));
#54443=CARTESIAN_POINT('Ctrl Pts',(1.64172379131339,0.283578808034988,10.4491479147204));
#54444=CARTESIAN_POINT('Ctrl Pts',(1.64451823989629,0.266747475550451,10.4480127400516));
#54445=CARTESIAN_POINT('Ctrl Pts',(1.64549974340452,0.260624343426591,10.4475983065123));
#54446=CARTESIAN_POINT('Ctrl Pts',(1.64729163037781,0.249031835206956,10.4468106756429));
#54447=CARTESIAN_POINT('Ctrl Pts',(1.64810900049549,0.243563727265705,10.4464378680942));
#54448=CARTESIAN_POINT('Ctrl Pts',(1.64998630900513,0.230562469279665,10.4455485069081));
#54449=CARTESIAN_POINT('Ctrl Pts',(1.65102188576581,0.223026005724653,10.4450306311319));
#54450=CARTESIAN_POINT('Ctrl Pts',(1.65436405447699,0.197403174146386,10.4432625954017));
#54451=CARTESIAN_POINT('Ctrl Pts',(1.65642524502749,0.179286858639511,10.4420001374996));
#54452=CARTESIAN_POINT('Ctrl Pts',(1.66077883916317,0.134487174555217,10.4388534931753));
#54453=CARTESIAN_POINT('Ctrl Pts',(1.66272587975138,0.107775887327628,10.4369558073158));
#54454=CARTESIAN_POINT('Ctrl Pts',(1.66853185680683,-0.0114541294322638,
10.428420284254));
#54455=CARTESIAN_POINT('Ctrl Pts',(1.66531735322964,-0.104151559382932,
10.4216210645194));
#54456=CARTESIAN_POINT('Ctrl Pts',(1.64328831539891,-0.290001190951868,
10.4080751717489));
#54457=CARTESIAN_POINT('Ctrl Pts',(1.6241827012998,-0.382796516104936,10.4013589210312));
#54458=CARTESIAN_POINT('Ctrl Pts',(1.59194549884264,-0.491549189958379,
10.3936035201721));
#54459=CARTESIAN_POINT('Ctrl Pts',(1.58628380419756,-0.509524111874708,
10.3923250235971));
#54460=CARTESIAN_POINT('Ctrl Pts',(1.57683847884317,-0.537826398018662,
10.3903165069736));
#54461=CARTESIAN_POINT('Ctrl Pts',(1.57325562463237,-0.548218544335189,
10.3895799854177));
#54462=CARTESIAN_POINT('Ctrl Pts',(1.56663364266792,-0.566826019985522,
10.3882627172603));
#54463=CARTESIAN_POINT('Ctrl Pts',(1.563632111927,-0.57505419816941,10.3876807549634));
#54464=CARTESIAN_POINT('Ctrl Pts',(1.55642795541582,-0.594329632513051,
10.3863184860453));
#54465=CARTESIAN_POINT('Ctrl Pts',(1.55217234317064,-0.605356689583083,
10.3855399742696));
#54466=CARTESIAN_POINT('Ctrl Pts',(1.53935026876353,-0.637556569767095,
10.3832683048517));
#54467=CARTESIAN_POINT('Ctrl Pts',(1.53046513894832,-0.658600159293423,
10.3817858431087));
#54468=CARTESIAN_POINT('Ctrl Pts',(1.48738175601694,-0.755054306929365,
10.3749902717327));
#54469=CARTESIAN_POINT('Ctrl Pts',(1.44802322456057,-0.82803536018141,10.369854072376));
#54470=CARTESIAN_POINT('Ctrl Pts',(1.37255838166571,-0.945999049889552,
10.3612689968606));
#54471=CARTESIAN_POINT('Ctrl Pts',(1.33925732218618,-0.99258272285283,10.3577927978951));
#54472=CARTESIAN_POINT('Ctrl Pts',(1.25570458371164,-1.09758144470337,10.3495576638826));
#54473=CARTESIAN_POINT('Ctrl Pts',(1.20367422713917,-1.15440212486887,10.3447804511836));
#54474=CARTESIAN_POINT('Ctrl Pts',(1.1395024236288,-1.21541140023655,10.3389888532485));
#54475=CARTESIAN_POINT('Ctrl Pts',(1.13100976875244,-1.22331824549376,10.3382241815778));
#54476=CARTESIAN_POINT('Ctrl Pts',(1.11768327242383,-1.23546811297546,10.337025729378));
#54477=CARTESIAN_POINT('Ctrl Pts',(1.11290608752657,-1.2397731213864,10.3365964017093));
#54478=CARTESIAN_POINT('Ctrl Pts',(1.10401186422665,-1.24769541069684,10.3357973307104));
#54479=CARTESIAN_POINT('Ctrl Pts',(1.09990175724881,-1.25132016504145,10.3354281493976));
#54480=CARTESIAN_POINT('Ctrl Pts',(1.09034300104577,-1.25966667103941,10.3345697801022));
#54481=CARTESIAN_POINT('Ctrl Pts',(1.08488153119255,-1.26437337859423,10.3340795340737));
#54482=CARTESIAN_POINT('Ctrl Pts',(1.06726214140492,-1.27935960772184,10.3324990251892));
#54483=CARTESIAN_POINT('Ctrl Pts',(1.05498777225002,-1.28949999551867,10.331399626505));
#54484=CARTESIAN_POINT('Ctrl Pts',(1.02517235629961,-1.31342117496283,10.3287367794479));
#54485=CARTESIAN_POINT('Ctrl Pts',(1.00749644154243,-1.32702839565862,10.3271643460276));
#54486=CARTESIAN_POINT('Ctrl Pts',(0.936851514025167,-1.37918701540653,
10.3209200153979));
#54487=CARTESIAN_POINT('Ctrl Pts',(0.881902963949549,-1.41495365485163,
10.3161522174584));
#54488=CARTESIAN_POINT('Ctrl Pts',(0.719059492045232,-1.50777243766725,
10.3025077605635));
#54489=CARTESIAN_POINT('Ctrl Pts',(0.606796047528954,-1.55635252708872,
10.2937000344992));
#54490=CARTESIAN_POINT('Ctrl Pts',(0.470211811428143,-1.59840390566161,
10.2838700771653));
#54491=CARTESIAN_POINT('Ctrl Pts',(0.450090416030545,-1.60418604895799,
10.2824421912624));
#54492=CARTESIAN_POINT('Ctrl Pts',(0.417743744655853,-1.61282471357215,
10.2801781055908));
#54493=CARTESIAN_POINT('Ctrl Pts',(0.405586462687128,-1.61592482162347,
10.2793341588286));
#54494=CARTESIAN_POINT('Ctrl Pts',(0.383886839600371,-1.62119790233165,
10.2778398648467));
#54495=CARTESIAN_POINT('Ctrl Pts',(0.37435831104621,-1.62342465366125,10.2771878179438));
#54496=CARTESIAN_POINT('Ctrl Pts',(0.354336484933997,-1.62791796063293,
10.275826070119));
#54497=CARTESIAN_POINT('Ctrl Pts',(0.343839755493118,-1.63016731127452,
10.2751169462049));
#54498=CARTESIAN_POINT('Ctrl Pts',(0.316036757655364,-1.63584473563991,
10.2732508311237));
#54499=CARTESIAN_POINT('Ctrl Pts',(0.298696221749054,-1.63909970323242,
10.2720993606642));
#54500=CARTESIAN_POINT('Ctrl Pts',(0.209036410039491,-1.65445944537256,
10.2662043979341));
#54501=CARTESIAN_POINT('Ctrl Pts',(0.136022668791075,-1.66205657727013,
10.2616049543371));
#54502=CARTESIAN_POINT('Ctrl Pts',(-0.0355262246515348,-1.66852135373109,
10.2510090765229));
#54503=CARTESIAN_POINT('Ctrl Pts',(-0.133921419902664,-1.66351722365645,
10.2450965467666));
#54504=CARTESIAN_POINT('Ctrl Pts',(-0.264249661837201,-1.64524626985364,
10.2369313986337));
#54505=CARTESIAN_POINT('Ctrl Pts',(-0.297054054106251,-1.63964075832284,
10.2348460701389));
#54506=CARTESIAN_POINT('Ctrl Pts',(-0.355457843579343,-1.6278507340082,
10.2310449034782));
#54507=CARTESIAN_POINT('Ctrl Pts',(-0.381120338374965,-1.6220343383052,
10.2293435483973));
#54508=CARTESIAN_POINT('Ctrl Pts',(-0.415376433943941,-1.613412444456,10.227017274837));
#54509=CARTESIAN_POINT('Ctrl Pts',(-0.424102012507536,-1.61114082926893,
10.2264198779463));
#54510=CARTESIAN_POINT('Ctrl Pts',(-0.43785222009138,-1.6074416673281,10.2254701539325));
#54511=CARTESIAN_POINT('Ctrl Pts',(-0.442889465352447,-1.60606108230223,
10.2251204614575));
#54512=CARTESIAN_POINT('Ctrl Pts',(-0.453345272968204,-1.60314247336473,
10.2243907587088));
#54513=CARTESIAN_POINT('Ctrl Pts',(-0.458762609777383,-1.6016006339314,
10.2240105162271));
#54514=CARTESIAN_POINT('Ctrl Pts',(-0.472060448823053,-1.59774290776513,
10.2230719594518));
#54515=CARTESIAN_POINT('Ctrl Pts',(-0.479931779706434,-1.59539617226091,
10.2225119182922));
#54516=CARTESIAN_POINT('Ctrl Pts',(-0.509047531882594,-1.58648072305025,
10.2204245024478));
#54517=CARTESIAN_POINT('Ctrl Pts',(-0.530176110913511,-1.57954539267471,
10.2188783366942));
#54518=CARTESIAN_POINT('Ctrl Pts',(-0.688136346235638,-1.52416970496632,
10.2071130849968));
#54519=CARTESIAN_POINT('Ctrl Pts',(-0.81825125996781,-1.45845578252264,
10.1963154800243));
#54520=CARTESIAN_POINT('Ctrl Pts',(-0.992426767600683,-1.3397574755361,
10.1812603762908));
#54521=CARTESIAN_POINT('Ctrl Pts',(-1.04442115794302,-1.29963355517777,
10.1766627759453));
#54522=CARTESIAN_POINT('Ctrl Pts',(-1.1072642679773,-1.24492365990061,10.1709759002014));
#54523=CARTESIAN_POINT('Ctrl Pts',(-1.12042405825076,-1.23309328509323,
10.1697769692047));
#54524=CARTESIAN_POINT('Ctrl Pts',(-1.14126920789528,-1.21374464662334,
10.1678640330061));
#54525=CARTESIAN_POINT('Ctrl Pts',(-1.14907432399157,-1.20635802289323,
10.1671445429376));
#54526=CARTESIAN_POINT('Ctrl Pts',(-1.16384689178002,-1.19210406343739,
10.165776305619));
#54527=CARTESIAN_POINT('Ctrl Pts',(-1.17082636543591,-1.18524989539507,
10.1651270309301));
#54528=CARTESIAN_POINT('Ctrl Pts',(-1.17804979590416,-1.17803007764691,
10.1644519459491));
#54529=CARTESIAN_POINT('Ctrl Pts',(-1.17835427897449,-1.1777255107595,10.1644234838322));
#54530=CARTESIAN_POINT('Ctrl Pts',(-1.17895143575263,-1.17712772619244,
10.1643676520178));
#54531=CARTESIAN_POINT('Ctrl Pts',(-1.17924411823485,-1.17683451735714,
10.1643402819368));
#54532=CARTESIAN_POINT('Ctrl Pts',(-1.17981941313689,-1.17625775774524,
10.1642864727945));
#54533=CARTESIAN_POINT('Ctrl Pts',(-1.18010203276548,-1.17597421422997,
10.1642600334187));
#54534=CARTESIAN_POINT('Ctrl Pts',(-1.18065873073384,-1.17541529362739,
10.1642079436958));
#54535=CARTESIAN_POINT('Ctrl Pts',(-1.18093281498866,-1.17513992249204,
10.1641822930911));
#54536=CARTESIAN_POINT('Ctrl Pts',(-1.18147379968419,-1.17459601736338,
10.1641316547117));
#54537=CARTESIAN_POINT('Ctrl Pts',(-1.18174070495256,-1.17432748822666,
10.164106666727));
#54538=CARTESIAN_POINT('Ctrl Pts',(-1.19026300994896,-1.16574748524836,
10.163308652557));
#54539=CARTESIAN_POINT('Ctrl Pts',(-1.19843077735734,-1.15734908981982,
10.1625394637603));
#54540=CARTESIAN_POINT('Ctrl Pts',(-1.22663276611044,-1.1277320640116,10.1598672343591));
#54541=CARTESIAN_POINT('Ctrl Pts',(-1.24619825585961,-1.10607306403677,
10.1579840837568));
#54542=CARTESIAN_POINT('Ctrl Pts',(-1.29193757900133,-1.0526841966272,10.1534967572877));
#54543=CARTESIAN_POINT('Ctrl Pts',(-1.31752553662098,-1.02047711461148,
10.150914488051));
#54544=CARTESIAN_POINT('Ctrl Pts',(-1.39298158149786,-0.917926056802289,
10.1430056288141));
#54545=CARTESIAN_POINT('Ctrl Pts',(-1.43860090400361,-0.844638211444959,
10.1377919984518));
#54546=CARTESIAN_POINT('Ctrl Pts',(-1.5150494001073,-0.697508779990399,
10.1276252951632));
#54547=CARTESIAN_POINT('Ctrl Pts',(-1.54663881374471,-0.624338186244144,
10.1226931331175));
#54548=CARTESIAN_POINT('Ctrl Pts',(-1.57670541841323,-0.538229587135547,
10.116727646752));
#54549=CARTESIAN_POINT('Ctrl Pts',(-1.5804215136236,-0.527218062670438,
10.1159618085966));
#54550=CARTESIAN_POINT('Ctrl Pts',(-1.58601565604507,-0.510050728955306,
10.114761911908));
#54551=CARTESIAN_POINT('Ctrl Pts',(-1.5879738305639,-0.503921141942606,
10.1143323232592));
#54552=CARTESIAN_POINT('Ctrl Pts',(-1.59153369951653,-0.492551024147773,
10.1135330316411));
#54553=CARTESIAN_POINT('Ctrl Pts',(-1.593145107703,-0.487313749764808,10.1131638935963));
#54554=CARTESIAN_POINT('Ctrl Pts',(-1.5968151420117,-0.475172914484262,
10.1123059765617));
#54555=CARTESIAN_POINT('Ctrl Pts',(-1.59885484861613,-0.46826388356232,
10.1118161434898));
#54556=CARTESIAN_POINT('Ctrl Pts',(-1.60524934620423,-0.446075075594156,
10.1102383249954));
#54557=CARTESIAN_POINT('Ctrl Pts',(-1.60943023850302,-0.430746674869565,
10.1091412456697));
#54558=CARTESIAN_POINT('Ctrl Pts',(-1.64820379414772,-0.28013834405567,
10.0983080807256));
#54559=CARTESIAN_POINT('Ctrl Pts',(-1.66587635268669,-0.141086637584619,
10.0879378005138));
#54560=CARTESIAN_POINT('Ctrl Pts',(-1.66599935349477,-0.0014677039958931,
10.0778956387897));
#54561=CARTESIAN_POINT('Ctrl Pts',(-1.66599935485773,-0.00146615606807475,
10.0778955274543));
#54562=CARTESIAN_POINT('Ctrl Pts',(-1.66604451061792,0.0498445256343925,
10.0742049818099));
#54563=CARTESIAN_POINT('Ctrl Pts',(-1.66371921130138,0.101134532714982,
10.0705587717341));
#54564=CARTESIAN_POINT('Ctrl Pts',(-1.65643808135581,0.180480131690436,
10.0649991798008));
#54565=CARTESIAN_POINT('Ctrl Pts',(-1.65312593791863,0.208650415156738,
10.0630410675269));
#54566=CARTESIAN_POINT('Ctrl Pts',(-1.64723819627737,0.249666341968592,
10.060212325594));
#54567=CARTESIAN_POINT('Ctrl Pts',(-1.64522800177558,0.262586741225869,
10.0593244752333));
#54568=CARTESIAN_POINT('Ctrl Pts',(-1.6414516794009,0.285109940362668,10.0577821230972));
#54569=CARTESIAN_POINT('Ctrl Pts',(-1.63975288551601,0.294723218267103,
10.0571255380111));
#54570=CARTESIAN_POINT('Ctrl Pts',(-1.63616171736016,0.314052218965795,
10.0558086504158));
#54571=CARTESIAN_POINT('Ctrl Pts',(-1.63426705928971,0.32376711968777,10.0551484494935));
#54572=CARTESIAN_POINT('Ctrl Pts',(-1.63019778812774,0.343685909006897,
10.0537980276507));
#54573=CARTESIAN_POINT('Ctrl Pts',(-1.62801367594708,0.35388742810494,10.0531081412161));
#54574=CARTESIAN_POINT('Ctrl Pts',(-1.62218781495125,0.379902624331914,
10.0513528795156));
#54575=CARTESIAN_POINT('Ctrl Pts',(-1.61841053607833,0.395685074290687,
10.0502918661254));
#54576=CARTESIAN_POINT('Ctrl Pts',(-1.60212869295147,0.459576182438404,
10.0460092657414));
#54577=CARTESIAN_POINT('Ctrl Pts',(-1.58770408784237,0.507171633669777,
10.0428492217377));
#54578=CARTESIAN_POINT('Ctrl Pts',(-1.5686401382185,0.561232615627931,10.0392603670108));
#54579=CARTESIAN_POINT('Ctrl Pts',(-1.56606003411924,0.568392357912186,
10.0387850497008));
#54580=CARTESIAN_POINT('Ctrl Pts',(-1.56343130417499,0.575533280641269,
10.0383108307813));
#54581=CARTESIAN_POINT('',(-1.66599992285883,0.000506985575740082,10.2730004785459));
#54582=CARTESIAN_POINT('Ctrl Pts',(-1.56343128570986,0.575533330801617,
10.2310772794004));
#54583=CARTESIAN_POINT('Ctrl Pts',(-1.57769043289253,0.536798481541238,
10.2340278998061));
#54584=CARTESIAN_POINT('Ctrl Pts',(-1.59050792609994,0.497539507700919,
10.2370180206381));
#54585=CARTESIAN_POINT('Ctrl Pts',(-1.6363410722794,0.337181098515292,10.2491421604763));
#54586=CARTESIAN_POINT('Ctrl Pts',(-1.65708987690961,0.212993145401417,
10.2582884449228));
#54587=CARTESIAN_POINT('Ctrl Pts',(-1.66522185482676,0.0586221925312235,
10.2690299316985));
#54588=CARTESIAN_POINT('Ctrl Pts',(-1.665991079245,0.0295678911884265,10.2710268732202));
#54589=CARTESIAN_POINT('Ctrl Pts',(-1.66599992285883,0.000506985575740082,
10.2730004785459));
#54590=CARTESIAN_POINT('Ctrl Pts',(-1.66599992316667,0.000505972977507134,
10.2730005473142));
#54591=CARTESIAN_POINT('Ctrl Pts',(-1.66600231739398,-0.00737741743330579,
10.2735359296996));
#54592=CARTESIAN_POINT('Ctrl Pts',(-1.66594875621251,-0.0152608683665852,
10.2740695753403));
#54593=CARTESIAN_POINT('Ctrl Pts',(-1.6657174916656,-0.0319067840115265,
10.2751927750027));
#54594=CARTESIAN_POINT('Ctrl Pts',(-1.66552660043235,-0.04066882409478,
10.2757818989175));
#54595=CARTESIAN_POINT('Ctrl Pts',(-1.66499291961764,-0.0586485338171585,
10.276986600463));
#54596=CARTESIAN_POINT('Ctrl Pts',(-1.66464270229388,-0.0678656944789535,
10.277601924675));
#54597=CARTESIAN_POINT('Ctrl Pts',(-1.66373873333539,-0.0873831661284348,
10.2789002997265));
#54598=CARTESIAN_POINT('Ctrl Pts',(-1.66316583041524,-0.0976822356759736,
10.2795827254178));
#54599=CARTESIAN_POINT('Ctrl Pts',(-1.66148205488959,-0.123607299753442,
10.2812941155429));
#54600=CARTESIAN_POINT('Ctrl Pts',(-1.66024636027905,-0.13922440104548,
10.2823191507774));
#54601=CARTESIAN_POINT('Ctrl Pts',(-1.65461640934936,-0.199544623175656,
10.2862580216255));
#54602=CARTESIAN_POINT('Ctrl Pts',(-1.64863511964054,-0.244082586298848,
10.2891225228046));
#54603=CARTESIAN_POINT('Ctrl Pts',(-1.6152777470171,-0.43391801524496,10.3012359628447));
#54604=CARTESIAN_POINT('Ctrl Pts',(-1.57043610681048,-0.575440724368906,
10.3099627622332));
#54605=CARTESIAN_POINT('Ctrl Pts',(-1.49591934339789,-0.733841893602513,
10.3209597415386));
#54606=CARTESIAN_POINT('Ctrl Pts',(-1.4837165807553,-0.758210754916007,
10.3226909143782));
#54607=CARTESIAN_POINT('Ctrl Pts',(-1.46225120392947,-0.798572759528369,
10.3256431019065));
#54608=CARTESIAN_POINT('Ctrl Pts',(-1.45330991405886,-0.81473140378043,
10.3268485324409));
#54609=CARTESIAN_POINT('Ctrl Pts',(-1.4402898165524,-0.837364737272315,
10.3285753807705));
#54610=CARTESIAN_POINT('Ctrl Pts',(-1.43643179415618,-0.843965730327751,
10.3290837162452));
#54611=CARTESIAN_POINT('Ctrl Pts',(-1.42970284416014,-0.855299019365696,
10.3299650364177));
#54612=CARTESIAN_POINT('Ctrl Pts',(-1.42685353924176,-0.860043959234143,
10.3303366399452));
#54613=CARTESIAN_POINT('Ctrl Pts',(-1.42077102197167,-0.87005973095406,
10.3311267377867));
#54614=CARTESIAN_POINT('Ctrl Pts',(-1.41753214669269,-0.87532670601818,
10.3315455703305));
#54615=CARTESIAN_POINT('Ctrl Pts',(-1.40856811430863,-0.889723552486969,
10.3326993605331));
#54616=CARTESIAN_POINT('Ctrl Pts',(-1.40278369205506,-0.898815904698617,
10.3334379797107));
#54617=CARTESIAN_POINT('Ctrl Pts',(-1.37231307019707,-0.945701084986023,
10.3372960347145));
#54618=CARTESIAN_POINT('Ctrl Pts',(-1.34618855269544,-0.982532087505519,
10.3404942129081));
#54619=CARTESIAN_POINT('Ctrl Pts',(-1.26433631065196,-1.08852799167126,
10.350109502701));
#54620=CARTESIAN_POINT('Ctrl Pts',(-1.20453844770308,-1.15435118152197,
10.3566255637043));
#54621=CARTESIAN_POINT('Ctrl Pts',(-1.07820786925432,-1.27285139244742,
10.3691507056581));
#54622=CARTESIAN_POINT('Ctrl Pts',(-1.01232742304659,-1.32585061739875,
10.3751512299512));
#54623=CARTESIAN_POINT('Ctrl Pts',(-0.923701412872644,-1.38667329308936,
10.3825429577679));
#54624=CARTESIAN_POINT('Ctrl Pts',(-0.904430381614241,-1.39931872671803,
10.3841132239525));
#54625=CARTESIAN_POINT('Ctrl Pts',(-0.87485304270165,-1.41786065235273,
10.3864691416193));
#54626=CARTESIAN_POINT('Ctrl Pts',(-0.864736570333892,-1.42405314239243,
10.3872656160984));
#54627=CARTESIAN_POINT('Ctrl Pts',(-0.847032371913599,-1.43463199039787,
10.3886436530887));
#54628=CARTESIAN_POINT('Ctrl Pts',(-0.839474679794697,-1.439067425092,10.3892269854162));
#54629=CARTESIAN_POINT('Ctrl Pts',(-0.822383113957587,-1.44891760188876,
10.3905353145224));
#54630=CARTESIAN_POINT('Ctrl Pts',(-0.812830015027769,-1.45429831174043,
10.3912590660205));
#54631=CARTESIAN_POINT('Ctrl Pts',(-0.786832817720502,-1.46860483632872,
10.3932089229169));
#54632=CARTESIAN_POINT('Ctrl Pts',(-0.77029003650322,-1.47734875838842,
10.3944285641664));
#54633=CARTESIAN_POINT('Ctrl Pts',(-0.666783350087545,-1.52984726864472,
10.4019373649262));
#54634=CARTESIAN_POINT('Ctrl Pts',(-0.576266493608423,-1.56619066123537,
10.4079594855773));
#54635=CARTESIAN_POINT('Ctrl Pts',(-0.415422537318817,-1.61492362266278,
10.4182441028165));
#54636=CARTESIAN_POINT('Ctrl Pts',(-0.346528060957935,-1.63109529875563,
10.4225305617474));
#54637=CARTESIAN_POINT('Ctrl Pts',(-0.238595163156672,-1.64928189056236,
10.4293148733688));
#54638=CARTESIAN_POINT('Ctrl Pts',(-0.200162399428393,-1.65438599627872,
10.4317445913411));
#54639=CARTESIAN_POINT('Ctrl Pts',(-0.137993412992661,-1.6604444806956,
10.4357462387257));
#54640=CARTESIAN_POINT('Ctrl Pts',(-0.114352530539566,-1.66223987906268,
10.4372844823368));
#54641=CARTESIAN_POINT('Ctrl Pts',(-0.0822813354591848,-1.66398815431015,
10.4394033849361));
#54642=CARTESIAN_POINT('Ctrl Pts',(-0.0738766537231008,-1.66438247661131,
10.4399616556576));
#54643=CARTESIAN_POINT('Ctrl Pts',(-0.0598021060484204,-1.66493599814267,
10.440902075835));
#54644=CARTESIAN_POINT('Ctrl Pts',(-0.0541336146227459,-1.66512994091761,
10.4412823311622));
#54645=CARTESIAN_POINT('Ctrl Pts',(-0.0425698921484775,-1.66546647451406,
10.4420613131198));
#54646=CARTESIAN_POINT('Ctrl Pts',(-0.0366747324390218,-1.66560671669856,
10.4424601514394));
#54647=CARTESIAN_POINT('Ctrl Pts',(-0.0213120945399635,-1.66589058729547,
10.4435037669758));
#54648=CARTESIAN_POINT('Ctrl Pts',(-0.0118440763266761,-1.6659848023095,
10.4441511564931));
#54649=CARTESIAN_POINT('Ctrl Pts',(0.0277042310925202,-1.66604120622537,
10.4468714940803));
#54650=CARTESIAN_POINT('Ctrl Pts',(0.0577779916927537,-1.66526942561437,
10.4489791126753));
#54651=CARTESIAN_POINT('Ctrl Pts',(0.113590959686809,-1.66232352407493,
10.4529439991073));
#54652=CARTESIAN_POINT('Ctrl Pts',(0.139333761767613,-1.66036393547833,
10.4547939485429));
#54653=CARTESIAN_POINT('Ctrl Pts',(0.266480985432943,-1.64770759362963,
10.4640074078436));
#54654=CARTESIAN_POINT('Ctrl Pts',(0.366808460838594,-1.62831378542954,
10.4715013816703));
#54655=CARTESIAN_POINT('Ctrl Pts',(0.534401804488663,-1.5796309995296,10.4840098652485));
#54656=CARTESIAN_POINT('Ctrl Pts',(0.602682416379695,-1.55486201721768,
10.4891072599739));
#54657=CARTESIAN_POINT('Ctrl Pts',(0.685253899559558,-1.51864832347157,
10.4952602072844));
#54658=CARTESIAN_POINT('Ctrl Pts',(0.701256240852304,-1.51132569724481,
10.4964523938551));
#54659=CARTESIAN_POINT('Ctrl Pts',(0.72682083540509,-1.49913391795845,10.4983572439567));
#54660=CARTESIAN_POINT('Ctrl Pts',(0.736456941472921,-1.49442370611996,
10.4990753090867));
#54661=CARTESIAN_POINT('Ctrl Pts',(0.754798944689003,-1.48523747612596,
10.5004425102007));
#54662=CARTESIAN_POINT('Ctrl Pts',(0.763512158371822,-1.48077716027341,
10.50109215781));
#54663=CARTESIAN_POINT('Ctrl Pts',(0.783320489724964,-1.47041589910944,
10.5025697222322));
#54664=CARTESIAN_POINT('Ctrl Pts',(0.79438925399797,-1.46446564776934,10.5033958644325));
#54665=CARTESIAN_POINT('Ctrl Pts',(0.823776648428824,-1.44823658637119,
10.5055914170822));
#54666=CARTESIAN_POINT('Ctrl Pts',(0.841970354458956,-1.4377354283724,10.5069529292663));
#54667=CARTESIAN_POINT('Ctrl Pts',(0.963391453077724,-1.36455722172156,
10.5160670344918));
#54668=CARTESIAN_POINT('Ctrl Pts',(1.05973955372423,-1.29116049709134,10.5234020613916));
#54669=CARTESIAN_POINT('Ctrl Pts',(1.19538407275145,-1.16232878033086,10.5348331747996));
#54670=CARTESIAN_POINT('Ctrl Pts',(1.24068317830539,-1.11384705307276,10.5388951779501));
#54671=CARTESIAN_POINT('Ctrl Pts',(1.29729686277346,-1.04550524030338,10.5445119402044));
#54672=CARTESIAN_POINT('Ctrl Pts',(1.31127167967211,-1.02792355703174,10.5459482107291));
#54673=CARTESIAN_POINT('Ctrl Pts',(1.33458833153797,-0.99733949774668,10.5484423841564));
#54674=CARTESIAN_POINT('Ctrl Pts',(1.34410621671358,-0.984474743453597,
10.5494902782853));
#54675=CARTESIAN_POINT('Ctrl Pts',(1.35764977824141,-0.965606170684461,
10.5510286510707));
#54676=CARTESIAN_POINT('Ctrl Pts',(1.36182435131569,-0.959709658472877,
10.5515095996445));
#54677=CARTESIAN_POINT('Ctrl Pts',(1.36907070962736,-0.949331822358583,
10.5523567755868));
#54678=CARTESIAN_POINT('Ctrl Pts',(1.37215912709303,-0.944862342160033,
10.5527218733202));
#54679=CARTESIAN_POINT('Ctrl Pts',(1.37883865700368,-0.935094074587906,
10.5535204291737));
#54680=CARTESIAN_POINT('Ctrl Pts',(1.38242105458173,-0.929789758374915,
10.5539544175496));
#54681=CARTESIAN_POINT('Ctrl Pts',(1.392336356158,-0.914924580279304,10.555171364952));
#54682=CARTESIAN_POINT('Ctrl Pts',(1.39860109487848,-0.90531899101855,10.5559585436493));
#54683=CARTESIAN_POINT('Ctrl Pts',(1.44003794386071,-0.840328106734557,
10.5612859709902));
#54684=CARTESIAN_POINT('Ctrl Pts',(1.4720073938494,-0.782976959801305,10.5659919335387));
#54685=CARTESIAN_POINT('Ctrl Pts',(1.50967435092355,-0.704900182846258,
10.5722755538515));
#54686=CARTESIAN_POINT('Ctrl Pts',(1.51847780466338,-0.68573030582163,10.573809216254));
#54687=CARTESIAN_POINT('Ctrl Pts',(1.5542528193068,-0.603759253145454,10.5803179177953));
#54688=CARTESIAN_POINT('Ctrl Pts',(1.5777117938742,-0.539493715143421,10.5852961966818));
#54689=CARTESIAN_POINT('Ctrl Pts',(1.61067252348948,-0.428423639548609,
10.5935953483652));
#54690=CARTESIAN_POINT('Ctrl Pts',(1.62223439333167,-0.382320608545958,
10.5969559058095));
#54691=CARTESIAN_POINT('Ctrl Pts',(1.63838388006684,-0.303838606504144,
10.6025265531334));
#54692=CARTESIAN_POINT('Ctrl Pts',(1.64401808229459,-0.271706533246437,
10.6047659871326));
#54693=CARTESIAN_POINT('Ctrl Pts',(1.65065426618434,-0.226009594290692,
10.6078946149127));
#54694=CARTESIAN_POINT('Ctrl Pts',(1.65243903747961,-0.212567846757036,
10.6088081023518));
#54695=CARTESIAN_POINT('Ctrl Pts',(1.65524357020508,-0.189269318118188,
10.6103801021523));
#54696=CARTESIAN_POINT('Ctrl Pts',(1.65633984319084,-0.179422636934863,
10.6110409857462));
#54697=CARTESIAN_POINT('Ctrl Pts',(1.65840828152017,-0.159205665583671,
10.6123909791254));
#54698=CARTESIAN_POINT('Ctrl Pts',(1.65937116652569,-0.14883484876422,10.6130797699055));
#54699=CARTESIAN_POINT('Ctrl Pts',(1.66157837221135,-0.122367973206287,
10.6148285276571));
#54700=CARTESIAN_POINT('Ctrl Pts',(1.66268612743982,-0.106261372987656,
10.6158841981877));
#54701=CARTESIAN_POINT('Ctrl Pts',(1.66620899337148,-0.0412464035442574,
10.620113959611));
#54702=CARTESIAN_POINT('Ctrl Pts',(1.66670165240875,0.00774397952933208,
10.6232284822794));
#54703=CARTESIAN_POINT('Ctrl Pts',(1.66127268200489,0.16720114244251,10.6332230751237));
#54704=CARTESIAN_POINT('Ctrl Pts',(1.64651757434476,0.27706195808729,10.6398682726536));
#54705=CARTESIAN_POINT('Ctrl Pts',(1.60613883295747,0.447224588114197,10.6506321884736));
#54706=CARTESIAN_POINT('Ctrl Pts',(1.58768161977321,0.508878212068735,10.6546409052297));
#54707=CARTESIAN_POINT('Ctrl Pts',(1.56057052943083,0.583439688656357,10.6597953694081));
#54708=CARTESIAN_POINT('Ctrl Pts',(1.55523956802041,0.597504891159565,10.6607816286632));
#54709=CARTESIAN_POINT('Ctrl Pts',(1.54713198203958,0.618052031154743,10.662245667467));
#54710=CARTESIAN_POINT('Ctrl Pts',(1.54450330162264,0.624592050738987,10.6627151590068));
#54711=CARTESIAN_POINT('Ctrl Pts',(1.53995943249461,0.635692861299592,10.6635183488665));
#54712=CARTESIAN_POINT('Ctrl Pts',(1.53806530504006,0.640262121453006,10.6638507881532));
#54713=CARTESIAN_POINT('Ctrl Pts',(1.53370248675802,0.650655589164751,10.6646112358927));
#54714=CARTESIAN_POINT('Ctrl Pts',(1.5312210122152,0.656474083277997,10.6650399899589));
#54715=CARTESIAN_POINT('Ctrl Pts',(1.52428088533716,0.672493661534344,10.6662285684006));
#54716=CARTESIAN_POINT('Ctrl Pts',(1.51975311804168,0.682664182231136,10.6669923152537));
#54717=CARTESIAN_POINT('Ctrl Pts',(1.49277333547937,0.741668814636968,10.6714735511826));
#54718=CARTESIAN_POINT('Ctrl Pts',(1.46807259050383,0.789434307082179,10.6753025602115));
#54719=CARTESIAN_POINT('Ctrl Pts',(1.39091888631392,0.922446227848898,10.6863963762827));
#54720=CARTESIAN_POINT('Ctrl Pts',(1.33303273924989,1.00428472022224,10.6937454565943));
#54721=CARTESIAN_POINT('Ctrl Pts',(1.22067696851961,1.13616164795766,10.7061672406998));
#54722=CARTESIAN_POINT('Ctrl Pts',(1.16957280121252,1.18870420461285,10.7113126707277));
#54723=CARTESIAN_POINT('Ctrl Pts',(1.10206806355061,1.2495251106592,10.7175137197659));
#54724=CARTESIAN_POINT('Ctrl Pts',(1.08877893056966,1.26112152496551,10.7187086187532));
#54725=CARTESIAN_POINT('Ctrl Pts',(1.06710925401079,1.27943309764039,10.7206167308812));
#54726=CARTESIAN_POINT('Ctrl Pts',(1.05884387393308,1.28628180088746,10.7213353789613));
#54727=CARTESIAN_POINT('Ctrl Pts',(1.04291753403978,1.29922083557553,10.7227030201961));
#54728=CARTESIAN_POINT('Ctrl Pts',(1.03526800200861,1.30532445521796,10.7233525313084));
#54729=CARTESIAN_POINT('Ctrl Pts',(1.01768705017753,1.31910066059491,10.7248288734215));
#54730=CARTESIAN_POINT('Ctrl Pts',(1.00772174952041,1.32672920174228,10.7256539403676));
#54731=CARTESIAN_POINT('Ctrl Pts',(0.980896928925395,1.34678725182318,10.7278446008576));
#54732=CARTESIAN_POINT('Ctrl Pts',(0.963887284568795,1.35901289624771,10.7292023531369));
#54733=CARTESIAN_POINT('Ctrl Pts',(0.846446264646202,1.44010884978967,10.7383784289865));
#54734=CARTESIAN_POINT('Ctrl Pts',(0.738956249855005,1.49810957425059,10.7457709604885));
#54735=CARTESIAN_POINT('Ctrl Pts',(0.538700003263964,1.57932015887205,10.7589769753229));
#54736=CARTESIAN_POINT('Ctrl Pts',(0.448466242992239,1.60727183898405,10.7647590000626));
#54737=CARTESIAN_POINT('Ctrl Pts',(0.344706560141308,1.62999260911108,10.771703561903));
#54738=CARTESIAN_POINT('Ctrl Pts',(0.333018072325539,1.63242073674257,10.7724900774257));
#54739=CARTESIAN_POINT('Ctrl Pts',(0.314993897449877,1.63596338962739,10.7737108094161));
#54740=CARTESIAN_POINT('Ctrl Pts',(0.308675880467755,1.63716723793832,10.7741401981372));
#54741=CARTESIAN_POINT('Ctrl Pts',(0.296961626055338,1.63932907900742,10.7749393446692));
#54742=CARTESIAN_POINT('Ctrl Pts',(0.29156744141781,1.64029706472519,10.7753085399827));
#54743=CARTESIAN_POINT('Ctrl Pts',(0.279185561107272,1.64245598663259,10.7761587075954));
#54744=CARTESIAN_POINT('Ctrl Pts',(0.272194964657453,1.64362895513929,10.7766406524396));
#54745=CARTESIAN_POINT('Ctrl Pts',(0.249727745455846,1.64725152309702,10.7781953963066));
#54746=CARTESIAN_POINT('Ctrl Pts',(0.234224500375187,1.64952731603788,10.7792770623071));
#54747=CARTESIAN_POINT('Ctrl Pts',(0.128487510135252,1.66352833135523,10.7867041415661));
#54748=CARTESIAN_POINT('Ctrl Pts',(0.0374642063310759,1.66806143651587,
10.7933350484026));
#54749=CARTESIAN_POINT('Ctrl Pts',(-0.138880849423573,1.66239935415567,
10.8061779287301));
#54750=CARTESIAN_POINT('Ctrl Pts',(-0.223967896481416,1.65308822197952,
10.8123720110889));
#54751=CARTESIAN_POINT('Ctrl Pts',(-0.339341631203659,1.63138657463041,
10.8206468781927));
#54752=CARTESIAN_POINT('Ctrl Pts',(-0.370537260164742,1.62458525970883,
10.8228727331643));
#54753=CARTESIAN_POINT('Ctrl Pts',(-0.42511510497349,1.61103203180071,10.8267460471704));
#54754=CARTESIAN_POINT('Ctrl Pts',(-0.448580123170537,1.60465667392301,
10.8284044486489));
#54755=CARTESIAN_POINT('Ctrl Pts',(-0.483510713401975,1.59433998913135,
10.83086407774));
#54756=CARTESIAN_POINT('Ctrl Pts',(-0.495085645133136,1.59078371513181,
10.8316776191502));
#54757=CARTESIAN_POINT('Ctrl Pts',(-0.515792207536282,1.58417394225279,
10.83313058553));
#54758=CARTESIAN_POINT('Ctrl Pts',(-0.524937980937905,1.58116691197144,
10.8337714952928));
#54759=CARTESIAN_POINT('Ctrl Pts',(-0.544556947626232,1.57452742066514,
10.8351447579746));
#54760=CARTESIAN_POINT('Ctrl Pts',(-0.55502103608637,1.57086935393278,10.8358762332698));
#54761=CARTESIAN_POINT('Ctrl Pts',(-0.583114639097111,1.56073253964241,
10.8378379793589));
#54762=CARTESIAN_POINT('Ctrl Pts',(-0.600672720115562,1.5540595459307,10.8390617891867));
#54763=CARTESIAN_POINT('Ctrl Pts',(-0.708017085899768,1.51117186319131,
10.8465372717711));
#54764=CARTESIAN_POINT('Ctrl Pts',(-0.794622663703553,1.46748318879487,
10.852525737974));
#54765=CARTESIAN_POINT('Ctrl Pts',(-0.937072908165522,1.3792933641321,10.8627782224018));
#54766=CARTESIAN_POINT('Ctrl Pts',(-0.994760852658286,1.3382847395058,10.86706537434));
#54767=CARTESIAN_POINT('Ctrl Pts',(-1.07975849744114,1.26932232134072,10.8738497976444));
#54768=CARTESIAN_POINT('Ctrl Pts',(-1.10898708882771,1.2438668778189,10.8762788648574));
#54769=CARTESIAN_POINT('Ctrl Pts',(-1.14909068465635,1.20640248530941,10.8797947452555));
#54770=CARTESIAN_POINT('Ctrl Pts',(-1.16072055394583,1.19521718194735,10.8808374947491));
#54771=CARTESIAN_POINT('Ctrl Pts',(-1.18102402996743,1.17511401172272,10.8827035146304));
#54772=CARTESIAN_POINT('Ctrl Pts',(-1.1897638022903,1.16626445202765,10.8835222734383));
#54773=CARTESIAN_POINT('Ctrl Pts',(-1.20294370476452,1.15261665892353,10.8847825210151));
#54774=CARTESIAN_POINT('Ctrl Pts',(-1.20745625485334,1.14788854347665,10.885218681442));
#54775=CARTESIAN_POINT('Ctrl Pts',(-1.21569313043718,1.13915588004169,10.8860237346351));
#54776=CARTESIAN_POINT('Ctrl Pts',(-1.21942570266535,1.13515939814867,10.8863919904103));
#54777=CARTESIAN_POINT('Ctrl Pts',(-1.22793498003955,1.1259580769118,10.8872394232869));
#54778=CARTESIAN_POINT('Ctrl Pts',(-1.23269828697405,1.12074119889272,10.8877195609718));
#54779=CARTESIAN_POINT('Ctrl Pts',(-1.24755617500255,1.10425920613157,10.8892350095249));
#54780=CARTESIAN_POINT('Ctrl Pts',(-1.25753027021177,1.09288717787126,10.8902784689742));
#54781=CARTESIAN_POINT('Ctrl Pts',(-1.33430095697377,1.0029141580135,10.8985069289534));
#54782=CARTESIAN_POINT('Ctrl Pts',(-1.39381639785012,0.918405265247922,
10.9060609482324));
#54783=CARTESIAN_POINT('Ctrl Pts',(-1.49160972963105,0.747918408494714,
10.9203537899979));
#54784=CARTESIAN_POINT('Ctrl Pts',(-1.53117834198928,0.663148153811631,
10.9270752438853));
#54785=CARTESIAN_POINT('Ctrl Pts',(-1.5634312473966,0.575533434879242,10.9335682035678));
#54786=CARTESIAN_POINT('Origin',(0.,0.,11.));
#54787=CARTESIAN_POINT('',(-1.56343130033056,0.575533291084625,11.6327248639491));
#54788=CARTESIAN_POINT('',(-1.56343130602848,0.57553327560628,11.4406228970922));
#54789=CARTESIAN_POINT('',(-1.56343130033213,0.575533291080363,11.));
#54790=CARTESIAN_POINT('Ctrl Pts',(-1.56343130602848,0.575533275606279,
11.4406228970922));
#54791=CARTESIAN_POINT('Ctrl Pts',(-1.52680415602541,0.675030620751227,
11.4331999282501));
#54792=CARTESIAN_POINT('Ctrl Pts',(-1.4807595962946,0.770812720066577,11.4254116886702));
#54793=CARTESIAN_POINT('Ctrl Pts',(-1.38901729314585,0.922647599030889,
11.4125310881713));
#54794=CARTESIAN_POINT('Ctrl Pts',(-1.34822687156867,0.981291912119414,
11.4073994728654));
#54795=CARTESIAN_POINT('Ctrl Pts',(-1.27719545497935,1.07058569585643,11.3993896440164));
#54796=CARTESIAN_POINT('Ctrl Pts',(-1.2493150986331,1.10299334354318,11.3964352948152));
#54797=CARTESIAN_POINT('Ctrl Pts',(-1.21122468512642,1.14396905522107,11.3926339048998));
#54798=CARTESIAN_POINT('Ctrl Pts',(-1.20211745493481,1.15353546939814,11.391741373696));
#54799=CARTESIAN_POINT('Ctrl Pts',(-1.18582658642031,1.17024522982793,11.3901730329286));
#54800=CARTESIAN_POINT('Ctrl Pts',(-1.17868985742044,1.17743314835424,11.3894952427524));
#54801=CARTESIAN_POINT('Ctrl Pts',(-1.16451042910342,1.19145615191932,11.3881664502302));
#54802=CARTESIAN_POINT('Ctrl Pts',(-1.1574720198851,1.19829496854766,11.3875152981215));
#54803=CARTESIAN_POINT('Ctrl Pts',(-1.14115476302766,1.21387158957363,11.3860246559792));
#54804=CARTESIAN_POINT('Ctrl Pts',(-1.13183517777627,1.22256597960806,11.3851870536404));
#54805=CARTESIAN_POINT('Ctrl Pts',(-1.10213430496782,1.24964365104814,11.3825596062455));
#54806=CARTESIAN_POINT('Ctrl Pts',(-1.08139739599307,1.26763129140331,11.3807862410512));
#54807=CARTESIAN_POINT('Ctrl Pts',(-0.958853784418267,1.36873145575102,
11.3706280493842));
#54808=CARTESIAN_POINT('Ctrl Pts',(-0.847946011875471,1.44007515277548,
11.3627263346979));
#54809=CARTESIAN_POINT('Ctrl Pts',(-0.665501442593592,1.52898003752134,
11.3502750842259));
#54810=CARTESIAN_POINT('Ctrl Pts',(-0.599258275396191,1.55613601526051,
11.3458415704982));
#54811=CARTESIAN_POINT('Ctrl Pts',(-0.516521726540974,1.58398565171396,
11.3401777510343));
#54812=CARTESIAN_POINT('Ctrl Pts',(-0.50148916581896,1.58880892840692,11.3391436631441));
#54813=CARTESIAN_POINT('Ctrl Pts',(-0.479518412867594,1.59551550459381,
11.3376219259028));
#54814=CARTESIAN_POINT('Ctrl Pts',(-0.472632468861314,1.59756883366874,
11.3371435213696));
#54815=CARTESIAN_POINT('Ctrl Pts',(-0.460521283147991,1.6010951312682,11.3362991599318));
#54816=CARTESIAN_POINT('Ctrl Pts',(-0.455301801929291,1.60258720183891,
11.335934307079));
#54817=CARTESIAN_POINT('Ctrl Pts',(-0.443887692550371,1.6057898408727,11.335134243773));
#54818=CARTESIAN_POINT('Ctrl Pts',(-0.437690527287485,1.60749006077306,
11.3346984844407));
#54819=CARTESIAN_POINT('Ctrl Pts',(-0.420295981326831,1.61215429016526,
11.3334718260548));
#54820=CARTESIAN_POINT('Ctrl Pts',(-0.409077553698217,1.6150373690936,11.3326766031399));
#54821=CARTESIAN_POINT('Ctrl Pts',(-0.328053294678667,1.63496186459302,
11.3269081042534));
#54822=CARTESIAN_POINT('Ctrl Pts',(-0.257246741716699,1.64758642932576,
11.3217365917514));
#54823=CARTESIAN_POINT('Ctrl Pts',(-0.172315049178187,1.65712074998418,
11.3155308954068));
#54824=CARTESIAN_POINT('Ctrl Pts',(-0.158756465695755,1.65847461139677,
11.3145400165099));
#54825=CARTESIAN_POINT('Ctrl Pts',(-0.0783239098896369,1.66551064060783,
11.3086647877825));
#54826=CARTESIAN_POINT('Ctrl Pts',(-0.0111693775689137,1.66731412506099,
11.3037747107781));
#54827=CARTESIAN_POINT('Ctrl Pts',(0.104740214183322,1.66342185065338,11.2954579894606));
#54828=CARTESIAN_POINT('Ctrl Pts',(0.15347488822052,1.65963518838055,11.291998283413));
#54829=CARTESIAN_POINT('Ctrl Pts',(0.234998124708908,1.64967832418225,11.2862845732992));
#54830=CARTESIAN_POINT('Ctrl Pts',(0.267893389389845,1.64465683265151,11.2839991919595));
#54831=CARTESIAN_POINT('Ctrl Pts',(0.314054636464036,1.63618834343614,11.280818718306));
#54832=CARTESIAN_POINT('Ctrl Pts',(0.32746043685702,1.63355816899194,11.2798982259755));
#54833=CARTESIAN_POINT('Ctrl Pts',(0.350546970495702,1.62873303832968,11.2783180740732));
#54834=CARTESIAN_POINT('Ctrl Pts',(0.360243057067358,1.62661594601923,11.2776559754844));
#54835=CARTESIAN_POINT('Ctrl Pts',(0.380042310638634,1.62210715441826,11.2763069139866));
#54836=CARTESIAN_POINT('Ctrl Pts',(0.390143211155946,1.6197073999143,11.2756202410596));
#54837=CARTESIAN_POINT('Ctrl Pts',(0.415739907847208,1.61337283609254,11.2738837381741));
#54838=CARTESIAN_POINT('Ctrl Pts',(0.431202937373876,1.60930905518004,11.2728380835525));
#54839=CARTESIAN_POINT('Ctrl Pts',(0.492367500966336,1.59228971733899,11.26871259214));
#54840=CARTESIAN_POINT('Ctrl Pts',(0.537566744035031,1.57760417506351,11.2656884909209));
#54841=CARTESIAN_POINT('Ctrl Pts',(0.68687195542736,1.52193008346564,11.2556951671206));
#54842=CARTESIAN_POINT('Ctrl Pts',(0.787460706370518,1.47240289906889,11.2489744714618));
#54843=CARTESIAN_POINT('Ctrl Pts',(0.937267060222162,1.37886949937426,11.2381071702515));
#54844=CARTESIAN_POINT('Ctrl Pts',(0.990151535062417,1.34139804771574,11.2340714925394));
#54845=CARTESIAN_POINT('Ctrl Pts',(1.05249865954227,1.2915224685893,11.2288847237947));
#54846=CARTESIAN_POINT('Ctrl Pts',(1.06415322615937,1.28193665497802,11.2278953388318));
#54847=CARTESIAN_POINT('Ctrl Pts',(1.08106472997162,1.26763751041616,11.2264275365377));
#54848=CARTESIAN_POINT('Ctrl Pts',(1.08642485530412,1.26304664896806,11.2259574683638));
#54849=CARTESIAN_POINT('Ctrl Pts',(1.09549250344564,1.25517992763709,11.2251536484357));
#54850=CARTESIAN_POINT('Ctrl Pts',(1.09921486510716,1.25192138542609,11.2248211614527));
#54851=CARTESIAN_POINT('Ctrl Pts',(1.10765885666109,1.24446285149135,11.2240611132963));
#54852=CARTESIAN_POINT('Ctrl Pts',(1.11237103269848,1.24025264110613,11.2236328109873));
#54853=CARTESIAN_POINT('Ctrl Pts',(1.1252979248929,1.22856986028904,11.2224466113756));
#54854=CARTESIAN_POINT('Ctrl Pts',(1.13346187702411,1.22104196411171,11.2216848158298));
#54855=CARTESIAN_POINT('Ctrl Pts',(1.18017906181246,1.17709229775537,11.2172549094665));
#54856=CARTESIAN_POINT('Ctrl Pts',(1.21704721143242,1.13893099589742,11.213478201823));
#54857=CARTESIAN_POINT('Ctrl Pts',(1.31907103785556,1.0227095699659,11.2023247677993));
#54858=CARTESIAN_POINT('Ctrl Pts',(1.37898936413965,0.940358125328246,11.1948565532927));
#54859=CARTESIAN_POINT('Ctrl Pts',(1.46813511871479,0.790813959349761,11.1823788814111));
#54860=CARTESIAN_POINT('Ctrl Pts',(1.50114435264857,0.726206357437456,11.1772874817726));
#54861=CARTESIAN_POINT('Ctrl Pts',(1.53680945967183,0.643492134973699,11.1711405835001));
#54862=CARTESIAN_POINT('Ctrl Pts',(1.54351848247649,0.62722896821404,11.1699487783287));
#54863=CARTESIAN_POINT('Ctrl Pts',(1.5539008833093,0.60088521559031,11.1680444115883));
#54864=CARTESIAN_POINT('Ctrl Pts',(1.55773652977485,0.590870468520734,11.1673264528803));
#54865=CARTESIAN_POINT('Ctrl Pts',(1.56488764334266,0.571645402353845,11.1659593763906));
#54866=CARTESIAN_POINT('Ctrl Pts',(1.56821914585558,0.562441570180001,11.1653097477712));
#54867=CARTESIAN_POINT('Ctrl Pts',(1.57564248484131,0.54135450266583,11.16383212123));
#54868=CARTESIAN_POINT('Ctrl Pts',(1.57968139197608,0.529453163017561,11.163005898946));
#54869=CARTESIAN_POINT('Ctrl Pts',(1.59011160202665,0.497536438770089,11.1608099012462));
#54870=CARTESIAN_POINT('Ctrl Pts',(1.59625973198114,0.477443552781406,11.1594480297858));
#54871=CARTESIAN_POINT('Ctrl Pts',(1.63514025446537,0.341218029154579,11.1503405848552));
#54872=CARTESIAN_POINT('Ctrl Pts',(1.65555405592692,0.221941455764129,11.1430117065387));
#54873=CARTESIAN_POINT('Ctrl Pts',(1.66694887180154,0.0352486599636227,
11.1315828566084));
#54874=CARTESIAN_POINT('Ctrl Pts',(1.66702963059881,-0.0311760937028539,
11.1275165565406));
#54875=CARTESIAN_POINT('Ctrl Pts',(1.66183494844437,-0.119856516986022,
11.1218944039437));
#54876=CARTESIAN_POINT('Ctrl Pts',(1.66006717219818,-0.142259845034495,
11.1204572759337));
#54877=CARTESIAN_POINT('Ctrl Pts',(1.65626496397208,-0.180551071752954,
11.1179617660694));
#54878=CARTESIAN_POINT('Ctrl Pts',(1.65445349808572,-0.196458384572196,
11.1169134076195));
#54879=CARTESIAN_POINT('Ctrl Pts',(1.65149220758552,-0.219503305305378,
11.115374491118));
#54880=CARTESIAN_POINT('Ctrl Pts',(1.65052465809985,-0.226663982444802,
11.1148934729786));
#54881=CARTESIAN_POINT('Ctrl Pts',(1.6487481033183,-0.239197004915987,11.1140462375138));
#54882=CARTESIAN_POINT('Ctrl Pts',(1.64795935499907,-0.244572031157596,
11.1136811506669));
#54883=CARTESIAN_POINT('Ctrl Pts',(1.64618422338066,-0.256270279034346,
11.1128826977338));
#54884=CARTESIAN_POINT('Ctrl Pts',(1.64518770943096,-0.262591604046556,
11.1124488021662));
#54885=CARTESIAN_POINT('Ctrl Pts',(1.64230460115243,-0.280219550505908,
11.1112322993519));
#54886=CARTESIAN_POINT('Ctrl Pts',(1.64033773656282,-0.291512420487836,
11.1104454769018));
#54887=CARTESIAN_POINT('Ctrl Pts',(1.62636357641658,-0.367121615552409,
11.1051310347302));
#54888=CARTESIAN_POINT('Ctrl Pts',(1.61069410804004,-0.43069634982824,11.1004386024904));
#54889=CARTESIAN_POINT('Ctrl Pts',(1.58462123779733,-0.51482538160596,11.094054689002));
#54890=CARTESIAN_POINT('Ctrl Pts',(1.57747126718797,-0.53633387036908,11.0924065178323));
#54891=CARTESIAN_POINT('Ctrl Pts',(1.54587439361479,-0.625278431057768,
11.0855367599596));
#54892=CARTESIAN_POINT('Ctrl Pts',(1.51752269974111,-0.691250150453006,
11.0803147437912));
#54893=CARTESIAN_POINT('Ctrl Pts',(1.46474236767866,-0.795037127142525,
11.0719943756124));
#54894=CARTESIAN_POINT('Ctrl Pts',(1.44288248100356,-0.8340533333331,11.0688394967384));
#54895=CARTESIAN_POINT('Ctrl Pts',(1.40313300937471,-0.89874835459799,11.0635682236071));
#54896=CARTESIAN_POINT('Ctrl Pts',(1.38604262743308,-0.924887511315888,
11.06142648367));
#54897=CARTESIAN_POINT('Ctrl Pts',(1.36061799401955,-0.961484536254143,
11.0584086580134));
#54898=CARTESIAN_POINT('Ctrl Pts',(1.35287796822737,-0.972345134275289,
11.0575105529012));
#54899=CARTESIAN_POINT('Ctrl Pts',(1.339183964611,-0.991080078548571,11.055956459253));
#54900=CARTESIAN_POINT('Ctrl Pts',(1.33328895953985,-0.998996481851152,
11.0552982464258));
#54901=CARTESIAN_POINT('Ctrl Pts',(1.32098328685084,-1.01521880652963,11.0539460078468));
#54902=CARTESIAN_POINT('Ctrl Pts',(1.31456379924634,-1.0235175110837,11.0532523668282));
#54903=CARTESIAN_POINT('Ctrl Pts',(1.29784442106834,-1.0447144521434,11.0514753121389));
#54904=CARTESIAN_POINT('Ctrl Pts',(1.2874303147992,-1.05752146278332,11.0503964804088));
#54905=CARTESIAN_POINT('Ctrl Pts',(1.24321814543559,-1.1102712127916,11.0459279575913));
#54906=CARTESIAN_POINT('Ctrl Pts',(1.20773655484132,-1.14876749734315,11.0426070753747));
#54907=CARTESIAN_POINT('Ctrl Pts',(1.09386779429036,-1.26119224913727,11.0326086012846));
#54908=CARTESIAN_POINT('Ctrl Pts',(1.01008361065357,-1.3292418322361,11.0261356558024));
#54909=CARTESIAN_POINT('Ctrl Pts',(0.867580219550214,-1.42367948567678,
11.0156081026858));
#54910=CARTESIAN_POINT('Ctrl Pts',(0.812900167325927,-1.45559275937939,
11.0116611147194));
#54911=CARTESIAN_POINT('Ctrl Pts',(0.743244896754736,-1.49109552685628,
11.0065806783263));
#54912=CARTESIAN_POINT('Ctrl Pts',(0.729854854169249,-1.49769512942274,
11.0056017023295));
#54913=CARTESIAN_POINT('Ctrl Pts',(0.710034204065723,-1.50713529911211,
11.0041464851551));
#54914=CARTESIAN_POINT('Ctrl Pts',(0.703670979873864,-1.51011672674677,
11.003678390824));
#54915=CARTESIAN_POINT('Ctrl Pts',(0.692799317502628,-1.51512690769399,
11.0028767758379));
#54916=CARTESIAN_POINT('Ctrl Pts',(0.688300404963809,-1.5171759925429,11.0025445006919));
#54917=CARTESIAN_POINT('Ctrl Pts',(0.678011511069755,-1.52180701106143,
11.0017832673895));
#54918=CARTESIAN_POINT('Ctrl Pts',(0.672216000650368,-1.52437588316461,
11.001353553614));
#54919=CARTESIAN_POINT('Ctrl Pts',(0.656145715460671,-1.53138960695786,
11.0001597305562));
#54920=CARTESIAN_POINT('Ctrl Pts',(0.645840806281897,-1.53576396760066,
10.9993916443118));
#54921=CARTESIAN_POINT('Ctrl Pts',(0.584467237533515,-1.56108968797728,
10.9948052768274));
#54922=CARTESIAN_POINT('Ctrl Pts',(0.532431721699831,-1.57959429665994,
10.9908694265627));
#54923=CARTESIAN_POINT('Ctrl Pts',(0.385388106416058,-1.62379362779525,
10.9797842684263));
#54924=CARTESIAN_POINT('Ctrl Pts',(0.2888673992686,-1.64371135266555,10.9725614598439));
#54925=CARTESIAN_POINT('Ctrl Pts',(0.118326635277756,-1.66340894264715,
10.9602519194087));
#54926=CARTESIAN_POINT('Ctrl Pts',(0.0450160413489503,-1.66700532130982,
10.955099061244));
#54927=CARTESIAN_POINT('Ctrl Pts',(-0.0459412770266675,-1.66545987923935,
10.9488906209917));
#54928=CARTESIAN_POINT('Ctrl Pts',(-0.0635745736514136,-1.66488003334527,
10.9476953464629));
#54929=CARTESIAN_POINT('Ctrl Pts',(-0.0919176337360897,-1.66349703247122,
10.9457868073769));
#54930=CARTESIAN_POINT('Ctrl Pts',(-0.102634232230457,-1.66287024512904,
10.9450681030364));
#54931=CARTESIAN_POINT('Ctrl Pts',(-0.123106500576227,-1.66147420513064,
10.9437004635255));
#54932=CARTESIAN_POINT('Ctrl Pts',(-0.132862874972388,-1.6607224958501,
10.9430510094189));
#54933=CARTESIAN_POINT('Ctrl Pts',(-0.155112072106176,-1.65881091274185,
10.9415749459233));
#54934=CARTESIAN_POINT('Ctrl Pts',(-0.167599648248697,-1.65759578045169,
10.9407500986715));
#54935=CARTESIAN_POINT('Ctrl Pts',(-0.200883931849875,-1.65397698815559,
10.9385603568907));
#54936=CARTESIAN_POINT('Ctrl Pts',(-0.221651471651399,-1.65132217302296,
10.9372032934373));
#54937=CARTESIAN_POINT('Ctrl Pts',(-0.363010652843222,-1.63053657821236,
10.9280168293121));
#54938=CARTESIAN_POINT('Ctrl Pts',(-0.481346589209406,-1.5996048221466,
10.9206146187411));
#54939=CARTESIAN_POINT('Ctrl Pts',(-0.656446875116323,-1.5326205730266,
10.9091574593696));
#54940=CARTESIAN_POINT('Ctrl Pts',(-0.716199669293584,-1.5056244932141,
10.9051411926259));
#54941=CARTESIAN_POINT('Ctrl Pts',(-0.793954798611089,-1.46481717569995,
10.8995820077205));
#54942=CARTESIAN_POINT('Ctrl Pts',(-0.813495263033446,-1.45405603007515,
10.8981550969396));
#54943=CARTESIAN_POINT('Ctrl Pts',(-0.846602371653801,-1.4349473589184,
10.8956756371163));
#54944=CARTESIAN_POINT('Ctrl Pts',(-0.860276528287626,-1.42679141711541,
10.8946329405356));
#54945=CARTESIAN_POINT('Ctrl Pts',(-0.879969658466467,-1.41465945845793,
10.8931008377304));
#54946=CARTESIAN_POINT('Ctrl Pts',(-0.88608348358604,-1.41083806248265,
10.8926208538071));
#54947=CARTESIAN_POINT('Ctrl Pts',(-0.896800415679471,-1.40404239541337,
10.8917714699259));
#54948=CARTESIAN_POINT('Ctrl Pts',(-0.901413938743539,-1.40108491656536,
10.8914031630923));
#54949=CARTESIAN_POINT('Ctrl Pts',(-0.911409599276173,-1.39460743482798,
10.8905993039523));
#54950=CARTESIAN_POINT('Ctrl Pts',(-0.916785892387817,-1.39107906998691,
10.8901632291134));
#54951=CARTESIAN_POINT('Ctrl Pts',(-0.931805368220433,-1.3810971708628,
10.8889348485243));
#54952=CARTESIAN_POINT('Ctrl Pts',(-0.941401531734948,-1.37457403469348,
10.8881382003642));
#54953=CARTESIAN_POINT('Ctrl Pts',(-1.01411976068916,-1.32402411731741,
10.8820151980566));
#54954=CARTESIAN_POINT('Ctrl Pts',(-1.07418446962033,-1.27577576066867,
10.8764617505525));
#54955=CARTESIAN_POINT('Ctrl Pts',(-1.17271831573672,-1.18472027527041,
10.866709789005));
#54956=CARTESIAN_POINT('Ctrl Pts',(-1.2127160994911,-1.14374398593016,10.8625340679763));
#54957=CARTESIAN_POINT('Ctrl Pts',(-1.30523270470012,-1.03864271114068,
10.8524157577727));
#54958=CARTESIAN_POINT('Ctrl Pts',(-1.35523646339031,-0.972496182516221,
10.8465359739544));
#54959=CARTESIAN_POINT('Ctrl Pts',(-1.41249751619161,-0.883701534918635,
10.8392722112035));
#54960=CARTESIAN_POINT('Ctrl Pts',(-1.42447989055803,-0.864253878928096,
10.8377163294764));
#54961=CARTESIAN_POINT('Ctrl Pts',(-1.44205075479366,-0.834377201235911,
10.8353774208782));
#54962=CARTESIAN_POINT('Ctrl Pts',(-1.44793394389673,-0.824125597186695,
10.8345838058823));
#54963=CARTESIAN_POINT('Ctrl Pts',(-1.45798593633717,-0.806169781612048,
10.8332089484065));
#54964=CARTESIAN_POINT('Ctrl Pts',(-1.46220393856249,-0.798493803620333,
10.8326259613752));
#54965=CARTESIAN_POINT('Ctrl Pts',(-1.47157871329896,-0.781110051626613,
10.8313161574842));
#54966=CARTESIAN_POINT('Ctrl Pts',(-1.47670037024429,-0.771383723224131,
10.8305906055266));
#54967=CARTESIAN_POINT('Ctrl Pts',(-1.49033970080047,-0.744848071586037,
10.8286302887352));
#54968=CARTESIAN_POINT('Ctrl Pts',(-1.49866922321161,-0.727943459207529,
10.827402110806));
#54969=CARTESIAN_POINT('Ctrl Pts',(-1.55032747202257,-0.618456952377694,
10.8195712382604));
#54970=CARTESIAN_POINT('Ctrl Pts',(-1.58534697505317,-0.522190676368287,
10.8132658863826));
#54971=CARTESIAN_POINT('Ctrl Pts',(-1.63137840859933,-0.346972750260619,
10.802190147954));
#54972=CARTESIAN_POINT('Ctrl Pts',(-1.64598176929133,-0.26931079204428,
10.7974061195732));
#54973=CARTESIAN_POINT('Ctrl Pts',(-1.65850626943725,-0.160734821567394,
10.7905689514215));
#54974=CARTESIAN_POINT('Ctrl Pts',(-1.66116101457131,-0.130470663733504,
10.7886468331598));
#54975=CARTESIAN_POINT('Ctrl Pts',(-1.66418791587085,-0.0802104585073211,
10.7854031531401));
#54976=CARTESIAN_POINT('Ctrl Pts',(-1.66503005317733,-0.0602492566000276,
10.7841014471221));
#54977=CARTESIAN_POINT('Ctrl Pts',(-1.66570362216151,-0.032397461746249,
10.782260418426));
#54978=CARTESIAN_POINT('Ctrl Pts',(-1.66583827534872,-0.0245150283787174,
10.7817366178689));
#54979=CARTESIAN_POINT('Ctrl Pts',(-1.6659726109324,-0.0110596327767957,
10.7808373124782));
#54980=CARTESIAN_POINT('Ctrl Pts',(-1.66600028457275,-0.00548696565446436,
10.7804633385582));
#54981=CARTESIAN_POINT('Ctrl Pts',(-1.66599968502267,0.00616352312797371,
10.779678150415));
#54982=CARTESIAN_POINT('Ctrl Pts',(-1.66596611339039,0.0122411424855048,
10.7792666713526));
#54983=CARTESIAN_POINT('Ctrl Pts',(-1.66578610194907,0.0286116915225238,
10.7781535096789));
#54984=CARTESIAN_POINT('Ctrl Pts',(-1.66557751929742,0.0389034723344217,
10.7774485682847));
#54985=CARTESIAN_POINT('Ctrl Pts',(-1.6639886650865,0.0926898451027791,
10.7737399160954));
#54986=CARTESIAN_POINT('Ctrl Pts',(-1.66100009117117,0.136116355026789,
10.7706620761982));
#54987=CARTESIAN_POINT('Ctrl Pts',(-1.6441454412181,0.291751984701615,10.7594389432007));
#54988=CARTESIAN_POINT('Ctrl Pts',(-1.62056971782624,0.402603097172142,
10.7511066252568));
#54989=CARTESIAN_POINT('Ctrl Pts',(-1.57889401068256,0.532146948207532,
10.741354356213));
#54990=CARTESIAN_POINT('Ctrl Pts',(-1.57138636178916,0.553923432122347,
10.7397133445268));
#54991=CARTESIAN_POINT('Ctrl Pts',(-1.56343131785294,0.575533243485219,
10.7380842620731));
#54992=CARTESIAN_POINT('Ctrl Pts',(-1.5634312473966,0.575533434879242,10.9335682035678));
#54993=CARTESIAN_POINT('Ctrl Pts',(-1.57071877584423,0.555736931321281,
10.9350352846818));
#54994=CARTESIAN_POINT('Ctrl Pts',(-1.57763279198976,0.535795252065528,
10.9364913948363));
#54995=CARTESIAN_POINT('Ctrl Pts',(-1.59014703553624,0.497354401049535,
10.9392573276825));
#54996=CARTESIAN_POINT('Ctrl Pts',(-1.59580591892224,0.478886749103904,
10.9405683569805));
#54997=CARTESIAN_POINT('Ctrl Pts',(-1.60420744729071,0.449663767309595,
10.9426159013899));
#54998=CARTESIAN_POINT('Ctrl Pts',(-1.60716580672233,0.438972798223727,
10.9433593532419));
#54999=CARTESIAN_POINT('Ctrl Pts',(-1.61251548064756,0.418860691160464,
10.9447477043977));
#55000=CARTESIAN_POINT('Ctrl Pts',(-1.61493153853463,0.409446683484319,
10.9453933779506));
#55001=CARTESIAN_POINT('Ctrl Pts',(-1.62018074961505,0.388223899812921,
10.9468398600334));
#55002=CARTESIAN_POINT('Ctrl Pts',(-1.6229674694414,0.37640412321985,10.947639148739));
#55003=CARTESIAN_POINT('Ctrl Pts',(-1.63080912829016,0.341436542247001,
10.949986006012));
#55004=CARTESIAN_POINT('Ctrl Pts',(-1.63549994704836,0.318209583739206,
10.9515220012339));
#55005=CARTESIAN_POINT('Ctrl Pts',(-1.65728489821288,0.197077252263585,
10.9594276681495));
#55006=CARTESIAN_POINT('Ctrl Pts',(-1.66608966735504,0.0978828953325324,
10.9655325939493));
#55007=CARTESIAN_POINT('Ctrl Pts',(-1.6658981856851,-0.112759820905185,
10.9784007705868));
#55008=CARTESIAN_POINT('Ctrl Pts',(-1.65465493934185,-0.223699563860263,
10.9851260456819));
#55009=CARTESIAN_POINT('Ctrl Pts',(-1.62953788689807,-0.346950391322927,
10.9933054270432));
#55010=CARTESIAN_POINT('Ctrl Pts',(-1.62644134714192,-0.36118805044362,
10.9942614427947));
#55011=CARTESIAN_POINT('Ctrl Pts',(-1.62159043659175,-0.382163438860362,
10.995688878288));
#55012=CARTESIAN_POINT('Ctrl Pts',(-1.61997982909137,-0.388934168013582,
10.9961525892672));
#55013=CARTESIAN_POINT('Ctrl Pts',(-1.61702944769712,-0.401000754908375,
10.9969845888326));
#55014=CARTESIAN_POINT('Ctrl Pts',(-1.61570598591677,-0.406300388195197,
10.9973519506303));
#55015=CARTESIAN_POINT('Ctrl Pts',(-1.61272094838418,-0.418008334236784,
10.9981678971318));
#55016=CARTESIAN_POINT('Ctrl Pts',(-1.61104725109372,-0.424413213506575,
10.9986171386645));
#55017=CARTESIAN_POINT('Ctrl Pts',(-1.60601331846817,-0.443218086920089,
10.9999442460219));
#55018=CARTESIAN_POINT('Ctrl Pts',(-1.60254785861527,-0.455589055315543,
11.0008277165885));
#55019=CARTESIAN_POINT('Ctrl Pts',(-1.59421373107115,-0.484067895332003,
11.0028837454387));
#55020=CARTESIAN_POINT('Ctrl Pts',(-1.58924344028509,-0.500144366576006,
11.0040609407974));
#55021=CARTESIAN_POINT('Ctrl Pts',(-1.57122404753477,-0.555445555352912,
11.0081616190516));
#55022=CARTESIAN_POINT('Ctrl Pts',(-1.55695977481508,-0.594256337775516,
11.0111291398076));
#55023=CARTESIAN_POINT('Ctrl Pts',(-1.49354422057804,-0.748788072819416,
11.0232153221401));
#55024=CARTESIAN_POINT('Ctrl Pts',(-1.43280319360239,-0.859325543723636,
11.0324490374598));
#55025=CARTESIAN_POINT('Ctrl Pts',(-1.33452346236187,-0.998288870543778,
11.0444224162866));
#55026=CARTESIAN_POINT('Ctrl Pts',(-1.30740062046708,-1.03355589882088,
11.0475023441914));
#55027=CARTESIAN_POINT('Ctrl Pts',(-1.26886397986868,-1.07971536313839,
11.0515926877636));
#55028=CARTESIAN_POINT('Ctrl Pts',(-1.25866220333435,-1.0915908353244,11.0526506948859));
#55029=CARTESIAN_POINT('Ctrl Pts',(-1.24146474006488,-1.11104799449976,
11.0543942439288));
#55030=CARTESIAN_POINT('Ctrl Pts',(-1.23456350768248,-1.11871144655892,
11.0550836343344));
#55031=CARTESIAN_POINT('Ctrl Pts',(-1.22085370597447,-1.13365407152389,
11.0564333893415));
#55032=CARTESIAN_POINT('Ctrl Pts',(-1.21405010425275,-1.14093719239031,
11.0570939227923));
#55033=CARTESIAN_POINT('Ctrl Pts',(-1.19760444729514,-1.15822825780232,
11.0586688508361));
#55034=CARTESIAN_POINT('Ctrl Pts',(-1.18790162510323,-1.16817757971492,
11.0595805813252));
#55035=CARTESIAN_POINT('Ctrl Pts',(-1.15345733722443,-1.20262393233005,
11.062758266647));
#55036=CARTESIAN_POINT('Ctrl Pts',(-1.12807253976171,-1.22646678244395,
11.0649958171087));
#55037=CARTESIAN_POINT('Ctrl Pts',(-1.0628586638089,-1.28398022448151,11.0705144053655));
#55038=CARTESIAN_POINT('Ctrl Pts',(-1.0221608785796,-1.31660985373681,11.073757275999));
#55039=CARTESIAN_POINT('Ctrl Pts',(-0.90025344298711,-1.40528410075077,
11.0830397046707));
#55040=CARTESIAN_POINT('Ctrl Pts',(-0.815521375226819,-1.45609167489788,
11.0889683104914));
#55041=CARTESIAN_POINT('Ctrl Pts',(-0.681969091694501,-1.52084061545234,
11.0982131396581));
#55042=CARTESIAN_POINT('Ctrl Pts',(-0.636192135361141,-1.5405507331665,
11.1013683615726));
#55043=CARTESIAN_POINT('Ctrl Pts',(-0.57940544221888,-1.56203850371185,
11.1053461791347));
#55044=CARTESIAN_POINT('Ctrl Pts',(-0.569167394054663,-1.56579801238063,
11.1060658148755));
#55045=CARTESIAN_POINT('Ctrl Pts',(-0.552982626069039,-1.57156151149899,
11.1072084448144));
#55046=CARTESIAN_POINT('Ctrl Pts',(-0.547060020292501,-1.57363296232603,
11.1076276218111));
#55047=CARTESIAN_POINT('Ctrl Pts',(-0.535914766197649,-1.57746052977105,
11.1084186492292));
#55048=CARTESIAN_POINT('Ctrl Pts',(-0.530694935239136,-1.57922425315533,
11.1087900536916));
#55049=CARTESIAN_POINT('Ctrl Pts',(-0.518379805478667,-1.58331744985111,
11.1096684103215));
#55050=CARTESIAN_POINT('Ctrl Pts',(-0.511277489692944,-1.58562514262265,
11.1101765919751));
#55051=CARTESIAN_POINT('Ctrl Pts',(-0.487580399527958,-1.59314906723114,
11.1118769844955));
#55052=CARTESIAN_POINT('Ctrl Pts',(-0.470920097836824,-1.59815293336517,
11.113080297446));
#55053=CARTESIAN_POINT('Ctrl Pts',(-0.430015462363119,-1.6097433922762,
11.1160487814468));
#55054=CARTESIAN_POINT('Ctrl Pts',(-0.405695028750299,-1.61604408804506,
11.1178256814515));
#55055=CARTESIAN_POINT('Ctrl Pts',(-0.301944554148621,-1.64043323263404,
11.1254318220529));
#55056=CARTESIAN_POINT('Ctrl Pts',(-0.221388769564987,-1.65323256412621,
11.1313952444484));
#55057=CARTESIAN_POINT('Ctrl Pts',(-0.0407492538871145,-1.66849066695665,
11.1445633330364));
#55058=CARTESIAN_POINT('Ctrl Pts',(0.0592922748583388,-1.66793644952417,
11.1517110401823));
#55059=CARTESIAN_POINT('Ctrl Pts',(0.182254356801667,-1.65617010868027,
11.1602152398388));
#55060=CARTESIAN_POINT('Ctrl Pts',(0.205763018494868,-1.65341397097984,
11.1618292834324));
#55061=CARTESIAN_POINT('Ctrl Pts',(0.241228459531508,-1.6484878395009,11.1642474711962));
#55062=CARTESIAN_POINT('Ctrl Pts',(0.253232517701558,-1.64668656160653,
11.1650630469841));
#55063=CARTESIAN_POINT('Ctrl Pts',(0.274810473112354,-1.64320712308749,
11.1665241585472));
#55064=CARTESIAN_POINT('Ctrl Pts',(0.284391296317817,-1.64157608503067,
11.1671711490236));
#55065=CARTESIAN_POINT('Ctrl Pts',(0.304879335289231,-1.6379034498421,11.1685511781591));
#55066=CARTESIAN_POINT('Ctrl Pts',(0.315781578301719,-1.63583652145177,
11.1692833812133));
#55067=CARTESIAN_POINT('Ctrl Pts',(0.345617973157832,-1.6298705131317,11.1712818744192));
#55068=CARTESIAN_POINT('Ctrl Pts',(0.364506565942917,-1.62575049955715,
11.172541123597));
#55069=CARTESIAN_POINT('Ctrl Pts',(0.406406977212751,-1.61584410742754,
11.1753241779941));
#55070=CARTESIAN_POINT('Ctrl Pts',(0.429375700771275,-1.60989297847586,
11.176842746633));
#55071=CARTESIAN_POINT('Ctrl Pts',(0.502462289296101,-1.58928089204364,
11.1816621023883));
#55072=CARTESIAN_POINT('Ctrl Pts',(0.552022549693937,-1.57275358056102,
11.1849097421345));
#55073=CARTESIAN_POINT('Ctrl Pts',(0.691895420096322,-1.51868049015584,
11.1941433219231));
#55074=CARTESIAN_POINT('Ctrl Pts',(0.779780028180677,-1.4754834137176,11.2000214587095));
#55075=CARTESIAN_POINT('Ctrl Pts',(0.906552665573704,-1.39866649981039,
11.2092497060903));
#55076=CARTESIAN_POINT('Ctrl Pts',(0.948521502198097,-1.37055157187994,
11.2124459724652));
#55077=CARTESIAN_POINT('Ctrl Pts',(0.997946899462727,-1.33408307474949,
11.2164698057187));
#55078=CARTESIAN_POINT('Ctrl Pts',(1.00668480134007,-1.32750192451012,11.2171915453012));
#55079=CARTESIAN_POINT('Ctrl Pts',(1.0203373446209,-1.3170068962905,11.2183367861368));
#55080=CARTESIAN_POINT('Ctrl Pts',(1.02529591862805,-1.313150310399,11.2187564414388));
#55081=CARTESIAN_POINT('Ctrl Pts',(1.03456122504432,-1.30585964486613,11.219547824224));
#55082=CARTESIAN_POINT('Ctrl Pts',(1.03887288149714,-1.30243213757523,11.219919100151));
#55083=CARTESIAN_POINT('Ctrl Pts',(1.04897971470817,-1.29431569884276,11.2207964074553));
#55084=CARTESIAN_POINT('Ctrl Pts',(1.05476050034396,-1.28960918565829,11.2213036594433));
#55085=CARTESIAN_POINT('Ctrl Pts',(1.07386438920556,-1.27384109603936,11.2229976776673));
#55086=CARTESIAN_POINT('Ctrl Pts',(1.08704609586862,-1.26261102130514,11.2241954365437));
#55087=CARTESIAN_POINT('Ctrl Pts',(1.11880073826701,-1.23469198631321,11.2271473499815));
#55088=CARTESIAN_POINT('Ctrl Pts',(1.13717781067257,-1.2177872909621,11.2289130752273));
#55089=CARTESIAN_POINT('Ctrl Pts',(1.2131757470624,-1.14465776625704,11.2364386001796));
#55090=CARTESIAN_POINT('Ctrl Pts',(1.26706010841115,-1.08470947627988,11.2423302485443));
#55091=CARTESIAN_POINT('Ctrl Pts',(1.37838783151862,-0.941186696358283,
11.2555272860077));
#55092=CARTESIAN_POINT('Ctrl Pts',(1.43298033683817,-0.855779733771383,
11.2627725523329));
#55093=CARTESIAN_POINT('Ctrl Pts',(1.49034833877706,-0.744966654909961,
11.2713628015766));
#55094=CARTESIAN_POINT('Ctrl Pts',(1.50075693265496,-0.723769449465426,
11.2729730255757));
#55095=CARTESIAN_POINT('Ctrl Pts',(1.5158242279257,-0.691360949786361,11.2753866800049));
#55096=CARTESIAN_POINT('Ctrl Pts',(1.52081647000792,-0.680308996631328,
11.2762014781242));
#55097=CARTESIAN_POINT('Ctrl Pts',(1.52959102711326,-0.660304261570677,
11.2776617473107));
#55098=CARTESIAN_POINT('Ctrl Pts',(1.53341647787516,-0.651371123339749,
11.2783086659074));
#55099=CARTESIAN_POINT('Ctrl Pts',(1.54144519839993,-0.632159785037457,
11.2796891279832));
#55100=CARTESIAN_POINT('Ctrl Pts',(1.54562433043445,-0.621871958442806,
11.2804218304875));
#55101=CARTESIAN_POINT('Ctrl Pts',(1.5568096386581,-0.593527460832807,11.2824232052748));
#55102=CARTESIAN_POINT('Ctrl Pts',(1.56360443582741,-0.575388839656622,
11.2836848017333));
#55103=CARTESIAN_POINT('Ctrl Pts',(1.60842018115751,-0.449092070961539,
11.292346721424));
#55104=CARTESIAN_POINT('Ctrl Pts',(1.63550625635248,-0.33737647683352,11.2993644250222));
#55105=CARTESIAN_POINT('Ctrl Pts',(1.66472655707294,-0.121781079564549,
11.312649761082));
#55106=CARTESIAN_POINT('Ctrl Pts',(1.66906779960012,-0.0187623355534116,
11.3189020300812));
#55107=CARTESIAN_POINT('Ctrl Pts',(1.66311812060077,0.0991145056551233,
11.3265685230733));
#55108=CARTESIAN_POINT('Ctrl Pts',(1.66214797711956,0.11423498116346,11.3275618398591));
#55109=CARTESIAN_POINT('Ctrl Pts',(1.6604229850146,0.136387255304573,11.3290344080363));
#55110=CARTESIAN_POINT('Ctrl Pts',(1.65982933562618,0.143431323765842,11.329505233388));
#55111=CARTESIAN_POINT('Ctrl Pts',(1.65869693862962,0.155917847918266,11.3303447371709));
#55112=CARTESIAN_POINT('Ctrl Pts',(1.65817619663891,0.161361732980802,11.3307124159305));
#55113=CARTESIAN_POINT('Ctrl Pts',(1.65697461111951,0.173302655689231,11.3315226458025));
#55114=CARTESIAN_POINT('Ctrl Pts',(1.65628236613275,0.179798198959596,11.331965791999));
#55115=CARTESIAN_POINT('Ctrl Pts',(1.6541631150953,0.198631964565432,11.3332573408261));
#55116=CARTESIAN_POINT('Ctrl Pts',(1.6526363438578,0.21095819672448,11.3341109191133));
#55117=CARTESIAN_POINT('Ctrl Pts',(1.64881347569599,0.239226967968099,11.3360858372393));
#55118=CARTESIAN_POINT('Ctrl Pts',(1.6464237279742,0.255155414175295,11.3372113436737));
#55119=CARTESIAN_POINT('Ctrl Pts',(1.63751661099934,0.309174098002841,11.3410662245656));
#55120=CARTESIAN_POINT('Ctrl Pts',(1.62990540172425,0.347069556616587,11.3438346452289));
#55121=CARTESIAN_POINT('Ctrl Pts',(1.60463244465315,0.453570587915134,11.3517418972522));
#55122=CARTESIAN_POINT('Ctrl Pts',(1.5839036070138,0.521364535189539,11.35692389511));
#55123=CARTESIAN_POINT('Ctrl Pts',(1.52475986563298,0.678265952061657,11.3690698922512));
#55124=CARTESIAN_POINT('Ctrl Pts',(1.48275295180678,0.765758997451002,11.3759576152573));
#55125=CARTESIAN_POINT('Ctrl Pts',(1.42379957556579,0.865276549473997,11.3838679462899));
#55126=CARTESIAN_POINT('Ctrl Pts',(1.41395432555655,0.881272916746876,11.3851425681699));
#55127=CARTESIAN_POINT('Ctrl Pts',(1.39787156684631,0.906440262667726,11.3871537340142));
#55128=CARTESIAN_POINT('Ctrl Pts',(1.39180962183681,0.915720947683956,11.3878966549857));
#55129=CARTESIAN_POINT('Ctrl Pts',(1.38031054826023,0.932947732230548,11.389278353703));
#55130=CARTESIAN_POINT('Ctrl Pts',(1.37489632535546,0.940908487520375,11.3899179512588));
#55131=CARTESIAN_POINT('Ctrl Pts',(1.36251735466579,0.958774775370628,11.3913561455047));
#55132=CARTESIAN_POINT('Ctrl Pts',(1.35551296069141,0.968652279186948,11.3921531969008));
#55133=CARTESIAN_POINT('Ctrl Pts',(1.33412278702271,0.998129981138125,11.3945385577487));
#55134=CARTESIAN_POINT('Ctrl Pts',(1.31941466489741,1.01749305158815,11.3961144338449));
#55135=CARTESIAN_POINT('Ctrl Pts',(1.28442739687989,1.06151834328147,11.3997251588363));
#55136=CARTESIAN_POINT('Ctrl Pts',(1.26385248940985,1.08593370088755,11.401748501344));
#55137=CARTESIAN_POINT('Ctrl Pts',(1.1856571824124,1.17348951001685,11.40911405457));
#55138=CARTESIAN_POINT('Ctrl Pts',(1.12390482189085,1.23276098760362,11.4143122881039));
#55139=CARTESIAN_POINT('Ctrl Pts',(0.987582775935279,1.34481045468046,11.4250927673246));
#55140=CARTESIAN_POINT('Ctrl Pts',(0.912685219320327,1.3967234262007,11.4306618544543));
#55141=CARTESIAN_POINT('Ctrl Pts',(0.820368580384159,1.45010242268945,11.4375818878878));
#55142=CARTESIAN_POINT('Ctrl Pts',(0.806690992839717,1.45775554965117,11.4386086515978));
#55143=CARTESIAN_POINT('Ctrl Pts',(0.786673382212309,1.46858818079766,11.4401165416515));
#55144=CARTESIAN_POINT('Ctrl Pts',(0.780417345423651,1.47192221855082,11.4405885228168));
#55145=CARTESIAN_POINT('Ctrl Pts',(0.76928740144223,1.47776281273496,11.4414298366642));
#55146=CARTESIAN_POINT('Ctrl Pts',(0.76442212667314,1.48028539399641,11.4417981623177));
#55147=CARTESIAN_POINT('Ctrl Pts',(0.753820348580666,1.48571607101186,11.4426020757118));
#55148=CARTESIAN_POINT('Ctrl Pts',(0.748079513365872,1.4886149266299,11.4430381861598));
#55149=CARTESIAN_POINT('Ctrl Pts',(0.731636610028338,1.49679869589307,11.4442892483032));
#55150=CARTESIAN_POINT('Ctrl Pts',(0.720894593532401,1.50200180750442,11.4451089064427));
#55151=CARTESIAN_POINT('Ctrl Pts',(0.624045348150771,1.54763445491757,11.4525138410255));
#55152=CARTESIAN_POINT('Ctrl Pts',(0.534687206007513,1.5807310934726,11.4594410883713));
#55153=CARTESIAN_POINT('Ctrl Pts',(0.326512974647072,1.6381539008925,11.4751607674641));
#55154=CARTESIAN_POINT('Ctrl Pts',(0.206849823337168,1.65752290284946,11.4838859404648));
#55155=CARTESIAN_POINT('Ctrl Pts',(0.0651569315275816,1.66485780232014,
11.4936460555163));
#55156=CARTESIAN_POINT('Ctrl Pts',(0.0441672989285181,1.66554683123939,
11.4950784885497));
#55157=CARTESIAN_POINT('Ctrl Pts',(0.0106062076012587,1.66601361714739,
11.4973483518401));
#55158=CARTESIAN_POINT('Ctrl Pts',(-0.00195884137095795,1.66604623048518,
11.4981935912387));
#55159=CARTESIAN_POINT('Ctrl Pts',(-0.0243108864459776,1.66585136903568,
11.4996893838935));
#55160=CARTESIAN_POINT('Ctrl Pts',(-0.0340976438810582,1.66567978934368,
11.5003416483516));
#55161=CARTESIAN_POINT('Ctrl Pts',(-0.0546048516140105,1.66513944123438,
11.5017030657081));
#55162=CARTESIAN_POINT('Ctrl Pts',(-0.0653244269441687,1.66475336818898,
11.5024116483862));
#55163=CARTESIAN_POINT('Ctrl Pts',(-0.0936217981824038,1.66346046930715,
11.5042745453528));
#55164=CARTESIAN_POINT('Ctrl Pts',(-0.111190540708841,1.6623785598202,11.5054233744802));
#55165=CARTESIAN_POINT('Ctrl Pts',(-0.201138235611418,1.65540704628226,
11.5112702134185));
#55166=CARTESIAN_POINT('Ctrl Pts',(-0.273097733343431,1.64506796748348,
11.5158271660273));
#55167=CARTESIAN_POINT('Ctrl Pts',(-0.444126025430088,1.60895826451098,
11.5266198914193));
#55168=CARTESIAN_POINT('Ctrl Pts',(-0.541933500201491,1.57870240203124,
11.5327552591224));
#55169=CARTESIAN_POINT('Ctrl Pts',(-0.684813868886588,1.51964993687359,
11.5423662780989));
#55170=CARTESIAN_POINT('Ctrl Pts',(-0.732300099447912,1.49734476944057,
11.5456805477235));
#55171=CARTESIAN_POINT('Ctrl Pts',(-0.788416693140658,1.46767747089229,
11.549837798198));
#55172=CARTESIAN_POINT('Ctrl Pts',(-0.798131138591723,1.46241741992534,
11.5505665234232));
#55173=CARTESIAN_POINT('Ctrl Pts',(-0.813307631085186,1.45400359921348,
11.5517204319693));
#55174=CARTESIAN_POINT('Ctrl Pts',(-0.818805509009888,1.45091464409118,
11.5521416732198));
#55175=CARTESIAN_POINT('Ctrl Pts',(-0.829067608600657,1.44507203294153,
11.552934253373));
#55176=CARTESIAN_POINT('Ctrl Pts',(-0.833835885294892,1.44232589691537,
11.5533051222678));
#55177=CARTESIAN_POINT('Ctrl Pts',(-0.844994237058272,1.4358257779647,11.5541790364662));
#55178=CARTESIAN_POINT('Ctrl Pts',(-0.851372954624263,1.4320527267639,11.5546832735889));
#55179=CARTESIAN_POINT('Ctrl Pts',(-0.872354061618967,1.41945254937007,
11.5563567410385));
#55180=CARTESIAN_POINT('Ctrl Pts',(-0.886845471993696,1.41044397309229,
11.5575366149008));
#55181=CARTESIAN_POINT('Ctrl Pts',(-0.921780841104532,1.38797519309314,
11.5604353497723));
#55182=CARTESIAN_POINT('Ctrl Pts',(-0.94207110789277,1.37428416131279,11.562165280873));
#55183=CARTESIAN_POINT('Ctrl Pts',(-1.02533432213211,1.31539111972873,11.5694379275501));
#55184=CARTESIAN_POINT('Ctrl Pts',(-1.08541377692279,1.26627023946867,11.5751052154449));
#55185=CARTESIAN_POINT('Ctrl Pts',(-1.21836055489277,1.14113652902151,11.5883788451767));
#55186=CARTESIAN_POINT('Ctrl Pts',(-1.28789587849737,1.06203864965379,11.5959174714854));
#55187=CARTESIAN_POINT('Ctrl Pts',(-1.36334154165655,0.957815814520947,
11.6047744259544));
#55188=CARTESIAN_POINT('Ctrl Pts',(-1.37675335546527,0.938435714612838,
11.6063814095401));
#55189=CARTESIAN_POINT('Ctrl Pts',(-1.39643244525766,0.908668942095237,
11.6087912171587));
#55190=CARTESIAN_POINT('Ctrl Pts',(-1.40300445911742,0.898488353653019,
11.6096053547727));
#55191=CARTESIAN_POINT('Ctrl Pts',(-1.4146454606119,0.880016269312702,11.6110649091812));
#55192=CARTESIAN_POINT('Ctrl Pts',(-1.41975402547408,0.87175049612799,11.6117117674137));
#55193=CARTESIAN_POINT('Ctrl Pts',(-1.43054829926958,0.853938525447834,
11.613092600602));
#55194=CARTESIAN_POINT('Ctrl Pts',(-1.43621144110945,0.84437914959494,11.6138257299991));
#55195=CARTESIAN_POINT('Ctrl Pts',(-1.45149864506568,0.817975550740554,
11.6158295684961));
#55196=CARTESIAN_POINT('Ctrl Pts',(-1.46092499291914,0.801018435680312,
11.6170931719142));
#55197=CARTESIAN_POINT('Ctrl Pts',(-1.48126649693276,0.762871863691643,
11.6198873021926));
#55198=CARTESIAN_POINT('Ctrl Pts',(-1.49202755603811,0.741604862674909,
11.6214125266085));
#55199=CARTESIAN_POINT('Ctrl Pts',(-1.52495553742761,0.67290921345574,11.6262464397793));
#55200=CARTESIAN_POINT('Ctrl Pts',(-1.54534568696583,0.624662706286318,
11.6295018139068));
#55201=CARTESIAN_POINT('Ctrl Pts',(-1.56343130033056,0.575533291084625,
11.6327248639491));
#55202=CARTESIAN_POINT('Origin',(0.,0.,11.));
#55203=CARTESIAN_POINT('',(-1.56343130033211,0.57553329108042,12.3306070045052));
#55204=CARTESIAN_POINT('',(-1.56343130033213,0.575533291080364,12.1392916035562));
#55205=CARTESIAN_POINT('',(-1.56343130033213,0.575533291080363,11.));
#55206=CARTESIAN_POINT('',(-1.66599938220149,0.00143474884533201,11.4785196366098));
#55207=CARTESIAN_POINT('Ctrl Pts',(-1.56343130033213,0.575533291080363,
12.1392916035562));
#55208=CARTESIAN_POINT('Ctrl Pts',(-1.54206084724692,0.633585945502796,
12.1351571376634));
#55209=CARTESIAN_POINT('Ctrl Pts',(-1.51747847922349,0.69037758855015,12.1310226717706));
#55210=CARTESIAN_POINT('Ctrl Pts',(-1.48986988536785,0.745549277160123,
12.1268882058779));
#55211=CARTESIAN_POINT('Ctrl Pts',(-1.46220722533534,0.800829009022508,
12.1227456434205));
#55212=CARTESIAN_POINT('Ctrl Pts',(-1.43150675994854,0.854482032851016,
12.1186030809631));
#55213=CARTESIAN_POINT('Ctrl Pts',(-1.3979984684239,0.906176738988833,12.1144605185057));
#55214=CARTESIAN_POINT('Ctrl Pts',(-1.39223108756224,0.91507432956307,12.113747508849));
#55215=CARTESIAN_POINT('Ctrl Pts',(-1.38638062297089,0.923913984412125,
12.1130344991924));
#55216=CARTESIAN_POINT('Ctrl Pts',(-1.38044836581346,0.93269411348145,12.1123214895357));
#55217=CARTESIAN_POINT('Ctrl Pts',(-1.34652463687341,0.98290345382218,12.1082441298256));
#55218=CARTESIAN_POINT('Ctrl Pts',(-1.30978799052863,1.03136324686654,12.1041667701154));
#55219=CARTESIAN_POINT('Ctrl Pts',(-1.27044517463845,1.07774071939306,12.1000894104053));
#55220=CARTESIAN_POINT('Ctrl Pts',(-1.2306824601219,1.12461317014033,12.095968533786));
#55221=CARTESIAN_POINT('Ctrl Pts',(-1.1882578366262,1.16935810112152,12.0918476571668));
#55222=CARTESIAN_POINT('Ctrl Pts',(-1.14343038978819,1.21166123306344,12.0877267805476));
#55223=CARTESIAN_POINT('Ctrl Pts',(-1.09919851005162,1.2534023353684,12.0836606529431));
#55224=CARTESIAN_POINT('Ctrl Pts',(-1.05262764816723,1.29276576409608,12.0795945253385));
#55225=CARTESIAN_POINT('Ctrl Pts',(-1.00400609036898,1.329484024162,12.0755283977339));
#55226=CARTESIAN_POINT('Ctrl Pts',(-0.955414279483092,1.36617981981268,
12.0714647578066));
#55227=CARTESIAN_POINT('Ctrl Pts',(-0.904774667943586,1.40023334757946,
12.0674011178792));
#55228=CARTESIAN_POINT('Ctrl Pts',(-0.852408730657561,1.43141725429686,
12.0633374779519));
#55229=CARTESIAN_POINT('Ctrl Pts',(-0.800055376895427,1.46259366752793,
12.0592748145164));
#55230=CARTESIAN_POINT('Ctrl Pts',(-0.745976960568927,1.49090156677985,
12.0552121510808));
#55231=CARTESIAN_POINT('Ctrl Pts',(-0.690522278667592,1.51615796758244,
12.0511494876453));
#55232=CARTESIAN_POINT('Ctrl Pts',(-0.633692199812496,1.54204078216175,
12.0469860613036));
#55233=CARTESIAN_POINT('Ctrl Pts',(-0.575417161880126,1.56471842482518,
12.0428226349618));
#55234=CARTESIAN_POINT('Ctrl Pts',(-0.516095133905195,1.58404602608617,
12.03865920862));
#55235=CARTESIAN_POINT('Ctrl Pts',(-0.458134905445043,1.60292994194196,
12.0345913581068));
#55236=CARTESIAN_POINT('Ctrl Pts',(-0.399175774768682,1.61861593101746,
12.0305235075935));
#55237=CARTESIAN_POINT('Ctrl Pts',(-0.339602531693703,1.63101996323381,
12.0264556570802));
#55238=CARTESIAN_POINT('Ctrl Pts',(-0.277929741679332,1.64386115224291,
12.0222444428242));
#55239=CARTESIAN_POINT('Ctrl Pts',(-0.215599329682191,1.65318459814998,
12.0180332285682));
#55240=CARTESIAN_POINT('Ctrl Pts',(-0.153044687118163,1.65895549179142,
12.0138220143122));
#55241=CARTESIAN_POINT('Ctrl Pts',(-0.0904900445541309,1.66472638543285,
12.0096108000562));
#55242=CARTESIAN_POINT('Ctrl Pts',(-0.0277117742953075,1.66694477799572,
12.0053995858002));
#55243=CARTESIAN_POINT('Ctrl Pts',(0.0348591494664867,1.66563526610674,
12.0011883715442));
#55244=CARTESIAN_POINT('Ctrl Pts',(0.0954412400614033,1.66436737739544,
11.997111011834));
#55245=CARTESIAN_POINT('Ctrl Pts',(0.156079149144275,1.65978734370476,11.9930336521239));
#55246=CARTESIAN_POINT('Ctrl Pts',(0.216381166954204,1.65188837110367,11.9889562924138));
#55247=CARTESIAN_POINT('Ctrl Pts',(0.277326777091683,1.64390509422312,11.9848354157945));
#55248=CARTESIAN_POINT('Ctrl Pts',(0.337928754544622,1.63253153470738,11.9807145391753));
#55249=CARTESIAN_POINT('Ctrl Pts',(0.397782539949318,1.6178149000771,11.9765936625561));
#55250=CARTESIAN_POINT('Ctrl Pts',(0.456841121790149,1.60329378725428,11.9725275349516));
#55251=CARTESIAN_POINT('Ctrl Pts',(0.515170759296967,1.58551801480475,11.968461407347));
#55252=CARTESIAN_POINT('Ctrl Pts',(0.572390360221283,1.56458469745992,11.9643952797424));
#55253=CARTESIAN_POINT('Ctrl Pts',(0.629574953907417,1.5436641872234,11.9603316398151));
#55254=CARTESIAN_POINT('Ctrl Pts',(0.685650377718311,1.51959013782031,11.9562679998877));
#55255=CARTESIAN_POINT('Ctrl Pts',(0.740251263076272,1.49250931907107,11.9522043599604));
#55256=CARTESIAN_POINT('Ctrl Pts',(0.794839027852877,1.46543500783692,11.9481416965249));
#55257=CARTESIAN_POINT('Ctrl Pts',(0.847952499137718,1.43535558895083,11.9440790330893));
#55258=CARTESIAN_POINT('Ctrl Pts',(0.899248765001825,1.40246485112558,11.9400163696538));
#55259=CARTESIAN_POINT('Ctrl Pts',(0.951817290040193,1.36875835132932,11.935852943312));
#55260=CARTESIAN_POINT('Ctrl Pts',(1.00247676149926,1.3320994714463,11.9316895169703));
#55261=CARTESIAN_POINT('Ctrl Pts',(1.05088961915896,1.29274398406798,11.9275260906285));
#55262=CARTESIAN_POINT('Ctrl Pts',(1.09819110877679,1.25429194327509,11.9234582401153));
#55263=CARTESIAN_POINT('Ctrl Pts',(1.14334769923026,1.21326619913791,11.919390389602));
#55264=CARTESIAN_POINT('Ctrl Pts',(1.18608009164613,1.16994445004911,11.9153225390887));
#55265=CARTESIAN_POINT('Ctrl Pts',(1.23031850688496,1.12509590736954,11.9111113248327));
#55266=CARTESIAN_POINT('Ctrl Pts',(1.27195823100646,1.07778692007959,11.9069001105767));
#55267=CARTESIAN_POINT('Ctrl Pts',(1.31073495670596,1.02836271483802,11.9026888963207));
#55268=CARTESIAN_POINT('Ctrl Pts',(1.34951168240545,0.978938509596461,11.8984776820647));
#55269=CARTESIAN_POINT('Ctrl Pts',(1.38542512570093,0.927399620658939,11.8942664678087));
#55270=CARTESIAN_POINT('Ctrl Pts',(1.41826219911196,0.874121464425921,11.8900552535526));
#55271=CARTESIAN_POINT('Ctrl Pts',(1.45005553756154,0.822536768314798,11.8859778938425));
#55272=CARTESIAN_POINT('Ctrl Pts',(1.47909650830513,0.769108734991152,11.8819005341324));
#55273=CARTESIAN_POINT('Ctrl Pts',(1.50516694787099,0.714162767887491,11.8778231744222));
#55274=CARTESIAN_POINT('Ctrl Pts',(1.53151563243573,0.658630372598905,11.873702297803));
#55275=CARTESIAN_POINT('Ctrl Pts',(1.55482964881038,0.601547851913972,11.8695814211838));
#55276=CARTESIAN_POINT('Ctrl Pts',(1.57492923255732,0.5432806939662,11.8654605445646));
#55277=CARTESIAN_POINT('Ctrl Pts',(1.59476177787856,0.485787660016459,11.86139441696));
#55278=CARTESIAN_POINT('Ctrl Pts',(1.61146461092941,0.427141772983075,11.8573282893554));
#55279=CARTESIAN_POINT('Ctrl Pts',(1.62491262407231,0.367715874188799,11.8532621617509));
#55280=CARTESIAN_POINT('Ctrl Pts',(1.63835240965349,0.308326332456741,11.8491985218235));
#55281=CARTESIAN_POINT('Ctrl Pts',(1.64854121075687,0.248158223442775,11.8451348818961));
#55282=CARTESIAN_POINT('Ctrl Pts',(1.65540416483726,0.18759811043677,11.8410712419688));
#55283=CARTESIAN_POINT('Ctrl Pts',(1.66226546975121,0.127052550013376,11.8370085785333));
#55284=CARTESIAN_POINT('Ctrl Pts',(1.66580245654855,0.0661156810681977,
11.8329459150977));
#55285=CARTESIAN_POINT('Ctrl Pts',(1.66599194485515,0.00518070243959675,
11.8288832516622));
#55286=CARTESIAN_POINT('Ctrl Pts',(1.66618613288467,-0.0572655964437612,
11.8247198253205));
#55287=CARTESIAN_POINT('Ctrl Pts',(1.66286449565371,-0.11970934912481,11.8205563989787));
#55288=CARTESIAN_POINT('Ctrl Pts',(1.65605883015649,-0.18172823407689,11.8163929726369));
#55289=CARTESIAN_POINT('Ctrl Pts',(1.64940939586525,-0.242323410327245,
11.8123251221237));
#55290=CARTESIAN_POINT('Ctrl Pts',(1.6394343571667,-0.302512511885207,11.8082572716104));
#55291=CARTESIAN_POINT('Ctrl Pts',(1.62621553145385,-0.361910272385679,
11.8041894210971));
#55292=CARTESIAN_POINT('Ctrl Pts',(1.6125308330835,-0.423401395272077,11.7999782068411));
#55293=CARTESIAN_POINT('Ctrl Pts',(1.5953695548898,-0.484043768527647,11.7957669925851));
#55294=CARTESIAN_POINT('Ctrl Pts',(1.57487837812754,-0.543428094697315,
11.7915557783291));
#55295=CARTESIAN_POINT('Ctrl Pts',(1.55438720136529,-0.602812420866984,
11.7873445640731));
#55296=CARTESIAN_POINT('Ctrl Pts',(1.53056642085407,-0.660938171598326,
11.7831333498171));
#55297=CARTESIAN_POINT('Ctrl Pts',(1.50361586187397,-0.717422706583087,
11.7789221355611));
#55298=CARTESIAN_POINT('Ctrl Pts',(1.47752193345548,-0.772111865859231,
11.7748447758509));
#55299=CARTESIAN_POINT('Ctrl Pts',(1.44838652639371,-0.825488459811084,
11.7707674161408));
#55300=CARTESIAN_POINT('Ctrl Pts',(1.41636469530226,-0.87719270967179,11.7666900564306));
#55301=CARTESIAN_POINT('Ctrl Pts',(1.3840011011065,-0.929448789466517,11.7625691798114));
#55302=CARTESIAN_POINT('Ctrl Pts',(1.34868925098605,-0.979996101643676,
11.7584483031922));
#55303=CARTESIAN_POINT('Ctrl Pts',(1.31063870291815,-1.02848538658215,11.754327426573));
#55304=CARTESIAN_POINT('Ctrl Pts',(1.27309368564042,-1.07633045408422,11.7502612989684));
#55305=CARTESIAN_POINT('Ctrl Pts',(1.23288262401006,-1.12217143160885,11.7461951713639));
#55306=CARTESIAN_POINT('Ctrl Pts',(1.19025089843454,-1.16570099029544,11.7421290437593));
#55307=CARTESIAN_POINT('Ctrl Pts',(1.14764525516199,-1.20920391738027,11.7380654038319));
#55308=CARTESIAN_POINT('Ctrl Pts',(1.10262224176067,-1.25039786444183,11.7340017639046));
#55309=CARTESIAN_POINT('Ctrl Pts',(1.0554660188658,-1.28901027265867,11.7299381239772));
#55310=CARTESIAN_POINT('Ctrl Pts',(1.00832112760153,-1.32761340232181,11.7258754605417));
#55311=CARTESIAN_POINT('Ctrl Pts',(0.959044440380017,-1.36363590041568,
11.7218127971062));
#55312=CARTESIAN_POINT('Ctrl Pts',(0.907953723972735,-1.39684502902936,
11.7177501336707));
#55313=CARTESIAN_POINT('Ctrl Pts',(0.855595846465663,-1.4308778163994,11.7135867073289));
#55314=CARTESIAN_POINT('Ctrl Pts',(0.801333193676861,-1.46195546166263,
11.7094232809872));
#55315=CARTESIAN_POINT('Ctrl Pts',(0.745537817954203,-1.48987561964081,
11.7052598546454));
#55316=CARTESIAN_POINT('Ctrl Pts',(0.691023283736475,-1.51715484104137,
11.7011920041321));
#55317=CARTESIAN_POINT('Ctrl Pts',(0.635046163916582,-1.54141986525428,
11.6971241536189));
#55318=CARTESIAN_POINT('Ctrl Pts',(0.577974509655393,-1.56253046888328,
11.6930563031056));
#55319=CARTESIAN_POINT('Ctrl Pts',(0.518891472248906,-1.58438507604392,
11.6888450888496));
#55320=CARTESIAN_POINT('Ctrl Pts',(0.458635869004211,-1.6028585484011,11.6846338745936));
#55321=CARTESIAN_POINT('Ctrl Pts',(0.397631121277882,-1.61785212284414,
11.6804226603376));
#55322=CARTESIAN_POINT('Ctrl Pts',(0.336626373551552,-1.63284569728718,
11.6762114460816));
#55323=CARTESIAN_POINT('Ctrl Pts',(0.274873085134287,-1.64435933493581,
11.6720002318256));
#55324=CARTESIAN_POINT('Ctrl Pts',(0.212801106105302,-1.65235337904468,
11.6677890175695));
#55325=CARTESIAN_POINT('Ctrl Pts',(0.152702101154361,-1.66009333037203,
11.6637116578594));
#55326=CARTESIAN_POINT('Ctrl Pts',(0.0920561875886168,-1.66456612528513,
11.6596342981493));
#55327=CARTESIAN_POINT('Ctrl Pts',(0.0312497260217383,-1.66570689337097,
11.6555569384391));
#55328=CARTESIAN_POINT('Ctrl Pts',(-0.0302057117079062,-1.66685983666444,
11.6514360618199));
#55329=CARTESIAN_POINT('Ctrl Pts',(-0.0918246332323487,-1.66460905070646,
11.6473151852007));
#55330=CARTESIAN_POINT('Ctrl Pts',(-0.15319995386838,-1.65894116054028,
11.6431943085815));
#55331=CARTESIAN_POINT('Ctrl Pts',(-0.213759856175037,-1.6533485726533,
11.6391281809769));
#55332=CARTESIAN_POINT('Ctrl Pts',(-0.274082066190559,-1.64442917375535,
11.6350620533723));
#55333=CARTESIAN_POINT('Ctrl Pts',(-0.33377529726945,-1.63222242691757,
11.6309959257678));
#55334=CARTESIAN_POINT('Ctrl Pts',(-0.393432007730964,-1.62002314822857,
11.6269322858404));
#55335=CARTESIAN_POINT('Ctrl Pts',(-0.452460001683601,-1.60454061160897,
11.622868645913));
#55336=CARTESIAN_POINT('Ctrl Pts',(-0.510476170309535,-1.58586571926696,
11.6188050059857));
#55337=CARTESIAN_POINT('Ctrl Pts',(-0.568478397662058,-1.56719531449774,
11.6147423425502));
#55338=CARTESIAN_POINT('Ctrl Pts',(-0.625468795245726,-1.54533423365308,
11.6106796791146));
#55339=CARTESIAN_POINT('Ctrl Pts',(-0.681079481799879,-1.52042321064604,
11.6066170156791));
#55340=CARTESIAN_POINT('Ctrl Pts',(-0.738069434563094,-1.49489433998425,
11.6024535893373));
#55341=CARTESIAN_POINT('Ctrl Pts',(-0.793609787320232,-1.46616239368055,
11.5982901629956));
#55342=CARTESIAN_POINT('Ctrl Pts',(-0.847328749322365,-1.43443019717649,
11.5941267366538));
#55343=CARTESIAN_POINT('Ctrl Pts',(-0.899814536079456,-1.40342644660179,
11.5900588861406));
#55344=CARTESIAN_POINT('Ctrl Pts',(-0.950561273723657,-1.36955908824795,
11.5859910356273));
#55345=CARTESIAN_POINT('Ctrl Pts',(-0.999251532235019,-1.33306127965895,
11.581923185114));
#55346=CARTESIAN_POINT('Ctrl Pts',(-1.04965778735748,-1.29527717443144,
11.577711970858));
#55347=CARTESIAN_POINT('Ctrl Pts',(-1.09785941592614,-1.25467409688016,
11.573500756602));
#55348=CARTESIAN_POINT('Ctrl Pts',(-1.14354378837388,-1.21155421012496,
11.569289542346));
#55349=CARTESIAN_POINT('Ctrl Pts',(-1.18922816082161,-1.16843432336977,
11.56507832809));
#55350=CARTESIAN_POINT('Ctrl Pts',(-1.23239491699965,-1.1227981135873,11.560867113834));
#55351=CARTESIAN_POINT('Ctrl Pts',(-1.27277759774085,-1.07498520300934,
11.5566558995779));
#55352=CARTESIAN_POINT('Ctrl Pts',(-1.3116212125385,-1.02899453951805,11.5526051832464));
#55353=CARTESIAN_POINT('Ctrl Pts',(-1.34805528098541,-0.980793330512334,
11.5485544669148));
#55354=CARTESIAN_POINT('Ctrl Pts',(-1.38181662139976,-0.930665796525989,
11.5445037505832));
#55355=CARTESIAN_POINT('Ctrl Pts',(-1.41552828728624,-0.880612017359611,
11.5404589942467));
#55356=CARTESIAN_POINT('Ctrl Pts',(-1.44657472963222,-0.828637955103961,
11.5364142379102));
#55357=CARTESIAN_POINT('Ctrl Pts',(-1.47473247479964,-0.775061370325818,
11.5323694815737));
#55358=CARTESIAN_POINT('Ctrl Pts',(-1.50285958738946,-0.721543071070213,
11.528329125494));
#55359=CARTESIAN_POINT('Ctrl Pts',(-1.52810399251593,-0.666426162304626,
11.5242887694144));
#55360=CARTESIAN_POINT('Ctrl Pts',(-1.55028629329074,-0.610056070238507,
11.5202484133348));
#55361=CARTESIAN_POINT('Ctrl Pts',(-1.57245652133952,-0.553716657617442,
11.5162102562205));
#55362=CARTESIAN_POINT('Ctrl Pts',(-1.59156775366362,-0.496125893490407,
11.5121720991063));
#55363=CARTESIAN_POINT('Ctrl Pts',(-1.60748808713347,-0.437650602334751,
11.5081339419921));
#55364=CARTESIAN_POINT('Ctrl Pts',(-1.62340334069714,-0.379193969644614,
11.5040970733847));
#55365=CARTESIAN_POINT('Ctrl Pts',(-1.63612958438953,-0.319853871896392,
11.5000602047774));
#55366=CARTESIAN_POINT('Ctrl Pts',(-1.64558501067163,-0.260011485617207,
11.4960233361701));
#55367=CARTESIAN_POINT('Ctrl Pts',(-1.6550445903921,-0.200142812668726,
11.4919846943074));
#55368=CARTESIAN_POINT('Ctrl Pts',(-1.66123040716838,-0.139771924292852,
11.4879460524447));
#55369=CARTESIAN_POINT('Ctrl Pts',(-1.66411221800991,-0.0792876148595837,
11.4839074105821));
#55370=CARTESIAN_POINT('Ctrl Pts',(-1.66539371692077,-0.0523911317368556,
11.4821114859246));
#55371=CARTESIAN_POINT('Ctrl Pts',(-1.66602255436523,-0.0254722673943331,
11.4803155612672));
#55372=CARTESIAN_POINT('Ctrl Pts',(-1.66599938220149,0.00143474884533201,
11.4785196366098));
#55373=CARTESIAN_POINT('Ctrl Pts',(-1.66599941321298,0.00139827537052137,
11.4779266028919));
#55374=CARTESIAN_POINT('Ctrl Pts',(-1.66589455998199,0.126327473850728,
11.4702430512039));
#55375=CARTESIAN_POINT('Ctrl Pts',(-1.65173819877438,0.250838710108895,
11.4627912325929));
#55376=CARTESIAN_POINT('Ctrl Pts',(-1.61997824373514,0.389254288929557,
11.453712034288));
#55377=CARTESIAN_POINT('Ctrl Pts',(-1.61589773461963,0.405860658420447,
11.4526088843924));
#55378=CARTESIAN_POINT('Ctrl Pts',(-1.60826460209374,0.434982944530017,
11.4506450534144));
#55379=CARTESIAN_POINT('Ctrl Pts',(-1.60481956514939,0.44752578699632,11.4497895839921));
#55380=CARTESIAN_POINT('Ctrl Pts',(-1.59939126133126,0.466420247224837,
11.4484844664259));
#55381=CARTESIAN_POINT('Ctrl Pts',(-1.59751613115846,0.472802771476853,
11.4480407437214));
#55382=CARTESIAN_POINT('Ctrl Pts',(-1.59403225077199,0.484403760595211,
11.4472287256181));
#55383=CARTESIAN_POINT('Ctrl Pts',(-1.59243600561464,0.489625760383796,
11.4468611486657));
#55384=CARTESIAN_POINT('Ctrl Pts',(-1.58875835588181,0.501448690897791,
11.4460242538234));
#55385=CARTESIAN_POINT('Ctrl Pts',(-1.58666148509883,0.508044516146688,
11.445554071794));
#55386=CARTESIAN_POINT('Ctrl Pts',(-1.5800847112575,0.528294240404594,11.4441008376607));
#55387=CARTESIAN_POINT('Ctrl Pts',(-1.57546933580326,0.54190297701641,11.4431105279836));
#55388=CARTESIAN_POINT('Ctrl Pts',(-1.56830545224653,0.562160722799511,
11.4416175787372));
#55389=CARTESIAN_POINT('Ctrl Pts',(-1.56588958929984,0.568855369760643,
11.4411211002045));
#55390=CARTESIAN_POINT('Ctrl Pts',(-1.56343130602848,0.57553327560628,11.4406228970922));
#55391=CARTESIAN_POINT('',(-1.66599994488069,0.000428552845177652,11.6700306692265));
#55392=CARTESIAN_POINT('Ctrl Pts',(-1.56343130033056,0.575533291084625,
11.6327248639491));
#55393=CARTESIAN_POINT('Ctrl Pts',(-1.56351122601218,0.575316173648889,
11.6327391075618));
#55394=CARTESIAN_POINT('Ctrl Pts',(-1.56359110668459,0.575099038970977,
11.6327533505678));
#55395=CARTESIAN_POINT('Ctrl Pts',(-1.60363162838075,0.466189362563932,
11.6398964400467));
#55396=CARTESIAN_POINT('Ctrl Pts',(-1.6321469700982,0.353636689900426,11.6468216608511));
#55397=CARTESIAN_POINT('Ctrl Pts',(-1.65364856931402,0.205335811496005,
11.6562926822567));
#55398=CARTESIAN_POINT('Ctrl Pts',(-1.65750085011162,0.171484535364838,
11.6584789615107));
#55399=CARTESIAN_POINT('Ctrl Pts',(-1.66112862429576,0.127692478015936,
11.6613659914878));
#55400=CARTESIAN_POINT('Ctrl Pts',(-1.66185686981429,0.117836360658527,
11.662019590846));
#55401=CARTESIAN_POINT('Ctrl Pts',(-1.66288543893601,0.101999370109436,
11.6630767880648));
#55402=CARTESIAN_POINT('Ctrl Pts',(-1.66324129210249,0.0960221637506752,
11.6634773912633));
#55403=CARTESIAN_POINT('Ctrl Pts',(-1.66384554950732,0.084858406409156,
11.6642288016679));
#55404=CARTESIAN_POINT('Ctrl Pts',(-1.66410193987922,0.079672407006859,
11.6645791617619));
#55405=CARTESIAN_POINT('Ctrl Pts',(-1.66458357073178,0.0689106409105714,
11.6653088109921));
#55406=CARTESIAN_POINT('Ctrl Pts',(-1.6648050480824,0.0633347457529103,
11.6656883000724));
#55407=CARTESIAN_POINT('Ctrl Pts',(-1.66529993332798,0.0490686009949908,
11.6666627492508));
#55408=CARTESIAN_POINT('Ctrl Pts',(-1.66553332743975,0.0403772563584407,
11.6672597434594));
#55409=CARTESIAN_POINT('Ctrl Pts',(-1.66589684342434,0.0212668390744461,
11.6685791600074));
#55410=CARTESIAN_POINT('Ctrl Pts',(-1.6659972647262,0.010847658152853,11.6693029296631));
#55411=CARTESIAN_POINT('Ctrl Pts',(-1.66599994488069,0.000428552845177652,
11.6700306692265));
#55412=CARTESIAN_POINT('Ctrl Pts',(-1.66599994441765,0.000430349150014435,
11.6700305437606));
#55413=CARTESIAN_POINT('Ctrl Pts',(-1.66603398663936,-0.131356455761258,
11.6792354043323));
#55414=CARTESIAN_POINT('Ctrl Pts',(-1.65043138951007,-0.262683581037981,
11.6890002640304));
#55415=CARTESIAN_POINT('Ctrl Pts',(-1.60343336664041,-0.457446627409522,
11.703442600239));
#55416=CARTESIAN_POINT('Ctrl Pts',(-1.58325195220095,-0.52304039504908,
11.7083083319204));
#55417=CARTESIAN_POINT('Ctrl Pts',(-1.54930763632162,-0.613164745409152,
11.7149684577475));
#55418=CARTESIAN_POINT('Ctrl Pts',(-1.53888539439045,-0.638871708300922,
11.7168657543864));
#55419=CARTESIAN_POINT('Ctrl Pts',(-1.52274474471149,-0.675993198741766,
11.7196034780031));
#55420=CARTESIAN_POINT('Ctrl Pts',(-1.5175298762557,-0.687620136864921,
11.7204606929069));
#55421=CARTESIAN_POINT('Ctrl Pts',(-1.50807622133212,-0.708066254024198,
11.7219679805535));
#55422=CARTESIAN_POINT('Ctrl Pts',(-1.50389223403985,-0.716909941936505,
11.722619892978));
#55423=CARTESIAN_POINT('Ctrl Pts',(-1.49495048662678,-0.735387293080214,
11.7239820993412));
#55424=CARTESIAN_POINT('Ctrl Pts',(-1.49017693360736,-0.745012848181586,
11.7246918097402));
#55425=CARTESIAN_POINT('Ctrl Pts',(-1.47730131768552,-0.770356734711056,
11.7265611697142));
#55426=CARTESIAN_POINT('Ctrl Pts',(-1.46904140783254,-0.785993678727426,
11.7277152636192));
#55427=CARTESIAN_POINT('Ctrl Pts',(-1.42861311348497,-0.859664469187664,
11.7331607037792));
#55428=CARTESIAN_POINT('Ctrl Pts',(-1.39324388539401,-0.91587740689338,
11.7373368070795));
#55429=CARTESIAN_POINT('Ctrl Pts',(-1.27035251924036,-1.08752511347798,
11.7504087997539));
#55430=CARTESIAN_POINT('Ctrl Pts',(-1.17112827482285,-1.1937145325723,11.7589556465323));
#55431=CARTESIAN_POINT('Ctrl Pts',(-1.04783918606911,-1.29530515211135,
11.7692150133112));
#55432=CARTESIAN_POINT('Ctrl Pts',(-1.03609839116646,-1.30471548094666,
11.7701893786152));
#55433=CARTESIAN_POINT('Ctrl Pts',(-1.01752458650463,-1.31919371058587,
11.7717296187688));
#55434=CARTESIAN_POINT('Ctrl Pts',(-1.01077719063821,-1.32437071619692,
11.7722889083239));
#55435=CARTESIAN_POINT('Ctrl Pts',(-0.998266884594302,-1.33381808025436,
11.7733260581721));
#55436=CARTESIAN_POINT('Ctrl Pts',(-0.992515424157479,-1.33810334885753,
11.7738029421152));
#55437=CARTESIAN_POINT('Ctrl Pts',(-0.986682520742523,-1.34239100405459,
11.7742868487018));
#55438=CARTESIAN_POINT('Ctrl Pts',(-0.986628435126881,-1.34243075631653,
11.7742913357505));
#55439=CARTESIAN_POINT('Ctrl Pts',(-0.986520182520877,-1.3425103105739,
11.7743003166458));
#55440=CARTESIAN_POINT('Ctrl Pts',(-0.986466015518797,-1.34255011256367,
11.7743048104935));
#55441=CARTESIAN_POINT('Ctrl Pts',(-0.986357584220192,-1.34262977793024,
11.7743138063081));
#55442=CARTESIAN_POINT('Ctrl Pts',(-0.986303319919582,-1.34266964129279,
11.7743183082755));
#55443=CARTESIAN_POINT('Ctrl Pts',(-0.986194677852247,-1.3427494412316,
11.7743273216717));
#55444=CARTESIAN_POINT('Ctrl Pts',(-0.986140300070534,-1.34278937779857,
11.7743318331018));
#55445=CARTESIAN_POINT('Ctrl Pts',(-0.986031414581058,-1.3428693361724,
11.7743408667899));
#55446=CARTESIAN_POINT('Ctrl Pts',(-0.985976906869207,-1.34290935795885,
11.7743453890482));
#55447=CARTESIAN_POINT('Ctrl Pts',(-0.985867744763561,-1.34298949900268,
11.7743544457834));
#55448=CARTESIAN_POINT('Ctrl Pts',(-0.985813090355817,-1.34302961824368,
11.7743589802616));
#55449=CARTESIAN_POINT('Ctrl Pts',(-0.985729207033549,-1.34309118518265,
11.7743659397949));
#55450=CARTESIAN_POINT('Ctrl Pts',(-0.985699979852384,-1.34311263527425,
11.7743683646886));
#55451=CARTESIAN_POINT('Ctrl Pts',(-0.985640794992522,-1.34315606860381,
11.7743732750975));
#55452=CARTESIAN_POINT('Ctrl Pts',(-0.985610837285705,-1.34317805178826,
11.7743757606155));
#55453=CARTESIAN_POINT('Ctrl Pts',(-0.985550154785851,-1.34322257792734,
11.7743807953099));
#55454=CARTESIAN_POINT('Ctrl Pts',(-0.985519429951186,-1.34324512083271,
11.7743833444901));
#55455=CARTESIAN_POINT('Ctrl Pts',(-0.985457174147864,-1.3432907948206,
11.7743885097501));
#55456=CARTESIAN_POINT('Ctrl Pts',(-0.985425643133429,-1.34331392585066,
11.774391125834));
#55457=CARTESIAN_POINT('Ctrl Pts',(-0.985361733237205,-1.34336080644189,
11.7743964283651));
#55458=CARTESIAN_POINT('Ctrl Pts',(-0.985329354312176,-1.34338455594189,
11.7743991148164));
#55459=CARTESIAN_POINT('Ctrl Pts',(-0.985263703952054,-1.34343270593545,
11.7744045617876));
#55460=CARTESIAN_POINT('Ctrl Pts',(-0.985230432458938,-1.34345710637115,
11.7744073223129));
#55461=CARTESIAN_POINT('Ctrl Pts',(-0.985162949113861,-1.3435065930218,
11.7744129214038));
#55462=CARTESIAN_POINT('Ctrl Pts',(-0.985128737227789,-1.34353167915303,
11.7744157599728));
#55463=CARTESIAN_POINT('Ctrl Pts',(-0.985059321787992,-1.34358257448658,
11.7744215194099));
#55464=CARTESIAN_POINT('Ctrl Pts',(-0.985024118168926,-1.34360838361888,
11.774424440284));
#55465=CARTESIAN_POINT('Ctrl Pts',(-0.984952664132694,-1.34366076501403,
11.7744303689075));
#55466=CARTESIAN_POINT('Ctrl Pts',(-0.984916413654861,-1.34368733719323,
11.7744333766625));
#55467=CARTESIAN_POINT('Ctrl Pts',(-0.984842806578718,-1.3437412877765,
11.7744394839719));
#55468=CARTESIAN_POINT('Ctrl Pts',(-0.98480544991269,-1.34376866609077,
11.7744425835325));
#55469=CARTESIAN_POINT('Ctrl Pts',(-0.984729566531095,-1.34382427537263,
11.7744488797597));
#55470=CARTESIAN_POINT('Ctrl Pts',(-0.984691039750174,-1.34385250623609,
11.7744520764325));
#55471=CARTESIAN_POINT('Ctrl Pts',(-0.984612747148914,-1.34390987070635,
11.7744585726106));
#55472=CARTESIAN_POINT('Ctrl Pts',(-0.984572981243418,-1.34393900420947,
11.7744618721238));
#55473=CARTESIAN_POINT('Ctrl Pts',(-0.984492135789026,-1.34399822810989,
11.7744685801758));
#55474=CARTESIAN_POINT('Ctrl Pts',(-0.984451056167939,-1.34402831837829,
11.7744719887214));
#55475=CARTESIAN_POINT('Ctrl Pts',(-0.984367502500312,-1.34408951442711,
11.7744789215439));
#55476=CARTESIAN_POINT('Ctrl Pts',(-0.984325028352428,-1.34412062008237,
11.7744824458302));
#55477=CARTESIAN_POINT('Ctrl Pts',(-0.984238597970242,-1.34418391049498,
11.7744896174109));
#55478=CARTESIAN_POINT('Ctrl Pts',(-0.984194641640596,-1.344216095103,11.7744932647144));
#55479=CARTESIAN_POINT('Ctrl Pts',(-0.984105151607308,-1.34428161252185,
11.7745006902395));
#55480=CARTESIAN_POINT('Ctrl Pts',(-0.984059617783356,-1.34431494517932,
11.7745044684725));
#55481=CARTESIAN_POINT('Ctrl Pts',(-0.983966868962051,-1.3443828339459,
11.7745121644736));
#55482=CARTESIAN_POINT('Ctrl Pts',(-0.983919653840739,-1.34441738987909,
11.7745160822535));
#55483=CARTESIAN_POINT('Ctrl Pts',(-0.98382342912629,-1.34448780730439,
11.7745240667539));
#55484=CARTESIAN_POINT('Ctrl Pts',(-0.983774419385979,-1.34452366860899,
11.7745281334883));
#55485=CARTESIAN_POINT('Ctrl Pts',(-0.983674481481536,-1.3445967865735,
11.774536426188));
#55486=CARTESIAN_POINT('Ctrl Pts',(-0.983623553165258,-1.34463404301702,
11.7745406521678));
#55487=CARTESIAN_POINT('Ctrl Pts',(-0.983519642200692,-1.3447100496814,
11.7745492746414));
#55488=CARTESIAN_POINT('Ctrl Pts',(-0.983466659376021,-1.34474879966651,
11.7745536711518));
#55489=CARTESIAN_POINT('Ctrl Pts',(-0.98335849000438,-1.34482790155846,
11.7745626470892));
#55490=CARTESIAN_POINT('Ctrl Pts',(-0.983303303267584,-1.3448682531969,
11.7745672265342));
#55491=CARTESIAN_POINT('Ctrl Pts',(-0.983190561451798,-1.34495067751751,
11.7745765820081));
#55492=CARTESIAN_POINT('Ctrl Pts',(-0.983133006146599,-1.34499274990903,
11.7745813580582));
#55493=CARTESIAN_POINT('Ctrl Pts',(-0.983015345271399,-1.34507874732413,
11.7745911218464));
#55494=CARTESIAN_POINT('Ctrl Pts',(-0.982955239470018,-1.3451226720045,
11.7745961096065));
#55495=CARTESIAN_POINT('Ctrl Pts',(-0.982832276008239,-1.34521251975161,
11.7746063135525));
#55496=CARTESIAN_POINT('Ctrl Pts',(-0.982769418077261,-1.34525844243851,
11.774611529764));
#55497=CARTESIAN_POINT('Ctrl Pts',(-0.98264072628005,-1.34535244813465,
11.7746222092176));
#55498=CARTESIAN_POINT('Ctrl Pts',(-0.982574892101502,-1.34540053071856,
11.7746276724892));
#55499=CARTESIAN_POINT('Ctrl Pts',(-0.982439997920563,-1.34549903671376,
11.7746388668118));
#55500=CARTESIAN_POINT('Ctrl Pts',(-0.982370937565766,-1.34554945964017,
11.774644597896));
#55501=CARTESIAN_POINT('Ctrl Pts',(-0.982229311403413,-1.34565284820831,
11.7746563510622));
#55502=CARTESIAN_POINT('Ctrl Pts',(-0.982156745193897,-1.34570581329698,
11.7746623731824));
#55503=CARTESIAN_POINT('Ctrl Pts',(-0.98200779326378,-1.34581451281754,
11.7746747344987));
#55504=CARTESIAN_POINT('Ctrl Pts',(-0.981931407084554,-1.34587024661445,
11.7746810737384));
#55505=CARTESIAN_POINT('Ctrl Pts',(-0.981774461103005,-1.34598473894333,
11.7746940986989));
#55506=CARTESIAN_POINT('Ctrl Pts',(-0.981693900772395,-1.34604349674471,
11.7747007844698));
#55507=CARTESIAN_POINT('Ctrl Pts',(-0.981528205529277,-1.34616432609519,
11.7747145357891));
#55508=CARTESIAN_POINT('Ctrl Pts',(-0.981443070009156,-1.34622639679655,
11.7747216013952));
#55509=CARTESIAN_POINT('Ctrl Pts',(-0.981267768335308,-1.34635418047198,
11.7747361502574));
#55510=CARTESIAN_POINT('Ctrl Pts',(-0.981177601469712,-1.34641989246381,
11.7747436335812));
#55511=CARTESIAN_POINT('Ctrl Pts',(-0.980991715854019,-1.34655533397261,
11.7747590611677));
#55512=CARTESIAN_POINT('Ctrl Pts',(-0.980895996271455,-1.34662506234026,
11.7747670055095));
#55513=CARTESIAN_POINT('Ctrl Pts',(-0.980698406307501,-1.34676896747204,
11.7747834048727));
#55514=CARTESIAN_POINT('Ctrl Pts',(-0.980596534945786,-1.34684314288341,
11.7747918599873));
#55515=CARTESIAN_POINT('Ctrl Pts',(-0.980414402392712,-1.34697572711404,
11.7748069768027));
#55516=CARTESIAN_POINT('Ctrl Pts',(-0.980334144381575,-1.34703414032945,
11.7748136382001));
#55517=CARTESIAN_POINT('Ctrl Pts',(-0.975982948706236,-1.35020042349244,
11.7751747900155));
#55518=CARTESIAN_POINT('Ctrl Pts',(-0.971697445285686,-1.35328783766756,
11.7755306943022));
#55519=CARTESIAN_POINT('Ctrl Pts',(-0.961601634330326,-1.36048850606521,
11.7763695572758));
#55520=CARTESIAN_POINT('Ctrl Pts',(-0.955779586134885,-1.36458493922316,
11.7768536194049));
#55521=CARTESIAN_POINT('Ctrl Pts',(-0.936919353971478,-1.37767521879511,
11.7784222346485));
#55522=CARTESIAN_POINT('Ctrl Pts',(-0.923779556000115,-1.38652016595796,
11.7795158694891));
#55523=CARTESIAN_POINT('Ctrl Pts',(-0.842741645057831,-1.4394069235811,
11.7862560411484));
#55524=CARTESIAN_POINT('Ctrl Pts',(-0.771840536400978,-1.4786363415004,
11.7921279719249));
#55525=CARTESIAN_POINT('Ctrl Pts',(-0.635225132019675,-1.5417144908593,
11.8030792897942));
#55526=CARTESIAN_POINT('Ctrl Pts',(-0.570304544354859,-1.5668912770405,
11.8081445063092));
#55527=CARTESIAN_POINT('Ctrl Pts',(-0.437679761108076,-1.60898523820064,
11.8181009063769));
#55528=CARTESIAN_POINT('Ctrl Pts',(-0.370101776274779,-1.62586102088633,
11.8229822940843));
#55529=CARTESIAN_POINT('Ctrl Pts',(-0.284534050029324,-1.64161491607919,
11.828918020116));
#55530=CARTESIAN_POINT('Ctrl Pts',(-0.267361496749432,-1.64449902047222,
11.8300974072706));
#55531=CARTESIAN_POINT('Ctrl Pts',(-0.23958190985519,-1.64871789249165,
11.8319868627773));
#55532=CARTESIAN_POINT('Ctrl Pts',(-0.229002117693853,-1.65022065792549,
11.8327021764599));
#55533=CARTESIAN_POINT('Ctrl Pts',(-0.208693432350862,-1.65290625323593,
11.8340673358782));
#55534=CARTESIAN_POINT('Ctrl Pts',(-0.198967163893991,-1.65410522802625,
11.834717663101));
#55535=CARTESIAN_POINT('Ctrl Pts',(-0.176665255871253,-1.65665486490992,
11.8362011677848));
#55536=CARTESIAN_POINT('Ctrl Pts',(-0.164083580604366,-1.65794829451888,
11.8370325194119));
#55537=CARTESIAN_POINT('Ctrl Pts',(-0.123630244531254,-1.66164198698757,
11.8396886943809));
#55538=CARTESIAN_POINT('Ctrl Pts',(-0.0957115400342689,-1.66348368723332,
11.8414961391643));
#55539=CARTESIAN_POINT('Ctrl Pts',(0.0633884750719321,-1.66995984489162,
11.8516757440964));
#55540=CARTESIAN_POINT('Ctrl Pts',(0.194704438299184,-1.65978210686203,
11.8595674751431));
#55541=CARTESIAN_POINT('Ctrl Pts',(0.393553145097003,-1.62042457267945,
11.8720039669014));
#55542=CARTESIAN_POINT('Ctrl Pts',(0.462662491482679,-1.60206146971411,
11.8764324582381));
#55543=CARTESIAN_POINT('Ctrl Pts',(0.545329691230732,-1.5743000060104,11.8820902736034));
#55544=CARTESIAN_POINT('Ctrl Pts',(0.560215102778949,-1.56906468169421,
11.8831238380227));
#55545=CARTESIAN_POINT('Ctrl Pts',(0.581766137854563,-1.56113925595726,
11.8846449596258));
#55546=CARTESIAN_POINT('Ctrl Pts',(0.588492770549207,-1.55861601105339,
11.8851232828879));
#55547=CARTESIAN_POINT('Ctrl Pts',(0.600273337117831,-1.55410983968561,
11.8859675726368));
#55548=CARTESIAN_POINT('Ctrl Pts',(0.605334214120422,-1.5521455991657,11.8863324360359));
#55549=CARTESIAN_POINT('Ctrl Pts',(0.61636631934651,-1.54780162690558,11.8871326126535));
#55550=CARTESIAN_POINT('Ctrl Pts',(0.622333311754694,-1.5454121008547,11.8875684756355));
#55551=CARTESIAN_POINT('Ctrl Pts',(0.63901938534665,-1.53861773258297,11.8887956389323));
#55552=CARTESIAN_POINT('Ctrl Pts',(0.649706306442231,-1.53413558673956,
11.8895912682762));
#55553=CARTESIAN_POINT('Ctrl Pts',(0.726949311234621,-1.50078767405729,
11.8954079626773));
#55554=CARTESIAN_POINT('Ctrl Pts',(0.791596867669645,-1.46771623997692,
11.9006310499472));
#55555=CARTESIAN_POINT('Ctrl Pts',(0.913746976415361,-1.39480611582528,
11.9109619629968));
#55556=CARTESIAN_POINT('Ctrl Pts',(0.971317722102258,-1.35534501075365,
11.9160563105154));
#55557=CARTESIAN_POINT('Ctrl Pts',(1.09158129590482,-1.26130286230433,11.9270547777676));
#55558=CARTESIAN_POINT('Ctrl Pts',(1.15301718221431,-1.20540026753727,11.9329115406124));
#55559=CARTESIAN_POINT('Ctrl Pts',(1.22250968953689,-1.13196957375865,11.9398166287807));
#55560=CARTESIAN_POINT('Ctrl Pts',(1.23476277469953,-1.11859107466111,11.9410464129022));
#55561=CARTESIAN_POINT('Ctrl Pts',(1.25398643962519,-1.09690088623189,11.9429964631351));
#55562=CARTESIAN_POINT('Ctrl Pts',(1.26109830432541,-1.08871696111644,11.9437226000039));
#55563=CARTESIAN_POINT('Ctrl Pts',(1.27445940930742,-1.07303516457316,11.9450961103957));
#55564=CARTESIAN_POINT('Ctrl Pts',(1.28072360982477,-1.06555069918825,11.9457440817464));
#55565=CARTESIAN_POINT('Ctrl Pts',(1.29489338579194,-1.04831516456348,11.9472193708277));
#55566=CARTESIAN_POINT('Ctrl Pts',(1.30275531252242,-1.03852885124719,11.9480449071877));
#55567=CARTESIAN_POINT('Ctrl Pts',(1.32315312210294,-1.01254203442473,11.9502062449185));
#55568=CARTESIAN_POINT('Ctrl Pts',(1.3355023758078,-0.996197279156565,11.9515347328452));
#55569=CARTESIAN_POINT('Ctrl Pts',(1.42269489460525,-0.876257853132006,
11.9610748167096));
#55570=CARTESIAN_POINT('Ctrl Pts',(1.48569974989495,-0.764584013101859,
11.9688091137676));
#55571=CARTESIAN_POINT('Ctrl Pts',(1.56974477611269,-0.565083332411271,
11.9820499852387));
#55572=CARTESIAN_POINT('Ctrl Pts',(1.59758536104025,-0.480764467601537,
11.9875057890123));
#55573=CARTESIAN_POINT('Ctrl Pts',(1.62147493628602,-0.382784617727158,
11.9940954894124));
#55574=CARTESIAN_POINT('Ctrl Pts',(1.62423620788779,-0.370893181551427,
11.9948994154069));
#55575=CARTESIAN_POINT('Ctrl Pts',(1.62826447606163,-0.352637056289172,
11.9961414951042));
#55576=CARTESIAN_POINT('Ctrl Pts',(1.62962544621324,-0.34629322686093,11.9965745535006));
#55577=CARTESIAN_POINT('Ctrl Pts',(1.63206614071279,-0.334583429377948,
11.9973768559177));
#55578=CARTESIAN_POINT('Ctrl Pts',(1.63315651948792,-0.32921989413831,11.9977454968429));
#55579=CARTESIAN_POINT('Ctrl Pts',(1.635583191509,-0.316974399285635,11.9985897405316));
#55580=CARTESIAN_POINT('Ctrl Pts',(1.63690248873875,-0.310089316252672,
11.9990662646382));
#55581=CARTESIAN_POINT('Ctrl Pts',(1.6409516813258,-0.288211410930166,12.0005858670875));
#55582=CARTESIAN_POINT('Ctrl Pts',(1.64351924256803,-0.273189853823298,
12.0016372798464));
#55583=CARTESIAN_POINT('Ctrl Pts',(1.66170828591985,-0.157216092594068,
12.0098058409452));
#55584=CARTESIAN_POINT('Ctrl Pts',(1.66821939069655,-0.055063232255153,
12.0172841914388));
#55585=CARTESIAN_POINT('Ctrl Pts',(1.66208384983329,0.162184241350495,12.0330906853072));
#55586=CARTESIAN_POINT('Ctrl Pts',(1.64689668242077,0.276707617527558,12.0413522611565));
#55587=CARTESIAN_POINT('Ctrl Pts',(1.61548033641506,0.407621595821442,12.0505645968275));
#55588=CARTESIAN_POINT('Ctrl Pts',(1.61062590548988,0.426399261760057,12.0518811549029));
#55589=CARTESIAN_POINT('Ctrl Pts',(1.60247660913864,0.45579395614083,12.053935322168));
#55590=CARTESIAN_POINT('Ctrl Pts',(1.59940162380001,0.466469580389054,12.054679943252));
#55591=CARTESIAN_POINT('Ctrl Pts',(1.59343729295197,0.486423693598618,12.0560693496815));
#55592=CARTESIAN_POINT('Ctrl Pts',(1.5905731230154,0.495709152068423,12.0567149208678));
#55593=CARTESIAN_POINT('Ctrl Pts',(1.58395458830252,0.516517886652601,12.0581597183115));
#55594=CARTESIAN_POINT('Ctrl Pts',(1.58015537018089,0.528026404720095,12.0589574403438));
#55595=CARTESIAN_POINT('Ctrl Pts',(1.5685970932728,0.561796115284195,12.0612950698144));
#55596=CARTESIAN_POINT('Ctrl Pts',(1.56049054784824,0.583935831772029,12.0628235431184));
#55597=CARTESIAN_POINT('Ctrl Pts',(1.51397534657671,0.703077720301254,12.0710403500499));
#55598=CARTESIAN_POINT('Ctrl Pts',(1.46698891716395,0.796483862879099,12.0774326370651));
#55599=CARTESIAN_POINT('Ctrl Pts',(1.37009380568516,0.951050105963993,12.0885732008225));
#55600=CARTESIAN_POINT('Ctrl Pts',(1.32402180554306,1.01420801253581,12.0933225075936));
#55601=CARTESIAN_POINT('Ctrl Pts',(1.25785695493157,1.09268275665934,12.0997966702496));
#55602=CARTESIAN_POINT('Ctrl Pts',(1.24160586941739,1.11111406418342,12.101363278968));
#55603=CARTESIAN_POINT('Ctrl Pts',(1.21335573224741,1.14176034996381,12.1040611110721));
#55604=CARTESIAN_POINT('Ctrl Pts',(1.20156479510996,1.15416238768577,12.1051800151383));
#55605=CARTESIAN_POINT('Ctrl Pts',(1.18439096655243,1.17167789474204,12.10680360542));
#55606=CARTESIAN_POINT('Ctrl Pts',(1.17916122379466,1.17694088797136,12.1072972277283));
#55607=CARTESIAN_POINT('Ctrl Pts',(1.16999127903623,1.18604666760592,12.1081617753799));
#55608=CARTESIAN_POINT('Ctrl Pts',(1.16606691271147,1.18990514110198,12.1085314692338));
#55609=CARTESIAN_POINT('Ctrl Pts',(1.15760818457584,1.19813980797576,12.109327806577));
#55610=CARTESIAN_POINT('Ctrl Pts',(1.15306816731345,1.20250967009976,12.109754877645));
#55611=CARTESIAN_POINT('Ctrl Pts',(1.14051643118753,1.2144545438741,12.1109343803344));
#55612=CARTESIAN_POINT('Ctrl Pts',(1.1324543028324,1.22197577909172,12.1116906413558));
#55613=CARTESIAN_POINT('Ctrl Pts',(1.08578159058867,1.26465863084304,12.1160580460715));
#55614=CARTESIAN_POINT('Ctrl Pts',(1.04561283865277,1.29806616987811,12.1197746346321));
#55615=CARTESIAN_POINT('Ctrl Pts',(0.922274046945783,1.39120107235297,12.1309161614006));
#55616=CARTESIAN_POINT('Ctrl Pts',(0.835086336067767,1.44522055309898,12.1384389192172));
#55617=CARTESIAN_POINT('Ctrl Pts',(0.678451414407801,1.52333259106065,12.1509848903164));
#55618=CARTESIAN_POINT('Ctrl Pts',(0.611349752946374,1.55148077716466,12.1560918686487));
#55619=CARTESIAN_POINT('Ctrl Pts',(0.525970440413315,1.58089247275333,12.1622544186653));
#55620=CARTESIAN_POINT('Ctrl Pts',(0.509235591179539,1.5863622122864,12.1634471502125));
#55621=CARTESIAN_POINT('Ctrl Pts',(0.482168946347427,1.59473639646233,12.1653526557288));
#55622=CARTESIAN_POINT('Ctrl Pts',(0.471890694364649,1.5978079511958,12.1660708379894));
#55623=CARTESIAN_POINT('Ctrl Pts',(0.452178784730743,1.60349185995082,12.1674381273289));
#55624=CARTESIAN_POINT('Ctrl Pts',(0.442750406742478,1.60612075591902,12.1680877473068));
#55625=CARTESIAN_POINT('Ctrl Pts',(0.421168881415953,1.6119338058194,12.1695650651406));
#55626=CARTESIAN_POINT('Ctrl Pts',(0.409001693086385,1.61506391528166,12.1703909905131));
#55627=CARTESIAN_POINT('Ctrl Pts',(0.376411860189157,1.62305600188474,12.1725855563133));
#55628=CARTESIAN_POINT('Ctrl Pts',(0.355930373959067,1.62767020791043,12.1739463099901));
#55629=CARTESIAN_POINT('Ctrl Pts',(0.216869048068561,1.65624830838414,12.1830734005652));
#55630=CARTESIAN_POINT('Ctrl Pts',(0.0960700514466558,1.66762257067173,
12.1904204602756));
#55631=CARTESIAN_POINT('Ctrl Pts',(-0.120037404404096,1.66439148513532,
12.2036273793222));
#55632=CARTESIAN_POINT('Ctrl Pts',(-0.214858783860496,1.65482278637109,
12.2094576746848));
#55633=CARTESIAN_POINT('Ctrl Pts',(-0.319992476927955,1.63502344014951,
12.2164532582019));
#55634=CARTESIAN_POINT('Ctrl Pts',(-0.331630655418141,1.63270264400285,
12.2172352091307));
#55635=CARTESIAN_POINT('Ctrl Pts',(-0.349521847394895,1.62893574290971,
12.2184503404108));
#55636=CARTESIAN_POINT('Ctrl Pts',(-0.35579323712848,1.62757744679036,12.2188787620984));
#55637=CARTESIAN_POINT('Ctrl Pts',(-0.367408172061214,1.62499147544707,
12.2196770960556));
#55638=CARTESIAN_POINT('Ctrl Pts',(-0.372753692315715,1.62377361162524,
12.2200464566257));
#55639=CARTESIAN_POINT('Ctrl Pts',(-0.385017427150709,1.62091583100708,
12.2208982680414));
#55640=CARTESIAN_POINT('Ctrl Pts',(-0.391931234238567,1.61925799470271,
12.2213817054945));
#55641=CARTESIAN_POINT('Ctrl Pts',(-0.414163985967001,1.61377615752227,
12.2229462195415));
#55642=CARTESIAN_POINT('Ctrl Pts',(-0.429438721486368,1.60977875284756,
12.2240363141017));
#55643=CARTESIAN_POINT('Ctrl Pts',(-0.526400270201027,1.58292571174338,
12.2310435701363));
#55644=CARTESIAN_POINT('Ctrl Pts',(-0.606290870467466,1.55407840913979,
12.2372085575747));
#55645=CARTESIAN_POINT('Ctrl Pts',(-0.75147822819113,1.48874846248248,12.2487975812908));
#55646=CARTESIAN_POINT('Ctrl Pts',(-0.817210142405856,1.45370579912225,
12.254207674579));
#55647=CARTESIAN_POINT('Ctrl Pts',(-0.915369574617103,1.39260650838689,
12.2624425815092));
#55648=CARTESIAN_POINT('Ctrl Pts',(-0.949538563852768,1.36953690210696,
12.26534230662));
#55649=CARTESIAN_POINT('Ctrl Pts',(-1.00658334860366,1.32785998509348,12.2702373418834));
#55650=CARTESIAN_POINT('Ctrl Pts',(-1.02988448278311,1.30987034483122,12.2722534438722));
#55651=CARTESIAN_POINT('Ctrl Pts',(-1.06280307663763,1.28303374696575,12.275127859017));
#55652=CARTESIAN_POINT('Ctrl Pts',(-1.07281125854004,1.27467721243081,12.2760054202603));
#55653=CARTESIAN_POINT('Ctrl Pts',(-1.09018721170492,1.25981917679213,12.2775358684295));
#55654=CARTESIAN_POINT('Ctrl Pts',(-1.09759737086515,1.25336847469488,12.2781907851928));
#55655=CARTESIAN_POINT('Ctrl Pts',(-1.11289024136472,1.23981606157601,12.2795473205956));
#55656=CARTESIAN_POINT('Ctrl Pts',(-1.12076306475678,1.23270382385122,12.2802484592181));
#55657=CARTESIAN_POINT('Ctrl Pts',(-1.14111368830597,1.21396311370241,12.2820686357315));
#55658=CARTESIAN_POINT('Ctrl Pts',(-1.15348201128652,1.2022171916083,12.2831826457114));
#55659=CARTESIAN_POINT('Ctrl Pts',(-1.20603984639188,1.15074624494546,12.2879543169931));
#55660=CARTESIAN_POINT('Ctrl Pts',(-1.24437656200537,1.10917853015273,12.2915308551066));
#55661=CARTESIAN_POINT('Ctrl Pts',(-1.34855371515168,0.984005354277316,
12.3016748695222));
#55662=CARTESIAN_POINT('Ctrl Pts',(-1.40859442624594,0.89594928338679,12.3080627300279));
#55663=CARTESIAN_POINT('Ctrl Pts',(-1.48869650157309,0.75028446684585,12.3183189307649));
#55664=CARTESIAN_POINT('Ctrl Pts',(-1.51470510814306,0.696283674936131,
12.322066071126));
#55665=CARTESIAN_POINT('Ctrl Pts',(-1.54334682177581,0.627573411891013,
12.3269069115109));
#55666=CARTESIAN_POINT('Ctrl Pts',(-1.54876984199068,0.614068189093516,
12.3278618260956));
#55667=CARTESIAN_POINT('Ctrl Pts',(-1.55652241791239,0.594005349406701,
12.3292879272482));
#55668=CARTESIAN_POINT('Ctrl Pts',(-1.55898909311836,0.587500975144137,
12.3297514257693));
#55669=CARTESIAN_POINT('Ctrl Pts',(-1.56209021298762,0.579166570564681,
12.3303470399816));
#55670=CARTESIAN_POINT('Ctrl Pts',(-1.56276234322638,0.577350507380284,
12.3304769274012));
#55671=CARTESIAN_POINT('Ctrl Pts',(-1.56343130033211,0.57553329108042,12.3306070045052));
#55672=CARTESIAN_POINT('Origin',(0.,0.,11.));
#55673=CARTESIAN_POINT('',(-1.56343129955154,0.575533293200813,13.0328805013286));
#55674=CARTESIAN_POINT('',(-1.56343130043543,0.575533290799732,12.8376620384731));
#55675=CARTESIAN_POINT('',(-1.56343130033213,0.575533291080363,11.));
#55676=CARTESIAN_POINT('',(-1.66599979399416,-0.000828499501219724,12.1785196366098));
#55677=CARTESIAN_POINT('Ctrl Pts',(-1.56343130043543,0.575533290799732,
12.8376620384731));
#55678=CARTESIAN_POINT('Ctrl Pts',(-1.56057559831165,0.583290781385264,
12.8371017145145));
#55679=CARTESIAN_POINT('Ctrl Pts',(-1.55766210304294,0.591027169998756,
12.8365432982622));
#55680=CARTESIAN_POINT('Ctrl Pts',(-1.55073987019112,0.609001417257086,
12.8352466917295));
#55681=CARTESIAN_POINT('Ctrl Pts',(-1.54668715783039,0.619221864160468,
12.8345100178133));
#55682=CARTESIAN_POINT('Ctrl Pts',(-1.53922479276641,0.637510579794046,
12.8331926154892));
#55683=CARTESIAN_POINT('Ctrl Pts',(-1.53585215848513,0.645593412530058,
12.8326106698783));
#55684=CARTESIAN_POINT('Ctrl Pts',(-1.52777989022075,0.664518040901161,
12.8312486170692));
#55685=CARTESIAN_POINT('Ctrl Pts',(-1.52302829944338,0.675337271868922,
12.8304703028192));
#55686=CARTESIAN_POINT('Ctrl Pts',(-1.50876244240094,0.706903682303832,
12.8281998300067));
#55687=CARTESIAN_POINT('Ctrl Pts',(-1.49893623451018,0.727507505204777,
12.8267183497455));
#55688=CARTESIAN_POINT('Ctrl Pts',(-1.45157381147596,0.821781581506401,
12.8199314107458));
#55689=CARTESIAN_POINT('Ctrl Pts',(-1.40900838731808,0.892798509151854,
12.8148023101353));
#55690=CARTESIAN_POINT('Ctrl Pts',(-1.32830444365616,1.00719797834112,12.8062190730838));
#55691=CARTESIAN_POINT('Ctrl Pts',(-1.29287377565974,1.05229168349336,12.8027377532157));
#55692=CARTESIAN_POINT('Ctrl Pts',(-1.20454490719384,1.15349898951133,12.7944938526621));
#55693=CARTESIAN_POINT('Ctrl Pts',(-1.14994279741213,1.20793906736155,12.7897130855228));
#55694=CARTESIAN_POINT('Ctrl Pts',(-1.08301538323613,1.26600486988038,12.783917516342));
#55695=CARTESIAN_POINT('Ctrl Pts',(-1.07417154403224,1.27351722656889,12.7831528290758));
#55696=CARTESIAN_POINT('Ctrl Pts',(-1.06030574833672,1.28504827783642,12.7819543575631));
#55697=CARTESIAN_POINT('Ctrl Pts',(-1.05533757187814,1.28913147593223,12.7815250264043));
#55698=CARTESIAN_POINT('Ctrl Pts',(-1.04609202335394,1.29664085729999,12.7807259524591));
#55699=CARTESIAN_POINT('Ctrl Pts',(-1.0418212358962,1.30007482222813,12.7803567717288));
#55700=CARTESIAN_POINT('Ctrl Pts',(-1.03189264308965,1.30797765808361,12.7794984084989));
#55701=CARTESIAN_POINT('Ctrl Pts',(-1.02622271557862,1.31243091784007,12.7790081680065));
#55702=CARTESIAN_POINT('Ctrl Pts',(-1.00794004544287,1.32659953831916,12.7774276952099));
#55703=CARTESIAN_POINT('Ctrl Pts',(-0.995217312512813,1.33617061966191,
12.7763283276406));
#55704=CARTESIAN_POINT('Ctrl Pts',(-0.964345296447192,1.35870955519144,
12.7736655707429));
#55705=CARTESIAN_POINT('Ctrl Pts',(-0.946069195009378,1.37149789794062,
12.772093197122));
#55706=CARTESIAN_POINT('Ctrl Pts',(-0.873128305739834,1.4203851549974,12.7658492339669));
#55707=CARTESIAN_POINT('Ctrl Pts',(-0.816612995169159,1.45361251486965,
12.7610817536197));
#55708=CARTESIAN_POINT('Ctrl Pts',(-0.649713390930293,1.5389276661131,12.7474371352029));
#55709=CARTESIAN_POINT('Ctrl Pts',(-0.535349698712847,1.5823517018954,12.7386289212694));
#55710=CARTESIAN_POINT('Ctrl Pts',(-0.396987483619256,1.61814557882303,
12.7287985526631));
#55711=CARTESIAN_POINT('Ctrl Pts',(-0.376624201347912,1.6230059939517,12.7273706947822));
#55712=CARTESIAN_POINT('Ctrl Pts',(-0.343918433953247,1.6301636423514,12.7251066445784));
#55713=CARTESIAN_POINT('Ctrl Pts',(-0.331632784990003,1.63270729186905,
12.7242627056457));
#55714=CARTESIAN_POINT('Ctrl Pts',(-0.309715813490914,1.6369874338899,12.7227684205637));
#55715=CARTESIAN_POINT('Ctrl Pts',(-0.30009584153034,1.63877827565464,12.7221163748024));
#55716=CARTESIAN_POINT('Ctrl Pts',(-0.27989024504765,1.64235583326689,12.720754624417));
#55717=CARTESIAN_POINT('Ctrl Pts',(-0.269301974878431,1.64412520440636,
12.7200454968439));
#55718=CARTESIAN_POINT('Ctrl Pts',(-0.241269103423719,1.64853160736399,
12.7181793607935));
#55719=CARTESIAN_POINT('Ctrl Pts',(-0.22379814631042,1.65099414570989,12.7170278732524));
#55720=CARTESIAN_POINT('Ctrl Pts',(-0.133527473468258,1.66225851132056,
12.7111326006945));
#55721=CARTESIAN_POINT('Ctrl Pts',(-0.0602390778271082,1.66652517346292,
12.706532883713));
#55722=CARTESIAN_POINT('Ctrl Pts',(0.111340547297109,1.66517601317831,12.6959423211969));
#55723=CARTESIAN_POINT('Ctrl Pts',(0.209316410812084,1.65571537404338,12.6900350446318));
#55724=CARTESIAN_POINT('Ctrl Pts',(0.336620595046811,1.63193756917198,12.6820004291875));
#55725=CARTESIAN_POINT('Ctrl Pts',(0.367187292189199,1.62533287293225,12.6800421494094));
#55726=CARTESIAN_POINT('Ctrl Pts',(0.42471792522947,1.61119627539996,12.6762708310402));
#55727=CARTESIAN_POINT('Ctrl Pts',(0.451713090547941,1.60383721744689,12.6744647713115));
#55728=CARTESIAN_POINT('Ctrl Pts',(0.487343324507959,1.59315333881851,12.6720165602298));
#55729=CARTESIAN_POINT('Ctrl Pts',(0.496155992159062,1.59043085317141,12.6714057178708));
#55730=CARTESIAN_POINT('Ctrl Pts',(0.509961453357943,1.58604004444888,12.6704397745767));
#55731=CARTESIAN_POINT('Ctrl Pts',(0.5149698822242,1.58442094311208,12.6700874664156));
#55732=CARTESIAN_POINT('Ctrl Pts',(0.525293349519783,1.58102950252258,12.6693572372349));
#55733=CARTESIAN_POINT('Ctrl Pts',(0.53060719267888,1.57925406258393,12.6689791215216));
#55734=CARTESIAN_POINT('Ctrl Pts',(0.543537145119363,1.57486133615667,12.6680537437906));
#55735=CARTESIAN_POINT('Ctrl Pts',(0.551143369018455,1.57221558203638,12.6675048627041));
#55736=CARTESIAN_POINT('Ctrl Pts',(0.578621066940668,1.56243382572882,12.6655063773052));
#55737=CARTESIAN_POINT('Ctrl Pts',(0.598374692312269,1.55497569889347,12.6640399318227));
#55738=CARTESIAN_POINT('Ctrl Pts',(0.648462494777282,1.53496899546784,12.6602543374306));
#55739=CARTESIAN_POINT('Ctrl Pts',(0.678576629772541,1.52189583096448,12.6579143257129));
#55740=CARTESIAN_POINT('Ctrl Pts',(0.773563509689639,1.47728034296331,12.650365946967));
#55741=CARTESIAN_POINT('Ctrl Pts',(0.836782745962807,1.44241189649882,12.645089282005));
#55742=CARTESIAN_POINT('Ctrl Pts',(0.985840585672479,1.34709283443898,12.6322469940775));
#55743=CARTESIAN_POINT('Ctrl Pts',(1.06862684113967,1.28241361246042,12.6247686914399));
#55744=CARTESIAN_POINT('Ctrl Pts',(1.15841197934364,1.19749275930731,12.6163175807843));
#55745=CARTESIAN_POINT('Ctrl Pts',(1.17180970316557,1.18438561787403,12.6150457582739));
#55746=CARTESIAN_POINT('Ctrl Pts',(1.19276877017959,1.16317725201868,12.6130380046328));
#55747=CARTESIAN_POINT('Ctrl Pts',(1.20047505464536,1.15522219168414,12.6122957327183));
#55748=CARTESIAN_POINT('Ctrl Pts',(1.2147310974028,1.14020921432831,12.6109146536075));
#55749=CARTESIAN_POINT('Ctrl Pts',(1.22130006555649,1.13317026432942,12.6102750327436));
#55750=CARTESIAN_POINT('Ctrl Pts',(1.23600017438321,1.11714210138051,12.6088360295651));
#55751=CARTESIAN_POINT('Ctrl Pts',(1.24409503467342,1.10812023869926,12.6080382005021));
#55752=CARTESIAN_POINT('Ctrl Pts',(1.2681716320533,1.08069003240263,12.6056478633689));
#55753=CARTESIAN_POINT('Ctrl Pts',(1.28384895068836,1.06201798710102,12.6040678684018));
#55754=CARTESIAN_POINT('Ctrl Pts',(1.31916609333923,1.01802895199933,12.6004460351622));
#55755=CARTESIAN_POINT('Ctrl Pts',(1.33849691329658,0.992475858893271,12.5984158074655));
#55756=CARTESIAN_POINT('Ctrl Pts',(1.40697996922379,0.896305644707766,12.5910091483143));
#55757=CARTESIAN_POINT('Ctrl Pts',(1.45137863982918,0.822470423455903,12.5857786008085));
#55758=CARTESIAN_POINT('Ctrl Pts',(1.53022645030923,0.664900465330985,12.5750134057199));
#55759=CARTESIAN_POINT('Ctrl Pts',(1.56395752351259,0.581135370906246,12.5694919535862));
#55760=CARTESIAN_POINT('Ctrl Pts',(1.59541098557232,0.480069234958713,12.5626236415821));
#55761=CARTESIAN_POINT('Ctrl Pts',(1.59986569041235,0.465007969949144,12.5615947547427));
#55762=CARTESIAN_POINT('Ctrl Pts',(1.60602248540584,0.443055428413562,12.560084326015));
#55763=CARTESIAN_POINT('Ctrl Pts',(1.60789466686261,0.436212186879269,12.559611972826));
#55764=CARTESIAN_POINT('Ctrl Pts',(1.61113555908841,0.42406161146778,12.5587702683391));
#55765=CARTESIAN_POINT('Ctrl Pts',(1.61252187288238,0.418759176941351,12.5584019279243));
#55766=CARTESIAN_POINT('Ctrl Pts',(1.61547692785096,0.407224259435909,12.5575983193294));
#55767=CARTESIAN_POINT('Ctrl Pts',(1.61703575545577,0.400989605828504,12.5571625315986));
#55768=CARTESIAN_POINT('Ctrl Pts',(1.62138155909899,0.38317072178033,12.5559132476047));
#55769=CARTESIAN_POINT('Ctrl Pts',(1.62408032073768,0.371565678825545,12.5550950647572));
#55770=CARTESIAN_POINT('Ctrl Pts',(1.6299522551859,0.345028505677191,12.5532152945406));
#55771=CARTESIAN_POINT('Ctrl Pts',(1.63304509380198,0.330079852204156,12.552150059365));
#55772=CARTESIAN_POINT('Ctrl Pts',(1.66343390912173,0.172303309547315,12.5408546389933));
#55773=CARTESIAN_POINT('Ctrl Pts',(1.67212456616911,0.0265298737222167,
12.5300370154238));
#55774=CARTESIAN_POINT('Ctrl Pts',(1.65713143432942,-0.183678472453655,
12.5149876719441));
#55775=CARTESIAN_POINT('Ctrl Pts',(1.6486565614359,-0.248507224866853,12.5104117126023));
#55776=CARTESIAN_POINT('Ctrl Pts',(1.63308638494221,-0.329993348806482,
12.5047500513115));
#55777=CARTESIAN_POINT('Ctrl Pts',(1.62950318735082,-0.347255172485597,
12.5035556776559));
#55778=CARTESIAN_POINT('Ctrl Pts',(1.62329888724151,-0.37492918146853,12.5016482219629));
#55779=CARTESIAN_POINT('Ctrl Pts',(1.62085003620628,-0.385378175157583,
12.5009297112279));
#55780=CARTESIAN_POINT('Ctrl Pts',(1.61597548857948,-0.405308499689075,
12.4995622183109));
#55781=CARTESIAN_POINT('Ctrl Pts',(1.61356689121204,-0.414793507863377,
12.4989127192926));
#55782=CARTESIAN_POINT('Ctrl Pts',(1.60782412232259,-0.436601120012205,
12.4974221321239));
#55783=CARTESIAN_POINT('Ctrl Pts',(1.60443158870425,-0.448907828584265,
12.4965829621367));
#55784=CARTESIAN_POINT('Ctrl Pts',(1.59318436874859,-0.487950849599055,
12.4939260728876));
#55785=CARTESIAN_POINT('Ctrl Pts',(1.58479998059536,-0.514530495347398,
12.4921254832463));
#55786=CARTESIAN_POINT('Ctrl Pts',(1.55184338920774,-0.610541811953956,
12.4856351875206));
#55787=CARTESIAN_POINT('Ctrl Pts',(1.52334121620919,-0.678536924626257,
12.4810697436467));
#55788=CARTESIAN_POINT('Ctrl Pts',(1.43231860924841,-0.860774525529232,
12.4685766669968));
#55789=CARTESIAN_POINT('Ctrl Pts',(1.36079280440545,-0.969898085276284,
12.4608133479951));
#55790=CARTESIAN_POINT('Ctrl Pts',(1.26754856362993,-1.08125319969806,12.4513805824067));
#55791=CARTESIAN_POINT('Ctrl Pts',(1.25761399258041,-1.0927922257186,12.4503824612273));
#55792=CARTESIAN_POINT('Ctrl Pts',(1.24282874878284,-1.10949667303317,12.4489041040428));
#55793=CARTESIAN_POINT('Ctrl Pts',(1.23810072629406,-1.11477026927804,12.448432388812));
#55794=CARTESIAN_POINT('Ctrl Pts',(1.2296622037612,-1.12406262361142,12.4475919526881));
#55795=CARTESIAN_POINT('Ctrl Pts',(1.2259653342221,-1.12809348678403,12.4472242407048));
#55796=CARTESIAN_POINT('Ctrl Pts',(1.21781710387063,-1.13689050910773,12.4464147379689));
#55797=CARTESIAN_POINT('Ctrl Pts',(1.21335764663822,-1.14164869635495,12.4459723597842));
#55798=CARTESIAN_POINT('Ctrl Pts',(1.20035988693036,-1.15535497288458,12.4446851914861));
#55799=CARTESIAN_POINT('Ctrl Pts',(1.19174994487353,-1.1642340906382,12.4438352771806));
#55800=CARTESIAN_POINT('Ctrl Pts',(1.1717634146485,-1.18439145099116,12.4418702398946));
#55801=CARTESIAN_POINT('Ctrl Pts',(1.16032153265617,-1.19560298934976,12.4407510056824));
#55802=CARTESIAN_POINT('Ctrl Pts',(1.12096389207017,-1.23307120188708,12.4369254454263));
#55803=CARTESIAN_POINT('Ctrl Pts',(1.09230574309102,-1.25852788137488,12.4341806519727));
#55804=CARTESIAN_POINT('Ctrl Pts',(1.00799976108115,-1.32836585757318,12.4262738327249));
#55805=CARTESIAN_POINT('Ctrl Pts',(0.950350454453864,-1.37020196613827,
12.4210669315802));
#55806=CARTESIAN_POINT('Ctrl Pts',(0.807994396116067,-1.46019174264913,
12.4088670573473));
#55807=CARTESIAN_POINT('Ctrl Pts',(0.721381755008904,-1.50486847168071,
12.4019509044062));
#55808=CARTESIAN_POINT('Ctrl Pts',(0.613886306307181,-1.54888856190578,
12.3940085432739));
#55809=CARTESIAN_POINT('Ctrl Pts',(0.596300533029561,-1.55574351980763,
12.3927280323966));
#55810=CARTESIAN_POINT('Ctrl Pts',(0.568287874932052,-1.56611808314776,
12.3907170993207));
#55811=CARTESIAN_POINT('Ctrl Pts',(0.557936541988382,-1.56983559149122,
12.3899801489876));
#55812=CARTESIAN_POINT('Ctrl Pts',(0.539278000104317,-1.57632862410038,
12.3886625029863));
#55813=CARTESIAN_POINT('Ctrl Pts',(0.53098436640402,-1.57914163398914,12.3880805873817));
#55814=CARTESIAN_POINT('Ctrl Pts',(0.511454572329717,-1.58559443376058,
12.3867189253395));
#55815=CARTESIAN_POINT('Ctrl Pts',(0.500201027098248,-1.58918042790537,
12.3859409684182));
#55816=CARTESIAN_POINT('Ctrl Pts',(0.467117947049906,-1.59933625980721,
12.3836726594754));
#55817=CARTESIAN_POINT('Ctrl Pts',(0.445190034989375,-1.60557826419364,
12.3821929539685));
#55818=CARTESIAN_POINT('Ctrl Pts',(0.343385113452899,-1.63231189911165,
12.3754216020902));
#55819=CARTESIAN_POINT('Ctrl Pts',(0.262180733524004,-1.64730660142348,
12.370305319463));
#55820=CARTESIAN_POINT('Ctrl Pts',(0.123064555626081,-1.66244195409447,
12.3617253778789));
#55821=CARTESIAN_POINT('Ctrl Pts',(0.0656546454323221,-1.66569731025476,
12.3582347937311));
#55822=CARTESIAN_POINT('Ctrl Pts',(-0.0689381260133705,-1.66635911481172,
12.3499750616312));
#55823=CARTESIAN_POINT('Ctrl Pts',(-0.145991509935956,-1.66138150591947,
12.3451878925344));
#55824=CARTESIAN_POINT('Ctrl Pts',(-0.233912265440251,-1.64953803028404,
12.3393851690594));
#55825=CARTESIAN_POINT('Ctrl Pts',(-0.245395861825237,-1.64786877929135,
12.3386204528906));
#55826=CARTESIAN_POINT('Ctrl Pts',(-0.263214778905215,-1.64508824619619,
12.3374219455859));
#55827=CARTESIAN_POINT('Ctrl Pts',(-0.269562944418963,-1.6440599664044,
12.3369926079593));
#55828=CARTESIAN_POINT('Ctrl Pts',(-0.281309516236458,-1.64208738807223,
12.3361935285534));
#55829=CARTESIAN_POINT('Ctrl Pts',(-0.286709408311424,-1.64115317566291,
12.3358243489025));
#55830=CARTESIAN_POINT('Ctrl Pts',(-0.299202503155856,-1.63892825983488,
12.3349659969122));
#55831=CARTESIAN_POINT('Ctrl Pts',(-0.306292006985218,-1.63761814242546,
12.3344757666785));
#55832=CARTESIAN_POINT('Ctrl Pts',(-0.32900837952904,-1.63326756240484,
12.3328953607541));
#55833=CARTESIAN_POINT('Ctrl Pts',(-0.344599713090734,-1.63004921264532,
12.3317960508413));
#55834=CARTESIAN_POINT('Ctrl Pts',(-0.381917767605521,-1.62178674822694,
12.3291334610089));
#55835=CARTESIAN_POINT('Ctrl Pts',(-0.403593648455485,-1.61652884432489,
12.3275611981952));
#55836=CARTESIAN_POINT('Ctrl Pts',(-0.488485698902753,-1.59412286814509,
12.3213179159231));
#55837=CARTESIAN_POINT('Ctrl Pts',(-0.550770955754018,-1.57368880392259,
12.3165510240262));
#55838=CARTESIAN_POINT('Ctrl Pts',(-0.725134649075396,-1.50486250417439,
12.3029053168529));
#55839=CARTESIAN_POINT('Ctrl Pts',(-0.833341213322183,-1.44775142919914,
12.2940954314001));
#55840=CARTESIAN_POINT('Ctrl Pts',(-0.951679353126265,-1.3675892298811,
12.2842640524843));
#55841=CARTESIAN_POINT('Ctrl Pts',(-0.968782440150438,-1.35552740491392,
12.2828366669265));
#55842=CARTESIAN_POINT('Ctrl Pts',(-0.995767213079444,-1.33572489658619,
12.2805732145575));
#55843=CARTESIAN_POINT('Ctrl Pts',(-1.00579609052524,-1.32818958783254,
12.2797294076052));
#55844=CARTESIAN_POINT('Ctrl Pts',(-1.02327447208066,-1.31474550010255,
12.2782538767596));
#55845=CARTESIAN_POINT('Ctrl Pts',(-1.03076017683544,-1.30888496039293,
12.2776203020706));
#55846=CARTESIAN_POINT('Ctrl Pts',(-1.04614409617535,-1.29662709516369,
12.2763146276187));
#55847=CARTESIAN_POINT('Ctrl Pts',(-1.05403477236289,-1.29022091141695,
12.2756429168749));
#55848=CARTESIAN_POINT('Ctrl Pts',(-1.07294992336873,-1.27457496983093,
12.2740274704699));
#55849=CARTESIAN_POINT('Ctrl Pts',(-1.08391444466818,-1.26526376285485,
12.2730866614192));
#55850=CARTESIAN_POINT('Ctrl Pts',(-1.10838038931192,-1.24393550483927,
12.2709761998746));
#55851=CARTESIAN_POINT('Ctrl Pts',(-1.12180972911259,-1.23183830049405,
12.2698098774782));
#55852=CARTESIAN_POINT('Ctrl Pts',(-1.16042215702941,-1.19590081336927,
12.266429461949));
#55853=CARTESIAN_POINT('Ctrl Pts',(-1.18506172067924,-1.17148934595956,
12.2642379928043));
#55854=CARTESIAN_POINT('Ctrl Pts',(-1.2698678103973,-1.0820522583828,12.25653001053));
#55855=CARTESIAN_POINT('Ctrl Pts',(-1.32559085351529,-1.01302078397566,
12.2511600030804));
#55856=CARTESIAN_POINT('Ctrl Pts',(-1.3802732333519,-0.932990624174738,
12.2452308882704));
#55857=CARTESIAN_POINT('Ctrl Pts',(-1.38493139246276,-0.926061952883341,
12.2447197628913));
#55858=CARTESIAN_POINT('Ctrl Pts',(-1.4339603460905,-0.851937633190046,
12.2392719570824));
#55859=CARTESIAN_POINT('Ctrl Pts',(-1.47345005913669,-0.781653017104703,
12.2342862640505));
#55860=CARTESIAN_POINT('Ctrl Pts',(-1.51264908651603,-0.698272213346401,
12.2282602124022));
#55861=CARTESIAN_POINT('Ctrl Pts',(-1.5174880631557,-0.687692738367644,
12.2274936026497));
#55862=CARTESIAN_POINT('Ctrl Pts',(-1.52483189046305,-0.671181903325557,
12.226292750525));
#55863=CARTESIAN_POINT('Ctrl Pts',(-1.52741393073529,-0.665284993248127,
12.2258629893137));
#55864=CARTESIAN_POINT('Ctrl Pts',(-1.53213033520592,-0.654341394089419,
12.2250635514958));
#55865=CARTESIAN_POINT('Ctrl Pts',(-1.53427405628802,-0.649298961271169,
12.224694441734));
#55866=CARTESIAN_POINT('Ctrl Pts',(-1.53917710858784,-0.637606201714705,
12.2238368222859));
#55867=CARTESIAN_POINT('Ctrl Pts',(-1.54191822992249,-0.630948498279305,
12.2233472611282));
#55868=CARTESIAN_POINT('Ctrl Pts',(-1.55056147758728,-0.609562837458039,
12.2217712124408));
#55869=CARTESIAN_POINT('Ctrl Pts',(-1.55629618887594,-0.594768757769509,
12.2206756585349));
#55870=CARTESIAN_POINT('Ctrl Pts',(-1.58699466918464,-0.512089318036046,
12.2145324142179));
#55871=CARTESIAN_POINT('Ctrl Pts',(-1.60772601932432,-0.442721744933113,
12.2093051861428));
#55872=CARTESIAN_POINT('Ctrl Pts',(-1.6517995721916,-0.250449698524759,
12.1949625177314));
#55873=CARTESIAN_POINT('Ctrl Pts',(-1.66593062834089,-0.125894015948298,
12.1858615843024));
#55874=CARTESIAN_POINT('Ctrl Pts',(-1.6659997452095,-0.000921391271100774,
12.1771821268692));
#55875=CARTESIAN_POINT('Ctrl Pts',(-1.66599979399416,-0.000828499501219724,
12.1785196366098));
#55876=CARTESIAN_POINT('Ctrl Pts',(-1.66603059434109,0.0611068083237465,
12.1743970351476));
#55877=CARTESIAN_POINT('Ctrl Pts',(-1.66260328405743,0.123036889626019,
12.1702744336855));
#55878=CARTESIAN_POINT('Ctrl Pts',(-1.65574596036209,0.18455707720003,12.1661518322233));
#55879=CARTESIAN_POINT('Ctrl Pts',(-1.64888676465322,0.246094059463739,
12.1620281053125));
#55880=CARTESIAN_POINT('Ctrl Pts',(-1.63859576107942,0.307220439264669,
12.1579043784017));
#55881=CARTESIAN_POINT('Ctrl Pts',(-1.62495263499754,0.367539023798209,
12.1537806514908));
#55882=CARTESIAN_POINT('Ctrl Pts',(-1.61129538063748,0.427920071856396,
12.1496526542126));
#55883=CARTESIAN_POINT('Ctrl Pts',(-1.59427920275196,0.487491181084654,
12.1455246569344));
#55884=CARTESIAN_POINT('Ctrl Pts',(-1.57403402702575,0.545868923611786,
12.1413966596562));
#55885=CARTESIAN_POINT('Ctrl Pts',(-1.57059271091171,0.555792090927155,
12.1406949742895));
#55886=CARTESIAN_POINT('Ctrl Pts',(-1.56705820997352,0.565680821823223,
12.1399932889229));
#55887=CARTESIAN_POINT('Ctrl Pts',(-1.56343130033213,0.575533291080363,
12.1392916035562));
#55888=CARTESIAN_POINT('Ctrl Pts',(-1.56343130033211,0.57553329108042,12.3306070045052));
#55889=CARTESIAN_POINT('Ctrl Pts',(-1.56446758603764,0.572718229756892,
12.3308085077741));
#55890=CARTESIAN_POINT('Ctrl Pts',(-1.56549625706293,0.569900401527806,
12.3310104699606));
#55891=CARTESIAN_POINT('Ctrl Pts',(-1.56869220479126,0.561071824407949,
12.3316440473536));
#55892=CARTESIAN_POINT('Ctrl Pts',(-1.57083245714038,0.555051541463941,
12.3320772473261));
#55893=CARTESIAN_POINT('Ctrl Pts',(-1.57670050032788,0.538239620125473,
12.3332899072989));
#55894=CARTESIAN_POINT('Ctrl Pts',(-1.58035198047519,0.527421990685742,
12.3340735414443));
#55895=CARTESIAN_POINT('Ctrl Pts',(-1.60364844798922,0.455990774229675,
12.3392661468574));
#55896=CARTESIAN_POINT('Ctrl Pts',(-1.61991141185927,0.394336341501583,
12.3438315550567));
#55897=CARTESIAN_POINT('Ctrl Pts',(-1.65472577035379,0.223091012756832,
12.3564903812482));
#55898=CARTESIAN_POINT('Ctrl Pts',(-1.66591584845416,0.112320009136745,
12.3646350425551));
#55899=CARTESIAN_POINT('Ctrl Pts',(-1.66603996118025,-0.0524117735343192,
12.3763075003104));
#55900=CARTESIAN_POINT('Ctrl Pts',(-1.66348724514481,-0.106053903022186,
12.3800442000452));
#55901=CARTESIAN_POINT('Ctrl Pts',(-1.6567543340318,-0.176063883185556,
12.3848366249681));
#55902=CARTESIAN_POINT('Ctrl Pts',(-1.65491131019478,-0.192618806661558,
12.3859637759678));
#55903=CARTESIAN_POINT('Ctrl Pts',(-1.65149915185674,-0.219584383903663,
12.387790395302));
#55904=CARTESIAN_POINT('Ctrl Pts',(-1.65007910939348,-0.2300123730685,12.3884944891604));
#55905=CARTESIAN_POINT('Ctrl Pts',(-1.64713786441424,-0.250179956294903,
12.3898520149602));
#55906=CARTESIAN_POINT('Ctrl Pts',(-1.64562884995618,-0.259920853771098,
12.3905058004801));
#55907=CARTESIAN_POINT('Ctrl Pts',(-1.64188875601092,-0.282724065010168,
12.3920321490832));
#55908=CARTESIAN_POINT('Ctrl Pts',(-1.63958808776659,-0.295774412888371,
12.3929024785311));
#55909=CARTESIAN_POINT('Ctrl Pts',(-1.63144104614049,-0.338967237042632,
12.3957736101069));
#55910=CARTESIAN_POINT('Ctrl Pts',(-1.62491697459146,-0.368976545595315,
12.3977530157594));
#55911=CARTESIAN_POINT('Ctrl Pts',(-1.60711224551937,-0.441195860488513,
12.4024938837271));
#55912=CARTESIAN_POINT('Ctrl Pts',(-1.59499364553735,-0.483176198129534,
12.405230313708));
#55913=CARTESIAN_POINT('Ctrl Pts',(-1.55831024370868,-0.593739349029494,
12.412449563597));
#55914=CARTESIAN_POINT('Ctrl Pts',(-1.53087599955039,-0.661268668922863,
12.4168694850393));
#55915=CARTESIAN_POINT('Ctrl Pts',(-1.49197226807926,-0.741513728241527,
12.4223249799457));
#55916=CARTESIAN_POINT('Ctrl Pts',(-1.48461594090737,-0.756134482598804,
12.4233278169476));
#55917=CARTESIAN_POINT('Ctrl Pts',(-1.44364627026296,-0.834658470757961,
12.4287732003365));
#55918=CARTESIAN_POINT('Ctrl Pts',(-1.40612496149368,-0.89642582148789,
12.4332700962649));
#55919=CARTESIAN_POINT('Ctrl Pts',(-1.35807678677339,-0.965048022709284,
12.4387496928834));
#55920=CARTESIAN_POINT('Ctrl Pts',(-1.35133264153374,-0.974469249592769,
12.4395132499669));
#55921=CARTESIAN_POINT('Ctrl Pts',(-1.34069557866648,-0.989005902002203,
12.4407103353552));
#55922=CARTESIAN_POINT('Ctrl Pts',(-1.33687023778565,-0.994170645669132,
12.4411394271612));
#55923=CARTESIAN_POINT('Ctrl Pts',(-1.32975869781132,-1.0036569534013,12.4419348232516));
#55924=CARTESIAN_POINT('Ctrl Pts',(-1.3264811421569,-1.00798474736811,12.4423005392839));
#55925=CARTESIAN_POINT('Ctrl Pts',(-1.31881663185041,-1.01800310352015,
12.4431537187448));
#55926=CARTESIAN_POINT('Ctrl Pts',(-1.3144139771517,-1.0236813562338,12.4436422511729));
#55927=CARTESIAN_POINT('Ctrl Pts',(-1.30022301681158,-1.04174144008166,
12.4452115325764));
#55928=CARTESIAN_POINT('Ctrl Pts',(-1.29029576155259,-1.05401229782464,
12.4463012426588));
#55929=CARTESIAN_POINT('Ctrl Pts',(-1.23445003931559,-1.12107056235004,
12.4523790691956));
#55930=CARTESIAN_POINT('Ctrl Pts',(-1.18522021283528,-1.1729949451118,12.4575428747315));
#55931=CARTESIAN_POINT('Ctrl Pts',(-1.03648388078091,-1.31092199938641,
12.4722894813691));
#55932=CARTESIAN_POINT('Ctrl Pts',(-0.929906078632625,-1.38856104739653,
12.4818583442618));
#55933=CARTESIAN_POINT('Ctrl Pts',(-0.791325093235982,-1.4663274900714,
12.4928494127712));
#55934=CARTESIAN_POINT('Ctrl Pts',(-0.767021162759265,-1.47918572286742,
12.4947304894388));
#55935=CARTESIAN_POINT('Ctrl Pts',(-0.730991711486161,-1.49712049200004,
12.4974534308588));
#55936=CARTESIAN_POINT('Ctrl Pts',(-0.719509436847579,-1.50267256440613,
12.4983116955461));
#55937=CARTESIAN_POINT('Ctrl Pts',(-0.699079505529343,-1.51226326414033,
12.4998223817845));
#55938=CARTESIAN_POINT('Ctrl Pts',(-0.690157910212084,-1.51635563149986,
12.5004766333418));
#55939=CARTESIAN_POINT('Ctrl Pts',(-0.671494076266293,-1.52471795218344,
12.5018342400799));
#55940=CARTESIAN_POINT('Ctrl Pts',(-0.661746039972998,-1.52897394209645,
12.5025370940772));
#55941=CARTESIAN_POINT('Ctrl Pts',(-0.636146653580155,-1.53985993886215,
12.5043671276162));
#55942=CARTESIAN_POINT('Ctrl Pts',(-0.620232066946704,-1.54633871294533,
12.505489175088));
#55943=CARTESIAN_POINT('Ctrl Pts',(-0.542555749103448,-1.5765682961704,
12.5108946335196));
#55944=CARTESIAN_POINT('Ctrl Pts',(-0.479512761874191,-1.59687299700896,
12.5150626776159));
#55945=CARTESIAN_POINT('Ctrl Pts',(-0.345211393460327,-1.63145381770276,
12.523655080517));
#55946=CARTESIAN_POINT('Ctrl Pts',(-0.273893291767488,-1.64493017053553,
12.5280562357795));
#55947=CARTESIAN_POINT('Ctrl Pts',(-0.183201766622668,-1.65600388313279,
12.5336457290519));
#55948=CARTESIAN_POINT('Ctrl Pts',(-0.164442267148961,-1.65797179487159,
12.5348017809404));
#55949=CARTESIAN_POINT('Ctrl Pts',(-0.0763489424746476,-1.66570314723546,
12.5402448789092));
#55950=CARTESIAN_POINT('Ctrl Pts',(-0.00673961622210144,-1.66743764353843,
12.5445860086788));
#55951=CARTESIAN_POINT('Ctrl Pts',(0.0743107810027824,-1.66438199013478,
12.54989178074));
#55952=CARTESIAN_POINT('Ctrl Pts',(0.0858516173689782,-1.66382660838408,
12.5506532629449));
#55953=CARTESIAN_POINT('Ctrl Pts',(0.103794408001332,-1.6627759734235,12.5518477785519));
#55954=CARTESIAN_POINT('Ctrl Pts',(0.110201114114792,-1.66236365694203,
12.5522764056177));
#55955=CARTESIAN_POINT('Ctrl Pts',(0.122021906417831,-1.66153427293247,
12.5530714114351));
#55956=CARTESIAN_POINT('Ctrl Pts',(0.127436532699472,-1.66112775330455,
12.5534372071176));
#55957=CARTESIAN_POINT('Ctrl Pts',(0.14002192729201,-1.66012097134327,12.5542911957228));
#55958=CARTESIAN_POINT('Ctrl Pts',(0.147190859989878,-1.65950071574014,
12.5547804646773));
#55959=CARTESIAN_POINT('Ctrl Pts',(0.170129346847267,-1.65736627746899,
12.5563545289229));
#55960=CARTESIAN_POINT('Ctrl Pts',(0.185880867914779,-1.65567364828763,
12.5574483593736));
#55961=CARTESIAN_POINT('Ctrl Pts',(0.273152607026711,-1.64503458079424,
12.5635720843458));
#55962=CARTESIAN_POINT('Ctrl Pts',(0.344051883962195,-1.63167931265417,
12.5687803620079));
#55963=CARTESIAN_POINT('Ctrl Pts',(0.542927146236723,-1.58067742148149,
12.5837078260743));
#55964=CARTESIAN_POINT('Ctrl Pts',(0.667587267516383,-1.53220455268447,
12.5934075863587));
#55965=CARTESIAN_POINT('Ctrl Pts',(0.80821909880595,-1.45705934765141,12.6044144112106));
#55966=CARTESIAN_POINT('Ctrl Pts',(0.830994490755951,-1.44419124248433,
12.6062013486946));
#55967=CARTESIAN_POINT('Ctrl Pts',(0.864156121751638,-1.42441052768645,
12.6088111500678));
#55968=CARTESIAN_POINT('Ctrl Pts',(0.874781985215312,-1.41790960470397,
12.6096486564339));
#55969=CARTESIAN_POINT('Ctrl Pts',(0.893592443344653,-1.40610937780125,
12.6111338497161));
#55970=CARTESIAN_POINT('Ctrl Pts',(0.901805207791379,-1.40085631357486,
12.6117831936628));
#55971=CARTESIAN_POINT('Ctrl Pts',(0.919098340835933,-1.38958013639452,
12.6131526373275));
#55972=CARTESIAN_POINT('Ctrl Pts',(0.92816671578582,-1.38353940052268,12.613872042054));
#55973=CARTESIAN_POINT('Ctrl Pts',(0.952380877821386,-1.36706433801552,
12.6157969559625));
#55974=CARTESIAN_POINT('Ctrl Pts',(0.967414506755512,-1.35646727071466,
12.6169962885753));
#55975=CARTESIAN_POINT('Ctrl Pts',(1.0542060815529,-1.29311166392279,12.6239517940272));
#55976=CARTESIAN_POINT('Ctrl Pts',(1.12182017033327,-1.23491325611185,12.6294881295165));
#55977=CARTESIAN_POINT('Ctrl Pts',(1.27605995464213,-1.0789773905794,12.6429400603205));
#55978=CARTESIAN_POINT('Ctrl Pts',(1.35646620014991,-0.97596648887954,12.6507144487269));
#55979=CARTESIAN_POINT('Ctrl Pts',(1.43192817028973,-0.851685563546782,
12.6601581807319));
#55980=CARTESIAN_POINT('Ctrl Pts',(1.43963111942049,-0.838599298970701,
12.6611536457715));
#55981=CARTESIAN_POINT('Ctrl Pts',(1.4506592312883,-0.819264215803973,12.662628809302));
#55982=CARTESIAN_POINT('Ctrl Pts',(1.45412540737038,-0.813096154040623,
12.6631000395227));
#55983=CARTESIAN_POINT('Ctrl Pts',(1.4602011441877,-0.802121270628105,12.6639399754963));
#55984=CARTESIAN_POINT('Ctrl Pts',(1.46282647380285,-0.797323410095747,
12.6643076774426));
#55985=CARTESIAN_POINT('Ctrl Pts',(1.46853338856125,-0.786770803510303,
12.6651176047101));
#55986=CARTESIAN_POINT('Ctrl Pts',(1.47160475180358,-0.78101092271485,12.6655604217574));
#55987=CARTESIAN_POINT('Ctrl Pts',(1.4804110650728,-0.764259628556052,12.6668500635657));
#55988=CARTESIAN_POINT('Ctrl Pts',(1.48605712722863,-0.7532223398701,12.6677020414222));
#55989=CARTESIAN_POINT('Ctrl Pts',(1.49873688770819,-0.727737540787147,
12.6696726361898));
#55990=CARTESIAN_POINT('Ctrl Pts',(1.50568571572696,-0.713249374451216,
12.6707953953461));
#55991=CARTESIAN_POINT('Ctrl Pts',(1.52857012660578,-0.663710620119195,
12.6746373982194));
#55992=CARTESIAN_POINT('Ctrl Pts',(1.5434991234233,-0.628210553659201,12.677395433115));
#55993=CARTESIAN_POINT('Ctrl Pts',(1.5824120914602,-0.525894072596553,12.6853025272015));
#55994=CARTESIAN_POINT('Ctrl Pts',(1.60337565580648,-0.458016548948634,
12.6904955002919));
#55995=CARTESIAN_POINT('Ctrl Pts',(1.64263487650365,-0.294529692479793,
12.7026747881614));
#55996=CARTESIAN_POINT('Ctrl Pts',(1.65701733547024,-0.198233437646106,
12.7095841718912));
#55997=CARTESIAN_POINT('Ctrl Pts',(1.66406909268071,-0.0823788135472152,
12.7175203561996));
#55998=CARTESIAN_POINT('Ctrl Pts',(1.66489558599313,-0.0635212777457633,
12.7188009401027));
#55999=CARTESIAN_POINT('Ctrl Pts',(1.66569627834598,-0.0336582903609436,
12.7208119855056));
#56000=CARTESIAN_POINT('Ctrl Pts',(1.6658821920898,-0.0226606338558027,
12.7215489758778));
#56001=CARTESIAN_POINT('Ctrl Pts',(1.66602048830805,-0.00290402437482544,
12.7228666931106));
#56002=CARTESIAN_POINT('Ctrl Pts',(1.66601273547824,0.00585414840646092,
12.7234486400382));
#56003=CARTESIAN_POINT('Ctrl Pts',(1.66583232787135,0.0264226917070504,
12.7248103758247));
#56004=CARTESIAN_POINT('Ctrl Pts',(1.66560313832769,0.0382321962668288,
12.7255883749658));
#56005=CARTESIAN_POINT('Ctrl Pts',(1.66456365857613,0.0728253820508035,
12.7278568127073));
#56006=CARTESIAN_POINT('Ctrl Pts',(1.66341127719024,0.0955966211118545,
12.7293366035104));
#56007=CARTESIAN_POINT('Ctrl Pts',(1.65593420860147,0.200595318176297,12.7361084636989));
#56008=CARTESIAN_POINT('Ctrl Pts',(1.64397703088971,0.282309070224945,12.7412251398327));
#56009=CARTESIAN_POINT('Ctrl Pts',(1.61350224552191,0.418889046400651,12.749805149775));
#56010=CARTESIAN_POINT('Ctrl Pts',(1.59809654389551,0.474283556633144,12.7532954166224));
#56011=CARTESIAN_POINT('Ctrl Pts',(1.55538074100362,0.601909665500186,12.7615545692918));
#56012=CARTESIAN_POINT('Ctrl Pts',(1.52585534103527,0.673250947316369,12.766341481159));
#56013=CARTESIAN_POINT('Ctrl Pts',(1.4863304897064,0.752670143702575,12.7721439405539));
#56014=CARTESIAN_POINT('Ctrl Pts',(1.48105180524546,0.763004719197057,12.7729086806488));
#56015=CARTESIAN_POINT('Ctrl Pts',(1.47268066488823,0.778979473758189,12.7741072310869));
#56016=CARTESIAN_POINT('Ctrl Pts',(1.46966265675198,0.784658545579505,12.7745365876939));
#56017=CARTESIAN_POINT('Ctrl Pts',(1.46401199251504,0.795144592612918,12.775335707109));
#56018=CARTESIAN_POINT('Ctrl Pts',(1.46138840695088,0.799956222695908,12.7757049077776));
#56019=CARTESIAN_POINT('Ctrl Pts',(1.45525830521939,0.811067969752821,12.7765633172911));
#56020=CARTESIAN_POINT('Ctrl Pts',(1.45173459718152,0.817358330830522,12.7770535842369));
#56021=CARTESIAN_POINT('Ctrl Pts',(1.44029902542701,0.837465352001482,12.77863414495));
#56022=CARTESIAN_POINT('Ctrl Pts',(1.43223015916051,0.851191061589421,12.77973357495));
#56023=CARTESIAN_POINT('Ctrl Pts',(1.41238735299022,0.883863978131697,12.7823964921449));
#56024=CARTESIAN_POINT('Ctrl Pts',(1.40042732984628,0.902694167579866,12.7839689646434));
#56025=CARTESIAN_POINT('Ctrl Pts',(1.35186641571567,0.97586113825294,12.7902134392875));
#56026=CARTESIAN_POINT('Ctrl Pts',(1.31245319359004,1.02825749797639,12.7949813437029));
#56027=CARTESIAN_POINT('Ctrl Pts',(1.1911489601694,1.17114793437916,12.8086256200138));
#56028=CARTESIAN_POINT('Ctrl Pts',(1.10225733378982,1.25517427220707,12.8174330566012));
#56029=CARTESIAN_POINT('Ctrl Pts',(0.988278330456608,1.34137994608991,12.8272627966982));
#56030=CARTESIAN_POINT('Ctrl Pts',(0.971345117600342,1.35369233940924,12.8286907243316));
#56031=CARTESIAN_POINT('Ctrl Pts',(0.943899110223326,1.37286848439712,12.8309548860188));
#56032=CARTESIAN_POINT('Ctrl Pts',(0.93353348679762,1.37993791516368,12.8317988673914));
#56033=CARTESIAN_POINT('Ctrl Pts',(0.914942723829558,1.39231159088029,12.833293229329));
#56034=CARTESIAN_POINT('Ctrl Pts',(0.906748949755013,1.39766165545498,12.8339453096561));
#56035=CARTESIAN_POINT('Ctrl Pts',(0.8894682065154,1.40872905666082,12.8353071348065));
#56036=CARTESIAN_POINT('Ctrl Pts',(0.880372128812226,1.41443139437494,12.8360163024898));
#56037=CARTESIAN_POINT('Ctrl Pts',(0.856182920587735,1.42927187315541,12.8378825522987));
#56038=CARTESIAN_POINT('Ctrl Pts',(0.840998397119315,1.43825902245204,12.8390341127294));
#56039=CARTESIAN_POINT('Ctrl Pts',(0.76197652369579,1.48334962765855,12.844930066255));
#56040=CARTESIAN_POINT('Ctrl Pts',(0.695944834037316,1.51545276559591,12.8495303518046));
#56041=CARTESIAN_POINT('Ctrl Pts',(0.537207197143363,1.5800551281359,12.8601082116231));
#56042=CARTESIAN_POINT('Ctrl Pts',(0.443328711433185,1.60892024035801,12.8660030087829));
#56043=CARTESIAN_POINT('Ctrl Pts',(0.321624669954097,1.63487351493144,12.8737223988559));
#56044=CARTESIAN_POINT('Ctrl Pts',(0.295662605808025,1.63976746736776,12.8753742495313));
#56045=CARTESIAN_POINT('Ctrl Pts',(0.237912932408908,1.64923748013971,12.8790810921117));
#56046=CARTESIAN_POINT('Ctrl Pts',(0.206088399131596,1.65351567395734,12.8811454363986));
#56047=CARTESIAN_POINT('Ctrl Pts',(0.164527922900877,1.65788431960283,12.8838924352525));
#56048=CARTESIAN_POINT('Ctrl Pts',(0.154884781049913,1.65881299370744,12.8845333804704));
#56049=CARTESIAN_POINT('Ctrl Pts',(0.139312011104854,1.66017574568347,12.8855749961719));
#56050=CARTESIAN_POINT('Ctrl Pts',(0.133387031678032,1.66066228956638,12.8859728275995));
#56051=CARTESIAN_POINT('Ctrl Pts',(0.121835508450726,1.66154865308232,12.8867516496581));
#56052=CARTESIAN_POINT('Ctrl Pts',(0.116209345184492,1.66195162448117,12.8871324660537));
#56053=CARTESIAN_POINT('Ctrl Pts',(0.102344652903931,1.66287393271677,12.8880744298977));
#56054=CARTESIAN_POINT('Ctrl Pts',(0.094104169108446,1.66336061704084,12.8886373318445));
#56055=CARTESIAN_POINT('Ctrl Pts',(0.0633597997430186,1.66494719775285,
12.890747975213));
#56056=CARTESIAN_POINT('Ctrl Pts',(0.0408390600815614,1.66565172952927,
12.8923150344996));
#56057=CARTESIAN_POINT('Ctrl Pts',(-0.0176901115778156,1.66629511057611,
12.8964307176475));
#56058=CARTESIAN_POINT('Ctrl Pts',(-0.0536938065023354,1.66552363755354,
12.8990046148275));
#56059=CARTESIAN_POINT('Ctrl Pts',(-0.162034491289828,1.65968573489037,
12.906828305595));
#56060=CARTESIAN_POINT('Ctrl Pts',(-0.234094610449637,1.6510637678514,12.9121341705021));
#56061=CARTESIAN_POINT('Ctrl Pts',(-0.395076733766986,1.6210486121683,12.924004206247));
#56062=CARTESIAN_POINT('Ctrl Pts',(-0.483275276334051,1.59697649060253,
12.930513595068));
#56063=CARTESIAN_POINT('Ctrl Pts',(-0.591086216962083,1.55779390330297,
12.9384086095892));
#56064=CARTESIAN_POINT('Ctrl Pts',(-0.612932587514291,1.54932840320655,
12.9400059079389));
#56065=CARTESIAN_POINT('Ctrl Pts',(-0.645771090704461,1.53580005992499,
12.9424042130378));
#56066=CARTESIAN_POINT('Ctrl Pts',(-0.656897835639443,1.53107392785202,
12.9432163723326));
#56067=CARTESIAN_POINT('Ctrl Pts',(-0.676871867716483,1.52233204185319,
12.9446737896956));
#56068=CARTESIAN_POINT('Ctrl Pts',(-0.685737240829575,1.51835925075639,
12.9453204709544));
#56069=CARTESIAN_POINT('Ctrl Pts',(-0.704684727462295,1.50966861481764,
12.9467024346316));
#56070=CARTESIAN_POINT('Ctrl Pts',(-0.714755375187231,1.50492679404536,
12.9474368576336));
#56071=CARTESIAN_POINT('Ctrl Pts',(-0.742330914489212,1.49160344755027,
12.9494481661858));
#56072=CARTESIAN_POINT('Ctrl Pts',(-0.759734233455017,1.48281488311805,
12.9507178551845));
#56073=CARTESIAN_POINT('Ctrl Pts',(-0.874977468800661,1.42205604085857,
12.9591369169189));
#56074=CARTESIAN_POINT('Ctrl Pts',(-0.967581614535266,1.36074208538991,
12.9659324284006));
#56075=CARTESIAN_POINT('Ctrl Pts',(-1.13625910694765,1.22307161813057,12.9792294424446));
#56076=CARTESIAN_POINT('Ctrl Pts',(-1.21238323939863,1.1476538812621,12.9857102706021));
#56077=CARTESIAN_POINT('Ctrl Pts',(-1.29015623642924,1.05416760272271,12.9936131451692));
#56078=CARTESIAN_POINT('Ctrl Pts',(-1.299414694512,1.04273384161376,12.9945779040289));
#56079=CARTESIAN_POINT('Ctrl Pts',(-1.31286032658278,1.02567194214856,12.9960174840741));
#56080=CARTESIAN_POINT('Ctrl Pts',(-1.31716561169085,1.0201372049804,12.9964844611958));
#56081=CARTESIAN_POINT('Ctrl Pts',(-1.32476907197542,1.01023406487874,12.9973203245247));
#56082=CARTESIAN_POINT('Ctrl Pts',(-1.32808084103939,1.00587635330449,12.9976882536763));
#56083=CARTESIAN_POINT('Ctrl Pts',(-1.3352707463399,0.996318279912363,12.9984956055479));
#56084=CARTESIAN_POINT('Ctrl Pts',(-1.33913994817879,0.991111636764372,
12.9989355909969));
#56085=CARTESIAN_POINT('Ctrl Pts',(-1.35019915862409,0.976046676796701,
13.0002088806265));
#56086=CARTESIAN_POINT('Ctrl Pts',(-1.3573112194442,0.966132038104315,13.0010471463176));
#56087=CARTESIAN_POINT('Ctrl Pts',(-1.37334739919323,0.943250071439848,
13.0029807794682));
#56088=CARTESIAN_POINT('Ctrl Pts',(-1.38219782330862,0.930232720082306,
13.004080083989));
#56089=CARTESIAN_POINT('Ctrl Pts',(-1.41140085906255,0.885943406134831,
13.0078128873333));
#56090=CARTESIAN_POINT('Ctrl Pts',(-1.4308861669804,0.854115057018459,13.0104830415073));
#56091=CARTESIAN_POINT('Ctrl Pts',(-1.49396270299068,0.7428577050065,13.0197138967315));
#56092=CARTESIAN_POINT('Ctrl Pts',(-1.53213819264634,0.660540752150257,
13.0263605310097));
#56093=CARTESIAN_POINT('Ctrl Pts',(-1.56343129955154,0.575533293200813,
13.0328805013286));
#56094=CARTESIAN_POINT('Origin',(0.,0.,11.));
#56095=CARTESIAN_POINT('',(-1.56343128722854,0.575533326676141,13.7334757494662));
#56096=CARTESIAN_POINT('',(-1.56343130308087,0.575533283613436,13.5398191707253));
#56097=CARTESIAN_POINT('',(-1.56343130033213,0.575533291080363,11.));
#56098=CARTESIAN_POINT('Ctrl Pts',(-1.56343130308087,0.575533283613436,
13.5398191707253));
#56099=CARTESIAN_POINT('Ctrl Pts',(-1.56078063958421,0.582733788610461,
13.539262439699));
#56100=CARTESIAN_POINT('Ctrl Pts',(-1.55808001184986,0.589916580831864,
13.5387050978713));
#56101=CARTESIAN_POINT('Ctrl Pts',(-1.51920569478185,0.691179829684495,
13.5308213929391));
#56102=CARTESIAN_POINT('Ctrl Pts',(-1.47461275565274,0.781816166493946,
13.5234617103585));
#56103=CARTESIAN_POINT('Ctrl Pts',(-1.4050123037459,0.895863785834677,13.5140118707061));
#56104=CARTESIAN_POINT('Ctrl Pts',(-1.3871047788544,0.92334829391982,13.5117168563318));
#56105=CARTESIAN_POINT('Ctrl Pts',(-1.35301290840937,0.97243994143396,13.5075859500054));
#56106=CARTESIAN_POINT('Ctrl Pts',(-1.33709294894636,0.994216255604684,
13.5057415119941));
#56107=CARTESIAN_POINT('Ctrl Pts',(-1.31288663661251,1.02569336596771,13.5030559264581));
#56108=CARTESIAN_POINT('Ctrl Pts',(-1.30500714666334,1.03570003590777,13.5021991455198));
#56109=CARTESIAN_POINT('Ctrl Pts',(-1.29087419197495,1.05323098385015,13.5006923770766));
#56110=CARTESIAN_POINT('Ctrl Pts',(-1.28466783429224,1.06079227344404,13.5000405536887));
#56111=CARTESIAN_POINT('Ctrl Pts',(-1.27150444843871,1.07654443136885,13.498678296485));
#56112=CARTESIAN_POINT('Ctrl Pts',(-1.2645340209572,1.08472355652462,13.4979684482144));
#56113=CARTESIAN_POINT('Ctrl Pts',(-1.24587774173042,1.10619065013814,13.4960981821036));
#56114=CARTESIAN_POINT('Ctrl Pts',(-1.23405829266994,1.11936109952817,13.4949433303307));
#56115=CARTESIAN_POINT('Ctrl Pts',(-1.17677516370477,1.18118147173559,13.4894820990634));
#56116=CARTESIAN_POINT('Ctrl Pts',(-1.12862917971982,1.22726817125945,13.4852918507597));
#56117=CARTESIAN_POINT('Ctrl Pts',(-0.967598779638467,1.36389662016979,
13.4722166900698));
#56118=CARTESIAN_POINT('Ctrl Pts',(-0.84565746427689,1.44267607924082,13.4636782140505));
#56119=CARTESIAN_POINT('Ctrl Pts',(-0.695280129621473,1.51414104592946,
13.4529846237284));
#56120=CARTESIAN_POINT('Ctrl Pts',(-0.675276858608457,1.52316729808642,
13.4515580273188));
#56121=CARTESIAN_POINT('Ctrl Pts',(-0.647587975310001,1.53500899270622,
13.4495698482882));
#56122=CARTESIAN_POINT('Ctrl Pts',(-0.640050249902359,1.53816724195143,
13.4490272581202));
#56123=CARTESIAN_POINT('Ctrl Pts',(-0.627286175390144,1.54340522601208,
13.4481056860776));
#56124=CARTESIAN_POINT('Ctrl Pts',(-0.622071845109108,1.54551423673817,
13.4477284311482));
#56125=CARTESIAN_POINT('Ctrl Pts',(-0.611985814380127,1.54953436488008,
13.4469970397734));
#56126=CARTESIAN_POINT('Ctrl Pts',(-0.607115649575051,1.55144899080622,
13.4466431449657));
#56127=CARTESIAN_POINT('Ctrl Pts',(-0.593782200643017,1.55661842456099,
13.4456724154139));
#56128=CARTESIAN_POINT('Ctrl Pts',(-0.58530138817499,1.55982707284114,13.4450529569165));
#56129=CARTESIAN_POINT('Ctrl Pts',(-0.551733935474446,1.57221476238125,
13.4425943311884));
#56130=CARTESIAN_POINT('Ctrl Pts',(-0.52645566784073,1.58085857356714,13.4407280152879));
#56131=CARTESIAN_POINT('Ctrl Pts',(-0.469636774464721,1.59877375708414,
13.4365163684573));
#56132=CARTESIAN_POINT('Ctrl Pts',(-0.438007177312401,1.60772687718784,
13.4341607017602));
#56133=CARTESIAN_POINT('Ctrl Pts',(-0.31086969184172,1.6396844174034,13.4246958855022));
#56134=CARTESIAN_POINT('Ctrl Pts',(-0.213666309556907,1.65515960133083,
13.417482567313));
#56135=CARTESIAN_POINT('Ctrl Pts',(-0.0425254251703389,1.66707019277201,
13.4051815671385));
#56136=CARTESIAN_POINT('Ctrl Pts',(0.0308792862739422,1.66732737994433,
13.4000282438992));
#56137=CARTESIAN_POINT('Ctrl Pts',(0.121678815063038,1.66164421266878,13.3938193383965));
#56138=CARTESIAN_POINT('Ctrl Pts',(0.139267835052863,1.66026255008328,13.3926240379113));
#56139=CARTESIAN_POINT('Ctrl Pts',(0.167519056633602,1.65759120286808,13.3907154676102));
#56140=CARTESIAN_POINT('Ctrl Pts',(0.178196112571544,1.65647740248834,13.3899967576915));
#56141=CARTESIAN_POINT('Ctrl Pts',(0.198583706422165,1.65415121918064,13.3886291139528));
#56142=CARTESIAN_POINT('Ctrl Pts',(0.208295746665879,1.65295633132395,13.387979661136));
#56143=CARTESIAN_POINT('Ctrl Pts',(0.230434731083972,1.65003431172002,13.3865036092579));
#56144=CARTESIAN_POINT('Ctrl Pts',(0.24285392001679,1.64825222068555,13.3856787722332));
#56145=CARTESIAN_POINT('Ctrl Pts',(0.275938340243625,1.64312271002202,13.3834890769573));
#56146=CARTESIAN_POINT('Ctrl Pts',(0.296563008300342,1.63952574011155,13.3821320492411));
#56147=CARTESIAN_POINT('Ctrl Pts',(0.436838295541776,1.61232775207546,13.3729450315476));
#56148=CARTESIAN_POINT('Ctrl Pts',(0.553652594887798,1.57603970122121,13.3655423060756));
#56149=CARTESIAN_POINT('Ctrl Pts',(0.725525139122892,1.50115316127148,13.3540849441));
#56150=CARTESIAN_POINT('Ctrl Pts',(0.783981987973894,1.47146815935395,13.350069025891));
#56151=CARTESIAN_POINT('Ctrl Pts',(0.859793329183877,1.42716816105914,13.3445102798992));
#56152=CARTESIAN_POINT('Ctrl Pts',(0.878822846214977,1.41552952457611,13.3430834406582));
#56153=CARTESIAN_POINT('Ctrl Pts',(0.911024586985196,1.3949350095035,13.3406040932607));
#56154=CARTESIAN_POINT('Ctrl Pts',(0.92431291500871,1.38616559923526,13.3395614363744));
#56155=CARTESIAN_POINT('Ctrl Pts',(0.943432967883764,1.37315047126158,13.3380293813489));
#56156=CARTESIAN_POINT('Ctrl Pts',(0.949366473040456,1.36905488446975,13.3375494046891));
#56157=CARTESIAN_POINT('Ctrl Pts',(0.959762963440568,1.3617786485229,13.3367000287527));
#56158=CARTESIAN_POINT('Ctrl Pts',(0.96423711734629,1.35861429913119,13.3363317225267));
#56159=CARTESIAN_POINT('Ctrl Pts',(0.973927715458534,1.35168863314032,13.3355278588063));
#56160=CARTESIAN_POINT('Ctrl Pts',(0.979137940286179,1.34791922840272,13.335091778725));
#56161=CARTESIAN_POINT('Ctrl Pts',(0.993687959381296,1.33726395556338,13.3338633695121));
#56162=CARTESIAN_POINT('Ctrl Pts',(1.00297761217376,1.33031069233537,13.3330666976623));
#56163=CARTESIAN_POINT('Ctrl Pts',(1.07338986423151,1.27645070864256,13.3269376250523));
#56164=CARTESIAN_POINT('Ctrl Pts',(1.13125854920797,1.22545649252868,13.3213776218073));
#56165=CARTESIAN_POINT('Ctrl Pts',(1.22567950514986,1.12984698623709,13.3116102235553));
#56166=CARTESIAN_POINT('Ctrl Pts',(1.26384165218415,1.08699080449051,13.3074255594243));
#56167=CARTESIAN_POINT('Ctrl Pts',(1.35140611942951,0.977795346120671,13.2973117178933));
#56168=CARTESIAN_POINT('Ctrl Pts',(1.3982336997387,0.909575912711863,13.2914448819633));
#56169=CARTESIAN_POINT('Ctrl Pts',(1.45128979341069,0.818434207668401,13.2841948610304));
#56170=CARTESIAN_POINT('Ctrl Pts',(1.4623630391522,0.798480461866163,13.2826405325659));
#56171=CARTESIAN_POINT('Ctrl Pts',(1.47854286792671,0.767858434776805,13.2803034588139));
#56172=CARTESIAN_POINT('Ctrl Pts',(1.48395119894103,0.757353576465818,13.2795101506542));
#56173=CARTESIAN_POINT('Ctrl Pts',(1.49317318631019,0.738963148905957,13.2781356308063));
#56174=CARTESIAN_POINT('Ctrl Pts',(1.49703719751134,0.731103504334115,13.2775526772985));
#56175=CARTESIAN_POINT('Ctrl Pts',(1.50561210861306,0.713308538150928,13.2762427012624));
#56176=CARTESIAN_POINT('Ctrl Pts',(1.51028702174477,0.703356249639429,13.2755169458164));
#56177=CARTESIAN_POINT('Ctrl Pts',(1.52271164583514,0.676210677261127,13.2735554594478));
#56178=CARTESIAN_POINT('Ctrl Pts',(1.53026865779012,0.658930586916578,13.2723263291607));
#56179=CARTESIAN_POINT('Ctrl Pts',(1.57568503437986,0.550082066185779,13.2646973156984));
#56180=CARTESIAN_POINT('Ctrl Pts',(1.60560791153685,0.455412450130569,13.2585747852756));
#56181=CARTESIAN_POINT('Ctrl Pts',(1.64233484059112,0.288800724711676,13.2481384938311));
#56182=CARTESIAN_POINT('Ctrl Pts',(1.65321572748002,0.218051881689388,13.2438020376228));
#56183=CARTESIAN_POINT('Ctrl Pts',(1.66277342371212,0.11002480217375,13.2370682061555));
#56184=CARTESIAN_POINT('Ctrl Pts',(1.66480415103102,0.0731279813369949,
13.2347479146914));
#56185=CARTESIAN_POINT('Ctrl Pts',(1.66594652090965,0.0205613540279227,
13.2313757891008));
#56186=CARTESIAN_POINT('Ctrl Pts',(1.66606611797867,0.00492259779151108,
13.2303641947194));
#56187=CARTESIAN_POINT('Ctrl Pts',(1.66588746166219,-0.0228551018100175,
13.2285488546726));
#56188=CARTESIAN_POINT('Ctrl Pts',(1.6656766834191,-0.0349936539018341,
13.2277492798936));
#56189=CARTESIAN_POINT('Ctrl Pts',(1.66515013662737,-0.0535997655218569,
13.2265125469586));
#56190=CARTESIAN_POINT('Ctrl Pts',(1.66492928284331,-0.0600698923750112,
13.2260804167628));
#56191=CARTESIAN_POINT('Ctrl Pts',(1.66445207230846,-0.0720088335210612,
13.2252789464481));
#56192=CARTESIAN_POINT('Ctrl Pts',(1.66420646245664,-0.0774778701527156,
13.2249101994056));
#56193=CARTESIAN_POINT('Ctrl Pts',(1.6635839609758,-0.0899655931361387,
13.2240645887955));
#56194=CARTESIAN_POINT('Ctrl Pts',(1.66318960528338,-0.0969831714899934,
13.2235867916918));
#56195=CARTESIAN_POINT('Ctrl Pts',(1.66179323419462,-0.119308791606604,
13.2220589024835));
#56196=CARTESIAN_POINT('Ctrl Pts',(1.66062421189745,-0.134605074720966,
13.221000351478));
#56197=CARTESIAN_POINT('Ctrl Pts',(1.64759505101927,-0.278841944485463,
13.2109212176064));
#56198=CARTESIAN_POINT('Ctrl Pts',(1.62095247647327,-0.405996383736341,
13.2013389509523));
#56199=CARTESIAN_POINT('Ctrl Pts',(1.55143803924907,-0.613688483427946,
13.1855174709197));
#56200=CARTESIAN_POINT('Ctrl Pts',(1.51621567986653,-0.696181189724852,
13.1791746308323));
#56201=CARTESIAN_POINT('Ctrl Pts',(1.46595758784083,-0.791746943407482,
13.1717969717608));
#56202=CARTESIAN_POINT('Ctrl Pts',(1.45711947032206,-0.807897127205963,
13.1705485992364));
#56203=CARTESIAN_POINT('Ctrl Pts',(1.44262523044902,-0.833371005094781,
13.1685762425694));
#56204=CARTESIAN_POINT('Ctrl Pts',(1.43714235200819,-0.842790992770211,
13.167846149872));
#56205=CARTESIAN_POINT('Ctrl Pts',(1.42658151334173,-0.860532508537247,
13.1664694336762));
#56206=CARTESIAN_POINT('Ctrl Pts',(1.42152221475058,-0.868864553497879,
13.1658221707996));
#56207=CARTESIAN_POINT('Ctrl Pts',(1.40983576291534,-0.887735371601575,
13.1643543181588));
#56208=CARTESIAN_POINT('Ctrl Pts',(1.40316297802466,-0.898245311427428,
13.1635354435235));
#56209=CARTESIAN_POINT('Ctrl Pts',(1.38212838401984,-0.930569281940887,
13.1610117372549));
#56210=CARTESIAN_POINT('Ctrl Pts',(1.36737058064036,-0.952121774673777,
13.1593216345085));
#56211=CARTESIAN_POINT('Ctrl Pts',(1.2742265167525,-1.08151523042013,13.149107220142));
#56212=CARTESIAN_POINT('Ctrl Pts',(1.18363875495021,-1.17997054149023,13.1410900669583));
#56213=CARTESIAN_POINT('Ctrl Pts',(1.02747062876932,-1.31341441604048,13.12849043018));
#56214=CARTESIAN_POINT('Ctrl Pts',(0.969686058859638,-1.3566354993666,13.1240238088173));
#56215=CARTESIAN_POINT('Ctrl Pts',(0.896016987663439,-1.40462114582404,
13.1183202779933));
#56216=CARTESIAN_POINT('Ctrl Pts',(0.882619619151807,-1.413078047567,13.1172826106798));
#56217=CARTESIAN_POINT('Ctrl Pts',(0.862965249064118,-1.42509605220349,
13.1157565627056));
#56218=CARTESIAN_POINT('Ctrl Pts',(0.856802088325468,-1.42880997888933,
13.1152775004625));
#56219=CARTESIAN_POINT('Ctrl Pts',(0.845946506869366,-1.4352560711809,13.1144324174677));
#56220=CARTESIAN_POINT('Ctrl Pts',(0.841264498009107,-1.43800539828144,
13.1140675074197));
#56221=CARTESIAN_POINT('Ctrl Pts',(0.831017597381068,-1.4439553185029,13.1132678569433));
#56222=CARTESIAN_POINT('Ctrl Pts',(0.82544770846477,-1.44714660145552,13.1128325725695));
#56223=CARTESIAN_POINT('Ctrl Pts',(0.809802895970906,-1.45599063454264,
13.1116085050967));
#56224=CARTESIAN_POINT('Ctrl Pts',(0.799687643343507,-1.4615707689722,13.1108154259741));
#56225=CARTESIAN_POINT('Ctrl Pts',(0.728319681671741,-1.49997866525846,
13.1052126204907));
#56226=CARTESIAN_POINT('Ctrl Pts',(0.665129678011054,-1.52904738028681,
13.1002173113484));
#56227=CARTESIAN_POINT('Ctrl Pts',(0.585077707710549,-1.55997018917972,
13.0939897622467));
#56228=CARTESIAN_POINT('Ctrl Pts',(0.569752010605036,-1.56563263697475,
13.0928017591634));
#56229=CARTESIAN_POINT('Ctrl Pts',(0.499829501062926,-1.59030452887988,
13.0874060885637));
#56230=CARTESIAN_POINT('Ctrl Pts',(0.444347214891184,-1.60669039069399,
13.0831938179496));
#56231=CARTESIAN_POINT('Ctrl Pts',(0.308650461485002,-1.63919779272084,
13.0731468346497));
#56232=CARTESIAN_POINT('Ctrl Pts',(0.227874294767913,-1.65236541209983,
13.0673792546634));
#56233=CARTESIAN_POINT('Ctrl Pts',(0.128432718112406,-1.66114058803395,
13.0605616511355));
#56234=CARTESIAN_POINT('Ctrl Pts',(0.110393852130142,-1.6624368434493,13.0593357655432));
#56235=CARTESIAN_POINT('Ctrl Pts',(0.0815240961288447,-1.66403939166931,
13.0573904249872));
#56236=CARTESIAN_POINT('Ctrl Pts',(0.0707055612236025,-1.66453417161388,
13.0566651483949));
#56237=CARTESIAN_POINT('Ctrl Pts',(0.0501273633291889,-1.66527431315372,
13.0552923739536));
#56238=CARTESIAN_POINT('Ctrl Pts',(0.040368912603012,-1.6655394466729,13.0546442869696));
#56239=CARTESIAN_POINT('Ctrl Pts',(0.0180369109477417,-1.66594980969968,
13.0531675064122));
#56240=CARTESIAN_POINT('Ctrl Pts',(0.00546281731895583,-1.66603849614875,
13.0523406080641));
#56241=CARTESIAN_POINT('Ctrl Pts',(-0.0276690126860467,-1.66589707070504,
13.0501730990491));
#56242=CARTESIAN_POINT('Ctrl Pts',(-0.0482239536893625,-1.66542881389035,
13.048839871726));
#56243=CARTESIAN_POINT('Ctrl Pts',(-0.219716227839807,-1.65834427223022,
13.0377983868978));
#56244=CARTESIAN_POINT('Ctrl Pts',(-0.36910939800944,-1.6316068049493,13.0287900245318));
#56245=CARTESIAN_POINT('Ctrl Pts',(-0.57118261835091,-1.56622616859821,
13.0156970738585));
#56246=CARTESIAN_POINT('Ctrl Pts',(-0.628416089250399,-1.54415206187481,
13.0118665903021));
#56247=CARTESIAN_POINT('Ctrl Pts',(-0.697709480844861,-1.51293552264221,
13.0069258374521));
#56248=CARTESIAN_POINT('Ctrl Pts',(-0.71104112904732,-1.50671592935183,
13.0059607929047));
#56249=CARTESIAN_POINT('Ctrl Pts',(-0.730579569469668,-1.49728364048205,
13.0045224355632));
#56250=CARTESIAN_POINT('Ctrl Pts',(-0.736851728182095,-1.49420692465061,
13.0040570025248));
#56251=CARTESIAN_POINT('Ctrl Pts',(-0.747524862531159,-1.48888783179757,
13.003258344186));
#56252=CARTESIAN_POINT('Ctrl Pts',(-0.751935511858444,-1.48666518786077,
13.0029263384185));
#56253=CARTESIAN_POINT('Ctrl Pts',(-0.762009933595512,-1.48153211502753,
13.0021634291434));
#56254=CARTESIAN_POINT('Ctrl Pts',(-0.767666821414207,-1.47860887142577,
13.0017317499293));
#56255=CARTESIAN_POINT('Ctrl Pts',(-0.783333953774059,-1.47039861089681,
13.0005272852728));
#56256=CARTESIAN_POINT('Ctrl Pts',(-0.793307055207248,-1.46504199827002,
12.9997504118401));
#56257=CARTESIAN_POINT('Ctrl Pts',(-0.855947731648896,-1.43057018268568,
12.9948100204932));
#56258=CARTESIAN_POINT('Ctrl Pts',(-0.907054729155208,-1.39872359923603,
12.9905067810779));
#56259=CARTESIAN_POINT('Ctrl Pts',(-1.08004453067157,-1.277454402411,12.9752226578679));
#56260=CARTESIAN_POINT('Ctrl Pts',(-1.19142423807187,-1.17427059935779,
12.9641259278032));
#56261=CARTESIAN_POINT('Ctrl Pts',(-1.30443208684846,-1.03669465385404,
12.9518253194119));
#56262=CARTESIAN_POINT('Ctrl Pts',(-1.32099318626975,-1.01550776564639,
12.9499872596514));
#56263=CARTESIAN_POINT('Ctrl Pts',(-1.34454598337578,-0.983824474894265,
12.9473181119125));
#56264=CARTESIAN_POINT('Ctrl Pts',(-1.35194230553156,-0.973635720600104,
12.9464714040762));
#56265=CARTESIAN_POINT('Ctrl Pts',(-1.36486839297745,-0.955398135602065,
12.9449759714982));
#56266=CARTESIAN_POINT('Ctrl Pts',(-1.37044415117428,-0.947382796522105,
12.9443255043583));
#56267=CARTESIAN_POINT('Ctrl Pts',(-1.38205020898995,-0.930381809153599,
12.9429597681231));
#56268=CARTESIAN_POINT('Ctrl Pts',(-1.38806409381718,-0.921385463170396,
12.9422451401098));
#56269=CARTESIAN_POINT('Ctrl Pts',(-1.40387118522243,-0.897233123533381,
12.9403474884827));
#56270=CARTESIAN_POINT('Ctrl Pts',(-1.41350671485392,-0.881975278032113,
12.9391703338852));
#56271=CARTESIAN_POINT('Ctrl Pts',(-1.46040253022888,-0.804972583718597,
12.9333313256575));
#56272=CARTESIAN_POINT('Ctrl Pts',(-1.49387638226336,-0.741007171254946,
12.928807563864));
#56273=CARTESIAN_POINT('Ctrl Pts',(-1.56867733661043,-0.572239445837458,
12.9174113369234));
#56274=CARTESIAN_POINT('Ctrl Pts',(-1.60371910744669,-0.4650685563014,12.910681293389));
#56275=CARTESIAN_POINT('Ctrl Pts',(-1.63392286958697,-0.32665739931845,
12.9018055102691));
#56276=CARTESIAN_POINT('Ctrl Pts',(-1.63939785886919,-0.297965539809874,
12.8999547654432));
#56277=CARTESIAN_POINT('Ctrl Pts',(-1.64725312081612,-0.249980647800218,
12.8968196084319));
#56278=CARTESIAN_POINT('Ctrl Pts',(-1.6500550709274,-0.230762543971044,
12.8955533950085));
#56279=CARTESIAN_POINT('Ctrl Pts',(-1.65351021530464,-0.203766457521889,
12.8937543841654));
#56280=CARTESIAN_POINT('Ctrl Pts',(-1.65444578406096,-0.196025363012954,
12.8932361856761));
#56281=CARTESIAN_POINT('Ctrl Pts',(-1.6559551224938,-0.182755378027296,
12.8923434403922));
#56282=CARTESIAN_POINT('Ctrl Pts',(-1.65655563773657,-0.177229552129271,
12.891970366896));
#56283=CARTESIAN_POINT('Ctrl Pts',(-1.6577585841788,-0.165619608456608,
12.8911835975408));
#56284=CARTESIAN_POINT('Ctrl Pts',(-1.65835518725454,-0.159535099590306,
12.89076960832));
#56285=CARTESIAN_POINT('Ctrl Pts',(-1.65988156014858,-0.143033515998585,
12.8896425915346));
#56286=CARTESIAN_POINT('Ctrl Pts',(-1.66074673008251,-0.132610953280565,
12.8889261699202));
#56287=CARTESIAN_POINT('Ctrl Pts',(-1.66448157853897,-0.0818216500600575,
12.8854149250593));
#56288=CARTESIAN_POINT('Ctrl Pts',(-1.66597766395643,-0.0413707825729691,
12.8825568699521));
#56289=CARTESIAN_POINT('Ctrl Pts',(-1.66604677910934,0.085236454430287,
12.8734955076404));
#56290=CARTESIAN_POINT('Ctrl Pts',(-1.65941215201514,0.171254168355328,
12.8671784700656));
#56291=CARTESIAN_POINT('Ctrl Pts',(-1.63083730655712,0.354732671185672,
12.8537186085672));
#56292=CARTESIAN_POINT('Ctrl Pts',(-1.60673147312273,0.451537197537825,
12.8466328130717));
#56293=CARTESIAN_POINT('Ctrl Pts',(-1.57065155998457,0.555627367079107,
12.8391004744649));
#56294=CARTESIAN_POINT('Ctrl Pts',(-1.56708883221216,0.565597636766373,
12.8383796912937));
#56295=CARTESIAN_POINT('Ctrl Pts',(-1.56343130043543,0.575533290799732,
12.8376620384731));
#56296=CARTESIAN_POINT('',(-1.6659993171282,-0.00113364010792655,13.0724915839951));
#56297=CARTESIAN_POINT('Ctrl Pts',(-1.56343129955154,0.575533293200813,
13.0328805013286));
#56298=CARTESIAN_POINT('Ctrl Pts',(-1.56437182275508,0.57297836991185,13.0330764608858));
#56299=CARTESIAN_POINT('Ctrl Pts',(-1.56530612886598,0.57042101700076,13.0332723164847));
#56300=CARTESIAN_POINT('Ctrl Pts',(-1.59042310597543,0.501145171435164,
13.0385699050769));
#56301=CARTESIAN_POINT('Ctrl Pts',(-1.61032706365741,0.432944842177226,
13.0435817436763));
#56302=CARTESIAN_POINT('Ctrl Pts',(-1.63017709847875,0.344204408370925,
13.0498276822958));
#56303=CARTESIAN_POINT('Ctrl Pts',(-1.63418232908532,0.32465708416631,13.0511871468137));
#56304=CARTESIAN_POINT('Ctrl Pts',(-1.64010568145126,0.292853317024579,
13.0533733767878));
#56305=CARTESIAN_POINT('Ctrl Pts',(-1.64223966793376,0.28063962497421,13.0542068841866));
#56306=CARTESIAN_POINT('Ctrl Pts',(-1.64580673800576,0.258787745058411,
13.0556876428351));
#56307=CARTESIAN_POINT('Ctrl Pts',(-1.64729196723902,0.249158779600448,
13.0563365141801));
#56308=CARTESIAN_POINT('Ctrl Pts',(-1.65000269526167,0.230499751549097,
13.0575871235083));
#56309=CARTESIAN_POINT('Ctrl Pts',(-1.65123873696157,0.221471598543318,
13.0581891717326));
#56310=CARTESIAN_POINT('Ctrl Pts',(-1.65377085400944,0.201775694529071,
13.059496189771));
#56311=CARTESIAN_POINT('Ctrl Pts',(-1.65503792035683,0.191104577514267,
13.0602002335343));
#56312=CARTESIAN_POINT('Ctrl Pts',(-1.65874178780854,0.157104509034263,
13.0624311029811));
#56313=CARTESIAN_POINT('Ctrl Pts',(-1.66078929393574,0.133735383052599,
13.0639459438566));
#56314=CARTESIAN_POINT('Ctrl Pts',(-1.6648052270699,0.0732272208265782,
13.0678274033941));
#56315=CARTESIAN_POINT('Ctrl Pts',(-1.66602496239537,0.0360513616570116,
13.0701723343068));
#56316=CARTESIAN_POINT('Ctrl Pts',(-1.66599961292089,-0.00113567048074876,
13.0724922261414));
#56317=CARTESIAN_POINT('Ctrl Pts',(-1.66599961432537,-0.0011336082690304,
13.0724920974914));
#56318=CARTESIAN_POINT('Ctrl Pts',(-1.66594641663436,-0.0793152298434674,
13.0773694154298));
#56319=CARTESIAN_POINT('Ctrl Pts',(-1.66038991779439,-0.157401370556992,
13.0821227248742));
#56320=CARTESIAN_POINT('Ctrl Pts',(-1.63597659975319,-0.32888564353002,
13.0927072487401));
#56321=CARTESIAN_POINT('Ctrl Pts',(-1.61456184732864,-0.421627816383002,
13.0985306909447));
#56322=CARTESIAN_POINT('Ctrl Pts',(-1.58171934603026,-0.523317043441458,
13.1055184031541));
#56323=CARTESIAN_POINT('Ctrl Pts',(-1.57795185575317,-0.534569676197079,
13.1063003063003));
#56324=CARTESIAN_POINT('Ctrl Pts',(-1.57196250313768,-0.551843331990107,
13.1075153789434));
#56325=CARTESIAN_POINT('Ctrl Pts',(-1.56982542374298,-0.557893636686304,
13.1079437904974));
#56326=CARTESIAN_POINT('Ctrl Pts',(-1.56579761599185,-0.569090402467872,
13.1087421159837));
#56327=CARTESIAN_POINT('Ctrl Pts',(-1.56391637035455,-0.574240057585588,
13.1091114783297));
#56328=CARTESIAN_POINT('Ctrl Pts',(-1.55953709223092,-0.586046595080044,
13.1099633071619));
#56329=CARTESIAN_POINT('Ctrl Pts',(-1.5570218352854,-0.592696847852759,
13.1104467604043));
#56330=CARTESIAN_POINT('Ctrl Pts',(-1.54899056781344,-0.613527281740871,
13.1119720894485));
#56331=CARTESIAN_POINT('Ctrl Pts',(-1.54332299985029,-0.627647657641964,
13.1130221764799));
#56332=CARTESIAN_POINT('Ctrl Pts',(-1.49876753404505,-0.734401104769392,
13.1210737566866));
#56333=CARTESIAN_POINT('Ctrl Pts',(-1.45176845576423,-0.823416107200453,
13.1284238402932));
#56334=CARTESIAN_POINT('Ctrl Pts',(-1.35399540663144,-0.973907586420926,
13.1414783635447));
#56335=CARTESIAN_POINT('Ctrl Pts',(-1.30628361340923,-1.03702701586896,
13.1471857940558));
#56336=CARTESIAN_POINT('Ctrl Pts',(-1.2341514856595,-1.11953569386178,13.1548972205387));
#56337=CARTESIAN_POINT('Ctrl Pts',(-1.21340561366253,-1.14198821286013,
13.1570252923463));
#56338=CARTESIAN_POINT('Ctrl Pts',(-1.17577701945939,-1.18052834702326,
13.1607315374277));
#56339=CARTESIAN_POINT('Ctrl Pts',(-1.1591529016014,-1.19685564022498,13.16231977149));
#56340=CARTESIAN_POINT('Ctrl Pts',(-1.13369744131278,-1.22082850347254,
13.1646806177124));
#56341=CARTESIAN_POINT('Ctrl Pts',(-1.12511988253612,-1.22873812721237,
13.1654645016534));
#56342=CARTESIAN_POINT('Ctrl Pts',(-1.10936568983615,-1.24296223464047,
13.1668835715654));
#56343=CARTESIAN_POINT('Ctrl Pts',(-1.10221652132255,-1.24930624635725,
13.1675199867346));
#56344=CARTESIAN_POINT('Ctrl Pts',(-1.08672728158303,-1.26281458867568,
13.1688829519083));
#56345=CARTESIAN_POINT('Ctrl Pts',(-1.07837005149802,-1.26995862597754,
13.1696086435282));
#56346=CARTESIAN_POINT('Ctrl Pts',(-1.05549225782594,-1.28912663682244,
13.1715696467484));
#56347=CARTESIAN_POINT('Ctrl Pts',(-1.04083706187644,-1.30098795138861,
13.1727983638934));
#56348=CARTESIAN_POINT('Ctrl Pts',(-0.949119568113573,-1.37267827943915,
13.1803283512919));
#56349=CARTESIAN_POINT('Ctrl Pts',(-0.867123123995699,-1.42589433654383,
13.186361681104));
#56350=CARTESIAN_POINT('Ctrl Pts',(-0.701277990085902,-1.51390102374039,
13.1978497701251));
#56351=CARTESIAN_POINT('Ctrl Pts',(-0.618330773170805,-1.54962964597898,
13.2032987686595));
#56352=CARTESIAN_POINT('Ctrl Pts',(-0.507857656181761,-1.58692645798029,
13.2106322252125));
#56353=CARTESIAN_POINT('Ctrl Pts',(-0.482612029858826,-1.59478539530338,
13.2123135892961));
#56354=CARTESIAN_POINT('Ctrl Pts',(-0.439822678907821,-1.60699665786356,
13.2151891066286));
#56355=CARTESIAN_POINT('Ctrl Pts',(-0.422375198756701,-1.61167036761957,
13.216368704717));
#56356=CARTESIAN_POINT('Ctrl Pts',(-0.397503724534727,-1.61790118319616,
13.2180647897242));
#56357=CARTESIAN_POINT('Ctrl Pts',(-0.390139073065968,-1.61969285599178,
13.2185688141468));
#56358=CARTESIAN_POINT('Ctrl Pts',(-0.377385245666111,-1.62270357860465,
13.2194451797666));
#56359=CARTESIAN_POINT('Ctrl Pts',(-0.372001805314126,-1.6239461763282,
13.2198161837269));
#56360=CARTESIAN_POINT('Ctrl Pts',(-0.36054868794128,-1.62652982756921,
13.2206079284222));
#56361=CARTESIAN_POINT('Ctrl Pts',(-0.35447775569873,-1.62786367791967,
13.2210290323115));
#56362=CARTESIAN_POINT('Ctrl Pts',(-0.337714440099959,-1.63144854396684,
13.2221954617577));
#56363=CARTESIAN_POINT('Ctrl Pts',(-0.327007382752697,-1.63362833913063,
13.2229445781537));
#56364=CARTESIAN_POINT('Ctrl Pts',(-0.269445461659474,-1.6447585322237,
13.2269910443427));
#56365=CARTESIAN_POINT('Ctrl Pts',(-0.222247987086075,-1.65179793529914,
13.2303763251464));
#56366=CARTESIAN_POINT('Ctrl Pts',(-0.0714595543652354,-1.66770848083152,
13.2412797687857));
#56367=CARTESIAN_POINT('Ctrl Pts',(0.0326943170026807,-1.66891899136661,
13.2489255994165));
#56368=CARTESIAN_POINT('Ctrl Pts',(0.211723165289117,-1.65422441558984,
13.2618217550684));
#56369=CARTESIAN_POINT('Ctrl Pts',(0.286659223639609,-1.64289821350859,
13.2671481186679));
#56370=CARTESIAN_POINT('Ctrl Pts',(0.377930991826556,-1.62266453672199,
13.2735297012681));
#56371=CARTESIAN_POINT('Ctrl Pts',(0.395224816857861,-1.6185392858934,13.2747343954035));
#56372=CARTESIAN_POINT('Ctrl Pts',(0.422878856893835,-1.61147303326979,
13.2766542861866));
#56373=CARTESIAN_POINT('Ctrl Pts',(0.433281949989266,-1.60870712865462,
13.2773750388266));
#56374=CARTESIAN_POINT('Ctrl Pts',(0.453082494615455,-1.60323668230582,
13.2787442899798));
#56375=CARTESIAN_POINT('Ctrl Pts',(0.462484329673286,-1.60054986119791,
13.2793933291659));
#56376=CARTESIAN_POINT('Ctrl Pts',(0.483840697693467,-1.59424282321754,
13.2808653592859));
#56377=CARTESIAN_POINT('Ctrl Pts',(0.495779358229588,-1.59057060271246,
13.281686623469));
#56378=CARTESIAN_POINT('Ctrl Pts',(0.527425156434536,-1.58044571696831,
13.2838600152122));
#56379=CARTESIAN_POINT('Ctrl Pts',(0.547055417135793,-1.57375868270628,
13.2852045010952));
#56380=CARTESIAN_POINT('Ctrl Pts',(0.683914761284068,-1.52426725944938,
13.2945642432359));
#56381=CARTESIAN_POINT('Ctrl Pts',(0.796134499740034,-1.4687762973108,13.3021284080007));
#56382=CARTESIAN_POINT('Ctrl Pts',(0.977395699649095,-1.35221265081053,
13.3153035585825));
#56383=CARTESIAN_POINT('Ctrl Pts',(1.04953485736196,-1.29701711762812,13.3208742210172));
#56384=CARTESIAN_POINT('Ctrl Pts',(1.12610108313259,-1.22784729175888,13.3276119279827));
#56385=CARTESIAN_POINT('Ctrl Pts',(1.13529241728116,-1.21935381476108,13.3284356522641));
#56386=CARTESIAN_POINT('Ctrl Pts',(1.14914841703908,-1.20625737012636,13.3297019776696));
#56387=CARTESIAN_POINT('Ctrl Pts',(1.15388328721975,-1.20172887257747,13.3301391713918));
#56388=CARTESIAN_POINT('Ctrl Pts',(1.16251998067545,-1.19337051496657,13.3309451565939));
#56389=CARTESIAN_POINT('Ctrl Pts',(1.16642981393031,-1.18954923302104,13.3313132998701));
#56390=CARTESIAN_POINT('Ctrl Pts',(1.17533394019365,-1.18076066362978,13.332159203262));
#56391=CARTESIAN_POINT('Ctrl Pts',(1.18031556950598,-1.17578091819978,13.3326379101307));
#56392=CARTESIAN_POINT('Ctrl Pts',(1.19581773468374,-1.16008681796706,13.3341443051606));
#56393=CARTESIAN_POINT('Ctrl Pts',(1.20622474609754,-1.14926206866399,13.335180009024));
#56394=CARTESIAN_POINT('Ctrl Pts',(1.28782784918856,-1.06205399162405,13.3434875419961));
#56395=CARTESIAN_POINT('Ctrl Pts',(1.35183997685693,-0.97927749833731,13.3511381568114));
#56396=CARTESIAN_POINT('Ctrl Pts',(1.46826907879617,-0.795345781820444,
13.366965950129));
#56397=CARTESIAN_POINT('Ctrl Pts',(1.51894816544301,-0.693681763120602,
13.3750832464998));
#56398=CARTESIAN_POINT('Ctrl Pts',(1.56575804935059,-0.569502907082649,
13.3841639609022));
#56399=CARTESIAN_POINT('Ctrl Pts',(1.57227922068042,-0.551243990973118,
13.3854800678179));
#56400=CARTESIAN_POINT('Ctrl Pts',(1.58203330260813,-0.522350468616721,
13.3875336947073));
#56401=CARTESIAN_POINT('Ctrl Pts',(1.58548088521564,-0.511790734176277,
13.3882782204302));
#56402=CARTESIAN_POINT('Ctrl Pts',(1.59174590795364,-0.491930263128515,
13.389667540571));
#56403=CARTESIAN_POINT('Ctrl Pts',(1.59458806627149,-0.48263788186675,13.3903131198856));
#56404=CARTESIAN_POINT('Ctrl Pts',(1.60079240038472,-0.461699690150318,
13.3917580536405));
#56405=CARTESIAN_POINT('Ctrl Pts',(1.60410913329456,-0.450040903094354,
13.392555902592));
#56406=CARTESIAN_POINT('Ctrl Pts',(1.6135034708557,-0.415594415919144,13.3948942789194));
#56407=CARTESIAN_POINT('Ctrl Pts',(1.61922496018563,-0.392712091490457,
13.3964233609263));
#56408=CARTESIAN_POINT('Ctrl Pts',(1.64738569855396,-0.268979061725007,
13.4045756307217));
#56409=CARTESIAN_POINT('Ctrl Pts',(1.66089396345492,-0.166324894291564,
13.4109092970689));
#56410=CARTESIAN_POINT('Ctrl Pts',(1.66779110162462,0.0157310073905968,
13.4220358017062));
#56411=CARTESIAN_POINT('Ctrl Pts',(1.66517752952499,0.0946397567061671,
13.4268299820002));
#56412=CARTESIAN_POINT('Ctrl Pts',(1.65442138496804,0.197625694297063,13.4333596480732));
#56413=CARTESIAN_POINT('Ctrl Pts',(1.65130989158162,0.222129572903168,13.4349341376021));
#56414=CARTESIAN_POINT('Ctrl Pts',(1.6451128113114,0.263543036510313,13.4376442198349));
#56415=CARTESIAN_POINT('Ctrl Pts',(1.64230807570083,0.280491037616897,13.4387673457008));
#56416=CARTESIAN_POINT('Ctrl Pts',(1.63791546024065,0.304703403121771,13.4403959886441));
#56417=CARTESIAN_POINT('Ctrl Pts',(1.63654011832794,0.312005856758478,13.4408903471462));
#56418=CARTESIAN_POINT('Ctrl Pts',(1.63406091403176,0.324701764141206,13.4417557242885));
#56419=CARTESIAN_POINT('Ctrl Pts',(1.63297909758993,0.330099336912054,13.4421255039631));
#56420=CARTESIAN_POINT('Ctrl Pts',(1.63060284967423,0.34165768584096,13.4429214851699));
#56421=CARTESIAN_POINT('Ctrl Pts',(1.62930026879551,0.347816414900361,13.4433481095066));
#56422=CARTESIAN_POINT('Ctrl Pts',(1.62562626459965,0.364713849182281,13.4445252066675));
#56423=CARTESIAN_POINT('Ctrl Pts',(1.62318341322813,0.375436459107247,13.445279484383));
#56424=CARTESIAN_POINT('Ctrl Pts',(1.60864725719351,0.43644588743802,13.4496100475103));
#56425=CARTESIAN_POINT('Ctrl Pts',(1.5943246158628,0.486167595361645,13.4532897920663));
#56426=CARTESIAN_POINT('Ctrl Pts',(1.54682683042447,0.626202626085136,13.4639468386568));
#56427=CARTESIAN_POINT('Ctrl Pts',(1.50811234273667,0.714423706511268,13.4710098991774));
#56428=CARTESIAN_POINT('Ctrl Pts',(1.43689683467623,0.844763274976809,13.4816893558122));
#56429=CARTESIAN_POINT('Ctrl Pts',(1.40963756537154,0.889505659470023,13.4854073257522));
#56430=CARTESIAN_POINT('Ctrl Pts',(1.36700508834127,0.952584884773113,13.4907128411085));
#56431=CARTESIAN_POINT('Ctrl Pts',(1.35327607537385,0.971990142080068,13.492354550582));
#56432=CARTESIAN_POINT('Ctrl Pts',(1.32761973893876,1.00665613460049,13.4953054711994));
#56433=CARTESIAN_POINT('Ctrl Pts',(1.31583282988615,1.02201505037389,13.4966196360212));
#56434=CARTESIAN_POINT('Ctrl Pts',(1.29686903061903,1.04585370298794,13.4986709366427));
#56435=CARTESIAN_POINT('Ctrl Pts',(1.2898707932599,1.05447266330533,13.4994150517637));
#56436=CARTESIAN_POINT('Ctrl Pts',(1.27658626579411,1.07050359099232,13.5008040008145));
#56437=CARTESIAN_POINT('Ctrl Pts',(1.27032030044567,1.07793171094363,13.501449615573));
#56438=CARTESIAN_POINT('Ctrl Pts',(1.25608802108515,1.0945071966981,13.5028951384433));
#56439=CARTESIAN_POINT('Ctrl Pts',(1.24808602625913,1.10362330728539,13.5036935356074));
#56440=CARTESIAN_POINT('Ctrl Pts',(1.22420703832332,1.1302350443473,13.5060351393241));
#56441=CARTESIAN_POINT('Ctrl Pts',(1.20805624409073,1.14748173371283,13.5075668518917));
#56442=CARTESIAN_POINT('Ctrl Pts',(1.12121219356062,1.23635175424994,13.5155490781954));
#56443=CARTESIAN_POINT('Ctrl Pts',(1.04450200498592,1.30180691117526,13.521727007672));
#56444=CARTESIAN_POINT('Ctrl Pts',(0.89631194875483,1.40667150828439,13.5328161457826));
#56445=CARTESIAN_POINT('Ctrl Pts',(0.826967695998072,1.44852423567307,13.5377284413919));
#56446=CARTESIAN_POINT('Ctrl Pts',(0.732550372742284,1.49651343739044,13.5444039369826));
#56447=CARTESIAN_POINT('Ctrl Pts',(0.709985259653346,1.50734976517217,13.5459988188556));
#56448=CARTESIAN_POINT('Ctrl Pts',(0.671381817628897,1.52482898373729,13.5487405664365));
#56449=CARTESIAN_POINT('Ctrl Pts',(0.655467719797646,1.53173724413384,13.5498745794582));
#56450=CARTESIAN_POINT('Ctrl Pts',(0.632560827739368,1.54125872280368,13.5515162451771));
#56451=CARTESIAN_POINT('Ctrl Pts',(0.625653235402655,1.54407567015345,13.552012493366));
#56452=CARTESIAN_POINT('Ctrl Pts',(0.613612275240564,1.5488919662284,13.5528800047154));
#56453=CARTESIAN_POINT('Ctrl Pts',(0.608487534973512,1.55091239796915,13.5532500097162));
#56454=CARTESIAN_POINT('Ctrl Pts',(0.597500109804599,1.55518135362252,13.5540450994273));
#56455=CARTESIAN_POINT('Ctrl Pts',(0.591634803735674,1.55742212634069,13.5544705948436));
#56456=CARTESIAN_POINT('Ctrl Pts',(0.575528857615562,1.56347110869394,13.5556416194534));
#56457=CARTESIAN_POINT('Ctrl Pts',(0.565263415286893,1.56721173718473,13.556390891968));
#56458=CARTESIAN_POINT('Ctrl Pts',(0.507613028939983,1.58757890712265,13.5606120528637));
#56459=CARTESIAN_POINT('Ctrl Pts',(0.459536245180714,1.60215579474568,13.564181501569));
#56460=CARTESIAN_POINT('Ctrl Pts',(0.315826916027447,1.63872804396251,13.5748602014975));
#56461=CARTESIAN_POINT('Ctrl Pts',(0.218822535736473,1.65447697896201,13.5820675301847));
#56462=CARTESIAN_POINT('Ctrl Pts',(0.068947111650721,1.66539047284085,13.5928711562973));
#56463=CARTESIAN_POINT('Ctrl Pts',(0.0167481776930115,1.66673318255776,
13.5965761550655));
#56464=CARTESIAN_POINT('Ctrl Pts',(-0.0591421275863616,1.66511880452352,
13.6018653978931));
#56465=CARTESIAN_POINT('Ctrl Pts',(-0.0828397490805629,1.66410819901216,
13.6035034348538));
#56466=CARTESIAN_POINT('Ctrl Pts',(-0.125794721988943,1.66135642232413,
13.6064484371513));
#56467=CARTESIAN_POINT('Ctrl Pts',(-0.145058377989086,1.6597854064981,13.6077603259338));
#56468=CARTESIAN_POINT('Ctrl Pts',(-0.175331846431883,1.65678539334367,
13.609808900019));
#56469=CARTESIAN_POINT('Ctrl Pts',(-0.186361649179719,1.65558099831943,
13.6105525337237));
#56470=CARTESIAN_POINT('Ctrl Pts',(-0.207028819953206,1.65311509449884,
13.6119410486164));
#56471=CARTESIAN_POINT('Ctrl Pts',(-0.216668718088043,1.6518792696185,13.6125867058587));
#56472=CARTESIAN_POINT('Ctrl Pts',(-0.238324314348732,1.64891021167148,
13.6140329240105));
#56473=CARTESIAN_POINT('Ctrl Pts',(-0.250333076225962,1.6471298458022,13.6148319675367));
#56474=CARTESIAN_POINT('Ctrl Pts',(-0.285699984000059,1.64149077482557,
13.617177379437));
#56475=CARTESIAN_POINT('Ctrl Pts',(-0.30899716580376,1.63726518520925,13.618712196327));
#56476=CARTESIAN_POINT('Ctrl Pts',(-0.429844577385538,1.61267461848072,
13.6266339965178));
#56477=CARTESIAN_POINT('Ctrl Pts',(-0.525516618505373,1.58408372494524,
13.6327545570776));
#56478=CARTESIAN_POINT('Ctrl Pts',(-0.693845206382381,1.51683663228789,
13.6438277354306));
#56479=CARTESIAN_POINT('Ctrl Pts',(-0.767290094424702,1.48103970721281,
13.6487809528885));
#56480=CARTESIAN_POINT('Ctrl Pts',(-0.870126671251356,1.42120841083277,
13.6562784316146));
#56481=CARTESIAN_POINT('Ctrl Pts',(-0.901797213001384,1.40132618438397,
13.658672574052));
#56482=CARTESIAN_POINT('Ctrl Pts',(-0.940923431179376,1.37488761110621,
13.6617753954154));
#56483=CARTESIAN_POINT('Ctrl Pts',(-0.949028215208555,1.36930576630687,
13.6624262713061));
#56484=CARTESIAN_POINT('Ctrl Pts',(-0.961976456792547,1.36021801218715,
13.6634801144471));
#56485=CARTESIAN_POINT('Ctrl Pts',(-0.96685146412288,1.35675715866733,13.663880120796));
#56486=CARTESIAN_POINT('Ctrl Pts',(-0.976221083068241,1.3500293593988,13.6646554097535));
#56487=CARTESIAN_POINT('Ctrl Pts',(-0.980718135153803,1.34676605616228,
13.6650304507609));
#56488=CARTESIAN_POINT('Ctrl Pts',(-0.990696712075996,1.33944858385314,
13.6658690519785));
#56489=CARTESIAN_POINT('Ctrl Pts',(-0.996169840212795,1.3353831395923,13.6663333654091));
#56490=CARTESIAN_POINT('Ctrl Pts',(-1.01233882568955,1.3232180876719,13.6677176580756));
#56491=CARTESIAN_POINT('Ctrl Pts',(-1.02296167288394,1.31502296311746,13.6686436321306));
#56492=CARTESIAN_POINT('Ctrl Pts',(-1.11775078980674,1.24005321068179,13.6770478036626));
#56493=CARTESIAN_POINT('Ctrl Pts',(-1.19536602389239,1.16541636455799,13.684928987173));
#56494=CARTESIAN_POINT('Ctrl Pts',(-1.33707113643737,0.999992349300045,
13.7007595888945));
#56495=CARTESIAN_POINT('Ctrl Pts',(-1.40039247174524,0.909204679859933,
13.7086606587543));
#56496=CARTESIAN_POINT('Ctrl Pts',(-1.46375495978593,0.795836181745914,
13.7175480643725));
#56497=CARTESIAN_POINT('Ctrl Pts',(-1.47294066768611,0.778703830393552,
13.7188677062834));
#56498=CARTESIAN_POINT('Ctrl Pts',(-1.48690633516537,0.751524566049916,
13.7209255669042));
#56499=CARTESIAN_POINT('Ctrl Pts',(-1.49188885135243,0.741584309785389,
13.7216708395729));
#56500=CARTESIAN_POINT('Ctrl Pts',(-1.50103809508365,0.72286584727561,13.7230608366402));
#56501=CARTESIAN_POINT('Ctrl Pts',(-1.50522823850449,0.714099679943736,
13.7237063533248));
#56502=CARTESIAN_POINT('Ctrl Pts',(-1.51446629478674,0.694330167065318,
13.7251502244848));
#56503=CARTESIAN_POINT('Ctrl Pts',(-1.51947148242464,0.683307372969721,
13.725947083331));
#56504=CARTESIAN_POINT('Ctrl Pts',(-1.53384182147373,0.65072106960216,13.728279636644));
#56505=CARTESIAN_POINT('Ctrl Pts',(-1.54287146842955,0.62901221315323,13.7298039731925));
#56506=CARTESIAN_POINT('Ctrl Pts',(-1.55554398581049,0.596628693154489,
13.732038227184));
#56507=CARTESIAN_POINT('Ctrl Pts',(-1.55954156847558,0.586099713912162,
13.7327585704354));
#56508=CARTESIAN_POINT('Ctrl Pts',(-1.56343128722854,0.575533326676141,
13.7334757494662));
#56509=CARTESIAN_POINT('Origin',(0.,0.,11.));
#56510=CARTESIAN_POINT('',(-1.56343129324813,0.575533310323967,14.4309760522469));
#56511=CARTESIAN_POINT('',(-1.56343134771032,0.575533162377876,14.2401853336637));
#56512=CARTESIAN_POINT('',(-1.56343130033213,0.575533291080363,11.));
#56513=CARTESIAN_POINT('',(-1.66599934497354,0.00147734482691685,13.5789038102816));
#56514=CARTESIAN_POINT('Ctrl Pts',(-1.56343134771032,0.575533162377876,
14.2401853336637));
#56515=CARTESIAN_POINT('Ctrl Pts',(-1.54563346535971,0.6238809709991,14.2369930364229));
#56516=CARTESIAN_POINT('Ctrl Pts',(-1.52559334840805,0.671401985184517,
14.2337520000224));
#56517=CARTESIAN_POINT('Ctrl Pts',(-1.49757772934425,0.730066810385444,
14.2295271102982));
#56518=CARTESIAN_POINT('Ctrl Pts',(-1.49164013259726,0.74212282705374,14.228646527073));
#56519=CARTESIAN_POINT('Ctrl Pts',(-1.48246906387274,0.760189470780374,
14.2273062252057));
#56520=CARTESIAN_POINT('Ctrl Pts',(-1.47934327443169,0.766254545960231,
14.2268527173139));
#56521=CARTESIAN_POINT('Ctrl Pts',(-1.47360413945224,0.777224372697188,
14.2260256687841));
#56522=CARTESIAN_POINT('Ctrl Pts',(-1.47100330149631,0.782135647627981,
14.2256528981661));
#56523=CARTESIAN_POINT('Ctrl Pts',(-1.46555501330078,0.792300581227544,
14.2248760014611));
#56524=CARTESIAN_POINT('Ctrl Pts',(-1.46270381546158,0.797552038062961,
14.2244716572804));
#56525=CARTESIAN_POINT('Ctrl Pts',(-1.45508859430806,0.811399887267858,
14.223397743613));
#56526=CARTESIAN_POINT('Ctrl Pts',(-1.45027673178433,0.819969501785932,
14.2227252866415));
#56527=CARTESIAN_POINT('Ctrl Pts',(-1.42687306751663,0.860799414295964,
14.2194852746845));
#56528=CARTESIAN_POINT('Ctrl Pts',(-1.40728044634848,0.89247053052591,14.2168634912301));
#56529=CARTESIAN_POINT('Ctrl Pts',(-1.34176895398326,0.990841446508917,
14.2084295866173));
#56530=CARTESIAN_POINT('Ctrl Pts',(-1.29204199221702,1.05486367364607,14.2025035926654));
#56531=CARTESIAN_POINT('Ctrl Pts',(-1.17058137687715,1.18970600930494,14.1893195173065));
#56532=CARTESIAN_POINT('Ctrl Pts',(-1.09667125964575,1.25816508452776,14.1821201096597));
#56533=CARTESIAN_POINT('Ctrl Pts',(-0.998310974699384,1.33397510882556,
14.173570776052));
#56534=CARTESIAN_POINT('Ctrl Pts',(-0.979289064811212,1.3480012685526,14.1719592169296));
#56535=CARTESIAN_POINT('Ctrl Pts',(-0.950060400568612,1.36860818889356,
14.1695440033051));
#56536=CARTESIAN_POINT('Ctrl Pts',(-0.940070228643677,1.37548941041134,
14.1687289585216));
#56537=CARTESIAN_POINT('Ctrl Pts',(-0.921943290830429,1.38768548053969,
14.1672684532143));
#56538=CARTESIAN_POINT('Ctrl Pts',(-0.91383357649876,1.39303934823724,14.1666215426324));
#56539=CARTESIAN_POINT('Ctrl Pts',(-0.89636059495744,1.40435640019398,14.1652413177582));
#56540=CARTESIAN_POINT('Ctrl Pts',(-0.886983596277834,1.41029760154465,
14.1645088423294));
#56541=CARTESIAN_POINT('Ctrl Pts',(-0.861097574966405,1.42633848922139,
14.1625086608307));
#56542=CARTESIAN_POINT('Ctrl Pts',(-0.844470530302214,1.43624513699585,
14.1612480166618));
#56543=CARTESIAN_POINT('Ctrl Pts',(-0.730415548716905,1.50153523367751,
14.1527534439515));
#56544=CARTESIAN_POINT('Ctrl Pts',(-0.627784055215815,1.54725771660207,
14.1458831227031));
#56545=CARTESIAN_POINT('Ctrl Pts',(-0.420819140924783,1.61544596338825,
14.1325757690076));
#56546=CARTESIAN_POINT('Ctrl Pts',(-0.31739842629686,1.63890403047336,14.1261573608561));
#56547=CARTESIAN_POINT('Ctrl Pts',(-0.197829185084652,1.65427853961648,
14.1183236842443));
#56548=CARTESIAN_POINT('Ctrl Pts',(-0.183165430651324,1.65596626219152,
14.1173558245408));
#56549=CARTESIAN_POINT('Ctrl Pts',(-0.161496397614285,1.65816893402883,
14.1159124818691));
#56550=CARTESIAN_POINT('Ctrl Pts',(-0.154506720980915,1.65883482268614,
14.1154449017786));
#56551=CARTESIAN_POINT('Ctrl Pts',(-0.142060615607765,1.65994118784928,
14.1146084037009));
#56552=CARTESIAN_POINT('Ctrl Pts',(-0.136605928331721,1.66039898354506,
14.1142404489481));
#56553=CARTESIAN_POINT('Ctrl Pts',(-0.124689668753647,1.66133996192484,
14.1134335935092));
#56554=CARTESIAN_POINT('Ctrl Pts',(-0.118227595407533,1.66181232836255,
14.1129941353254));
#56555=CARTESIAN_POINT('Ctrl Pts',(-0.0996240660430227,1.66306315785753,
14.1117238138352));
#56556=CARTESIAN_POINT('Ctrl Pts',(-0.0874769232334655,1.66374631115576,
14.110888023148));
#56557=CARTESIAN_POINT('Ctrl Pts',(-0.0596576469455694,1.66500537460731,
14.1089610324874));
#56558=CARTESIAN_POINT('Ctrl Pts',(-0.0439828416268084,1.66549314092908,
14.107865931585));
#56559=CARTESIAN_POINT('Ctrl Pts',(0.00879052807203655,1.66638985170575,
14.1041525076836));
#56560=CARTESIAN_POINT('Ctrl Pts',(0.0458936552049288,1.66578084923985,
14.1014979024997));
#56561=CARTESIAN_POINT('Ctrl Pts',(0.154192615018678,1.66038241316854,14.0936727626892));
#56562=CARTESIAN_POINT('Ctrl Pts',(0.225139961452177,1.65225818079694,14.0884525567434));
#56563=CARTESIAN_POINT('Ctrl Pts',(0.392780698625073,1.62206057255451,14.0761072669606));
#56564=CARTESIAN_POINT('Ctrl Pts',(0.488469176903136,1.59585752020852,14.0690619385057));
#56565=CARTESIAN_POINT('Ctrl Pts',(0.598952188973332,1.55472439847301,14.0610013049357));
#56566=CARTESIAN_POINT('Ctrl Pts',(0.616514083691443,1.54784434463828,14.0597217016109));
#56567=CARTESIAN_POINT('Ctrl Pts',(0.644124184180432,1.53648330061058,14.0577118572541));
#56568=CARTESIAN_POINT('Ctrl Pts',(0.654250891343624,1.5321986421189,14.0569751000901));
#56569=CARTESIAN_POINT('Ctrl Pts',(0.672366042715144,1.52432168644296,14.0556576244148));
#56570=CARTESIAN_POINT('Ctrl Pts',(0.680369899815099,1.52076609101846,14.0550756878771));
#56571=CARTESIAN_POINT('Ctrl Pts',(0.699104290881365,1.51226610435816,14.0537137529317));
#56572=CARTESIAN_POINT('Ctrl Pts',(0.709811097704624,1.50727031335604,14.0529355464373));
#56573=CARTESIAN_POINT('Ctrl Pts',(0.741035689520064,1.4922944232628,14.0506657262689));
#56574=CARTESIAN_POINT('Ctrl Pts',(0.761403195200306,1.48200600359717,14.0491847813041));
#56575=CARTESIAN_POINT('Ctrl Pts',(0.854510586831767,1.43254747595464,14.0424025466643));
#56576=CARTESIAN_POINT('Ctrl Pts',(0.924488179485203,1.38841799612802,14.0372773146484));
#56577=CARTESIAN_POINT('Ctrl Pts',(1.0370176359957,1.30515907449163,14.0286950754777));
#56578=CARTESIAN_POINT('Ctrl Pts',(1.08133293829069,1.26868624512614,14.0252109619448));
#56579=CARTESIAN_POINT('Ctrl Pts',(1.18056782468595,1.17802930381744,14.0169622835631));
#56580=CARTESIAN_POINT('Ctrl Pts',(1.23377562680633,1.12218002308815,14.0121795820669));
#56581=CARTESIAN_POINT('Ctrl Pts',(1.29032435379716,1.05392301236079,14.006381851432));
#56582=CARTESIAN_POINT('Ctrl Pts',(1.29763357951774,1.04491039270479,14.0056171555454));
#56583=CARTESIAN_POINT('Ctrl Pts',(1.30884618423056,1.03078563374416,14.0044186733575));
#56584=CARTESIAN_POINT('Ctrl Pts',(1.31281527588576,1.0257257940794,14.0039893402696));
#56585=CARTESIAN_POINT('Ctrl Pts',(1.32011231479558,1.01631171912152,14.0031902646955));
#56586=CARTESIAN_POINT('Ctrl Pts',(1.32344819184896,1.01196388987053,14.002821084287));
#56587=CARTESIAN_POINT('Ctrl Pts',(1.33112299369749,1.00185805178356,14.001962724409));
#56588=CARTESIAN_POINT('Ctrl Pts',(1.33544603590394,0.996088279534443,14.001472486976));
#56589=CARTESIAN_POINT('Ctrl Pts',(1.34919473411293,0.977488123683293,13.9998920341239));
#56590=CARTESIAN_POINT('Ctrl Pts',(1.35847365012393,0.964551065583285,13.9987926837506));
#56591=CARTESIAN_POINT('Ctrl Pts',(1.38030376940767,0.933174683519973,13.9961299766807));
#56592=CARTESIAN_POINT('Ctrl Pts',(1.39267263102929,0.914612665691757,13.9945576361085));
#56593=CARTESIAN_POINT('Ctrl Pts',(1.43988580768317,0.840580502041863,13.9883138760368));
#56594=CARTESIAN_POINT('Ctrl Pts',(1.47181742078354,0.783325794241625,13.9835465712049));
#56595=CARTESIAN_POINT('Ctrl Pts',(1.55331359258663,0.614527139730089,13.969901863511));
#56596=CARTESIAN_POINT('Ctrl Pts',(1.59412513062366,0.499201510077962,13.9610933799439));
#56597=CARTESIAN_POINT('Ctrl Pts',(1.62676149294236,0.36005723460561,13.951262784045));
#56598=CARTESIAN_POINT('Ctrl Pts',(1.6311571553045,0.339588826138155,13.9498349416575));
#56599=CARTESIAN_POINT('Ctrl Pts',(1.63756855242655,0.306728910578537,13.9475709110637));
#56600=CARTESIAN_POINT('Ctrl Pts',(1.63983192631386,0.294388615384434,13.9467269764598));
#56601=CARTESIAN_POINT('Ctrl Pts',(1.64361214699959,0.272379980739625,13.9452326962979));
#56602=CARTESIAN_POINT('Ctrl Pts',(1.64518358605755,0.262721751784548,13.9445806511672));
#56603=CARTESIAN_POINT('Ctrl Pts',(1.6483003688112,0.242439945547055,13.9432188993649));
#56604=CARTESIAN_POINT('Ctrl Pts',(1.64982831132455,0.231814117928783,13.9425097697681));
#56605=CARTESIAN_POINT('Ctrl Pts',(1.65359560538315,0.203688045354073,13.9406436221211));
#56606=CARTESIAN_POINT('Ctrl Pts',(1.65565990477688,0.186165422120089,13.9394921251335));
#56607=CARTESIAN_POINT('Ctrl Pts',(1.66486715616074,0.0956591143175343,
13.9335966812282));
#56608=CARTESIAN_POINT('Ctrl Pts',(1.66746466905398,0.0222900669585823,
13.9289968130541));
#56609=CARTESIAN_POINT('Ctrl Pts',(1.66221157731468,-0.149166442099089,
13.9184092242576));
#56610=CARTESIAN_POINT('Ctrl Pts',(1.65053357868766,-0.246851681141567,
13.9125048852937));
#56611=CARTESIAN_POINT('Ctrl Pts',(1.62412326944738,-0.372406347329133,
13.9045451698716));
#56612=CARTESIAN_POINT('Ctrl Pts',(1.61712676958313,-0.401701029241101,
13.9026598110306));
#56613=CARTESIAN_POINT('Ctrl Pts',(1.60185589100986,-0.458750009173098,
13.8989048108138));
#56614=CARTESIAN_POINT('Ctrl Pts',(1.59364422586159,-0.486509721322128,
13.8970380384637));
#56615=CARTESIAN_POINT('Ctrl Pts',(1.58183292350379,-0.522922376135999,
13.894519352753));
#56616=CARTESIAN_POINT('Ctrl Pts',(1.57887697231132,-0.531780693187206,
13.893901057406));
#56617=CARTESIAN_POINT('Ctrl Pts',(1.57394255919479,-0.546164129779019,
13.892887319373));
#56618=CARTESIAN_POINT('Ctrl Pts',(1.57200904936928,-0.551704615093206,
13.89249444526));
#56619=CARTESIAN_POINT('Ctrl Pts',(1.56814248244164,-0.562598928924352,
13.891717013266));
#56620=CARTESIAN_POINT('Ctrl Pts',(1.56621118938815,-0.567953261247392,
13.8913325575065));
#56621=CARTESIAN_POINT('Ctrl Pts',(1.56132237414522,-0.581292482588408,
13.890369035037));
#56622=CARTESIAN_POINT('Ctrl Pts',(1.55833102945422,-0.589264712314062,
13.8897880369667));
#56623=CARTESIAN_POINT('Ctrl Pts',(1.54650137756292,-0.620071799448701,
13.8875238407525));
#56624=CARTESIAN_POINT('Ctrl Pts',(1.53722165269512,-0.64273243528617,13.8858176465327));
#56625=CARTESIAN_POINT('Ctrl Pts',(1.51121919480198,-0.702441739492555,
13.8812275890391));
#56626=CARTESIAN_POINT('Ctrl Pts',(1.49363464222281,-0.73909605995518,13.8783114153314));
#56627=CARTESIAN_POINT('Ctrl Pts',(1.41843721688195,-0.882174823563911,
13.8666206778354));
#56628=CARTESIAN_POINT('Ctrl Pts',(1.35063621685571,-0.98284507183653,13.8577305146817));
#56629=CARTESIAN_POINT('Ctrl Pts',(1.24079926080148,-1.1128293885765,13.845713901872));
#56630=CARTESIAN_POINT('Ctrl Pts',(1.20742575525371,-1.14895428628584,13.8423003242044));
#56631=CARTESIAN_POINT('Ctrl Pts',(1.16101762901055,-1.19492899975054,13.8378527771523));
#56632=CARTESIAN_POINT('Ctrl Pts',(1.14936975050277,-1.206136997994,13.8367596503541));
#56633=CARTESIAN_POINT('Ctrl Pts',(1.12994828453142,-1.22428813035644,13.8349739617505));
#56634=CARTESIAN_POINT('Ctrl Pts',(1.122269615377,-1.23133077228182,13.8342771626411));
#56635=CARTESIAN_POINT('Ctrl Pts',(1.10716354434819,-1.24492689836098,13.8329239249175));
#56636=CARTESIAN_POINT('Ctrl Pts',(1.09974278647722,-1.25148707823925,13.8322672209326));
#56637=CARTESIAN_POINT('Ctrl Pts',(1.08203627521113,-1.26686106612458,13.8307189041629));
#56638=CARTESIAN_POINT('Ctrl Pts',(1.07170056471045,-1.2756164702845,13.8298297195221));
#56639=CARTESIAN_POINT('Ctrl Pts',(1.0361853513146,-1.30496510445069,13.8268221174587));
#56640=CARTESIAN_POINT('Ctrl Pts',(1.01050909888216,-1.32494739206604,13.8247280838217));
#56641=CARTESIAN_POINT('Ctrl Pts',(0.946075914446345,-1.37212845246582,
13.8196477977291));
#56642=CARTESIAN_POINT('Ctrl Pts',(0.906713012574381,-1.39845204921205,
13.8166919006341));
#56643=CARTESIAN_POINT('Ctrl Pts',(0.807692499540422,-1.45873003779954,
13.8095293113601));
#56644=CARTESIAN_POINT('Ctrl Pts',(0.746958094718095,-1.4907428724512,13.8053656004681));
#56645=CARTESIAN_POINT('Ctrl Pts',(0.664818609608883,-1.52775474603952,
13.7998517172005));
#56646=CARTESIAN_POINT('Ctrl Pts',(0.645045718180894,-1.53620777951307,
13.7985326368586));
#56647=CARTESIAN_POINT('Ctrl Pts',(0.564611272681701,-1.56876724247348,
13.7931804330185));
#56648=CARTESIAN_POINT('Ctrl Pts',(0.502727428624714,-1.5896790948502,13.7890946793647));
#56649=CARTESIAN_POINT('Ctrl Pts',(0.428732256208436,-1.60993042299665,
13.7840750992329));
#56650=CARTESIAN_POINT('Ctrl Pts',(0.417648936072857,-1.61284117715866,
13.7833197531945));
#56651=CARTESIAN_POINT('Ctrl Pts',(0.400331639152728,-1.61719866476476,
13.7821328525658));
#56652=CARTESIAN_POINT('Ctrl Pts',(0.394117611889677,-1.61872426534024,
13.7817056157596));
#56653=CARTESIAN_POINT('Ctrl Pts',(0.382611398806776,-1.62147896530772,
13.7809117901695));
#56654=CARTESIAN_POINT('Ctrl Pts',(0.377321800387743,-1.62271802024248,
13.7805457690901));
#56655=CARTESIAN_POINT('Ctrl Pts',(0.364981670268074,-1.62554501980323,
13.779689400248));
#56656=CARTESIAN_POINT('Ctrl Pts',(0.357926796742602,-1.6271129752856,13.7791979555529));
#56657=CARTESIAN_POINT('Ctrl Pts',(0.335204284521835,-1.63200815983335,
13.7776096197283));
#56658=CARTESIAN_POINT('Ctrl Pts',(0.319499333643773,-1.63515524487017,
13.7765034702519));
#56659=CARTESIAN_POINT('Ctrl Pts',(0.281644111067665,-1.64217482879068,
13.7738210428304));
#56660=CARTESIAN_POINT('Ctrl Pts',(0.25945639203253,-1.64582619124666,13.7722356151435));
#56661=CARTESIAN_POINT('Ctrl Pts',(0.171442144395756,-1.6584865168876,13.765911054626));
#56662=CARTESIAN_POINT('Ctrl Pts',(0.105177976392292,-1.66400319144999,
13.7610738493845));
#56663=CARTESIAN_POINT('Ctrl Pts',(-0.0817395807860534,-1.66835366240431,
13.7474638294159));
#56664=CARTESIAN_POINT('Ctrl Pts',(-0.202214437460003,-1.65807257065349,
13.7387616953583));
#56665=CARTESIAN_POINT('Ctrl Pts',(-0.341162978413611,-1.63082968095876,
13.7290212042229));
#56666=CARTESIAN_POINT('Ctrl Pts',(-0.361707668032832,-1.62639640274447,
13.7275876120691));
#56667=CARTESIAN_POINT('Ctrl Pts',(-0.394397417196678,-1.61869226563308,
13.7253163054304));
#56668=CARTESIAN_POINT('Ctrl Pts',(-0.406598280424448,-1.61567070496945,
13.7244707656162));
#56669=CARTESIAN_POINT('Ctrl Pts',(-0.428237884255776,-1.6100509683455,
13.7229746596417));
#56670=CARTESIAN_POINT('Ctrl Pts',(-0.437689994314263,-1.6075071639306,
13.7223223793115));
#56671=CARTESIAN_POINT('Ctrl Pts',(-0.457448896860064,-1.6020023373628,
13.7209611465605));
#56672=CARTESIAN_POINT('Ctrl Pts',(-0.467750654004095,-1.59902480184126,
13.7202527623937));
#56673=CARTESIAN_POINT('Ctrl Pts',(-0.494871308041044,-1.59090154160773,
13.7183908870772));
#56674=CARTESIAN_POINT('Ctrl Pts',(-0.511638994089605,-1.5855885042182,
13.7172428704566));
#56675=CARTESIAN_POINT('Ctrl Pts',(-0.596996012848846,-1.55704704383942,
13.7114098519396));
#56676=CARTESIAN_POINT('Ctrl Pts',(-0.664106598019126,-1.52962873299698,
13.7068650589325));
#56677=CARTESIAN_POINT('Ctrl Pts',(-0.789909425776177,-1.46838490236284,
13.6982250950865));
#56678=CARTESIAN_POINT('Ctrl Pts',(-0.848741156108113,-1.43518283132511,
13.6941276729167));
#56679=CARTESIAN_POINT('Ctrl Pts',(-0.972486968042734,-1.35506923630702,
13.6851051377307));
#56680=CARTESIAN_POINT('Ctrl Pts',(-1.03635633275848,-1.30686877467561,
13.6801783319021));
#56681=CARTESIAN_POINT('Ctrl Pts',(-1.10838978117183,-1.24389588515171,
13.6739706539603));
#56682=CARTESIAN_POINT('Ctrl Pts',(-1.12011837726404,-1.23334490581664,
13.6729372944684));
#56683=CARTESIAN_POINT('Ctrl Pts',(-1.13691070342952,-1.21780152994364,
13.6714214880085));
#56684=CARTESIAN_POINT('Ctrl Pts',(-1.1420954897882,-1.21294039487503,13.6709483214237));
#56685=CARTESIAN_POINT('Ctrl Pts',(-1.15122409152189,-1.20427120904506,
13.6701057230189));
#56686=CARTESIAN_POINT('Ctrl Pts',(-1.15518044786978,-1.20047664926562,
13.6697373101891));
#56687=CARTESIAN_POINT('Ctrl Pts',(-1.16283254150445,-1.1930646346198,13.6690183625882));
#56688=CARTESIAN_POINT('Ctrl Pts',(-1.16653014622713,-1.18944951892796,
13.6686680367671));
#56689=CARTESIAN_POINT('Ctrl Pts',(-1.17693583912778,-1.17918077509708,
13.6676740257869));
#56690=CARTESIAN_POINT('Ctrl Pts',(-1.18360410971571,-1.17248734357653,
13.667027385642));
#56691=CARTESIAN_POINT('Ctrl Pts',(-1.21629711548992,-1.13910787880694,
13.6638105917625));
#56692=CARTESIAN_POINT('Ctrl Pts',(-1.24147608955379,-1.11161237426235,
13.6611857879259));
#56693=CARTESIAN_POINT('Ctrl Pts',(-1.31851935295915,-1.02159617019656,
13.6527303637501));
#56694=CARTESIAN_POINT('Ctrl Pts',(-1.36674463254303,-0.956117313027135,
13.6467852495804));
#56695=CARTESIAN_POINT('Ctrl Pts',(-1.46335756600952,-0.802605262317195,
13.6336090333831));
#56696=CARTESIAN_POINT('Ctrl Pts',(-1.5089664705099,-0.713173743223769,
13.6264357489282));
#56697=CARTESIAN_POINT('Ctrl Pts',(-1.55506955322967,-0.598225566857417,
13.6179093717365));
#56698=CARTESIAN_POINT('Ctrl Pts',(-1.56340403948772,-0.576092920493208,
13.6162967056883));
#56699=CARTESIAN_POINT('Ctrl Pts',(-1.5752981142217,-0.542345895267034,
13.6138801782969));
#56700=CARTESIAN_POINT('Ctrl Pts',(-1.5792062842643,-0.53085849718675,13.613064908146));
#56701=CARTESIAN_POINT('Ctrl Pts',(-1.58601785467818,-0.510095867559207,
13.6116041587127));
#56702=CARTESIAN_POINT('Ctrl Pts',(-1.58896622093097,-0.500836086025938,
13.6109572272941));
#56703=CARTESIAN_POINT('Ctrl Pts',(-1.59510789100386,-0.480946962539583,
13.6095771278574));
#56704=CARTESIAN_POINT('Ctrl Pts',(-1.59827635500801,-0.47031039512805,
13.6088447971468));
#56705=CARTESIAN_POINT('Ctrl Pts',(-1.60667469781162,-0.44105160928162,
13.606845450595));
#56706=CARTESIAN_POINT('Ctrl Pts',(-1.61168704269081,-0.422368362481585,
13.6055854865577));
#56707=CARTESIAN_POINT('Ctrl Pts',(-1.62212464255702,-0.380567083425392,
13.6028005949439));
#56708=CARTESIAN_POINT('Ctrl Pts',(-1.62738338033289,-0.357411637320071,
13.6012809151057));
#56709=CARTESIAN_POINT('Ctrl Pts',(-1.65475686652148,-0.223706991316348,
13.5926196156324));
#56710=CARTESIAN_POINT('Ctrl Pts',(-1.66609931397845,-0.11125753849907,
13.5858033966699));
#56711=CARTESIAN_POINT('Ctrl Pts',(-1.66599934497354,0.00147734482691685,
13.5789038102816));
#56712=CARTESIAN_POINT('Ctrl Pts',(-1.66599934402992,0.00147840856629485,
13.5789037451788));
#56713=CARTESIAN_POINT('Ctrl Pts',(-1.66592908092197,0.0806569891074675,
13.574057867085));
#56714=CARTESIAN_POINT('Ctrl Pts',(-1.6602143015703,0.159723172896025,13.5691777217738));
#56715=CARTESIAN_POINT('Ctrl Pts',(-1.64726516269832,0.249408511033996,
13.5633054302498));
#56716=CARTESIAN_POINT('Ctrl Pts',(-1.6455120615802,0.260724299713883,13.5625582417345));
#56717=CARTESIAN_POINT('Ctrl Pts',(-1.64248438447374,0.279018560692953,
13.5613387763251));
#56718=CARTESIAN_POINT('Ctrl Pts',(-1.64128160451835,0.286008742536837,
13.5608700963127));
#56719=CARTESIAN_POINT('Ctrl Pts',(-1.63908799017727,0.298287632070213,
13.5600416776263));
#56720=CARTESIAN_POINT('Ctrl Pts',(-1.63811609140399,0.303579676626428,
13.5596829558826));
#56721=CARTESIAN_POINT('Ctrl Pts',(-1.63611223900365,0.314200901439896,
13.5589594396421));
#56722=CARTESIAN_POINT('Ctrl Pts',(-1.6350798705893,0.319529780461453,13.5585946214091));
#56723=CARTESIAN_POINT('Ctrl Pts',(-1.63276757311799,0.331160690881833,
13.5577943014799));
#56724=CARTESIAN_POINT('Ctrl Pts',(-1.6314772142538,0.3374602893509,13.5573582478506));
#56725=CARTESIAN_POINT('Ctrl Pts',(-1.6277565484286,0.355104529492732,13.5561299830623));
#56726=CARTESIAN_POINT('Ctrl Pts',(-1.62524421130851,0.366431224965538,
13.5553334307419));
#56727=CARTESIAN_POINT('Ctrl Pts',(-1.60699162244934,0.444838754306764,
13.5497675594891));
#56728=CARTESIAN_POINT('Ctrl Pts',(-1.58722440750297,0.510899516444609,
13.5448165457068));
#56729=CARTESIAN_POINT('Ctrl Pts',(-1.56343130308087,0.575533283613436,
13.5398191707253));
#56730=CARTESIAN_POINT('Ctrl Pts',(-1.56343128722854,0.575533326676141,
13.7334757494662));
#56731=CARTESIAN_POINT('Ctrl Pts',(-1.59690734452391,0.484595907550651,
13.7396480019741));
#56732=CARTESIAN_POINT('Ctrl Pts',(-1.62239473420442,0.390886997980895,
13.7455715221201));
#56733=CARTESIAN_POINT('Ctrl Pts',(-1.65292263072649,0.221481194025369,
13.7560824791613));
#56734=CARTESIAN_POINT('Ctrl Pts',(-1.66123106262291,0.146686404472933,
13.7606625393582));
#56735=CARTESIAN_POINT('Ctrl Pts',(-1.66549569668114,0.0475373490342522,
13.7669268541262));
#56736=CARTESIAN_POINT('Ctrl Pts',(-1.66600871481831,0.0234639447436344,
13.7684630656757));
#56737=CARTESIAN_POINT('Ctrl Pts',(-1.66599370775538,-0.017467284978389,
13.7711135804174));
#56738=CARTESIAN_POINT('Ctrl Pts',(-1.66573169945979,-0.0343218927635916,
13.7722161249464));
#56739=CARTESIAN_POINT('Ctrl Pts',(-1.66498991816257,-0.058462075114235,
13.7738149067866));
#56740=CARTESIAN_POINT('Ctrl Pts',(-1.66471790388819,-0.0657536108263884,
13.7743003900498));
#56741=CARTESIAN_POINT('Ctrl Pts',(-1.66415667463459,-0.078542097544096,
13.7751567527131));
#56742=CARTESIAN_POINT('Ctrl Pts',(-1.66388810168304,-0.0840397696474318,
13.7755264907577));
#56743=CARTESIAN_POINT('Ctrl Pts',(-1.66325379827517,-0.0958252009860064,
13.7763226435167));
#56744=CARTESIAN_POINT('Ctrl Pts',(-1.66287966297194,-0.102112143263391,
13.7767494833393));
#56745=CARTESIAN_POINT('Ctrl Pts',(-1.66173409061338,-0.119681680786548,
13.7779480140864));
#56746=CARTESIAN_POINT('Ctrl Pts',(-1.6608834224287,-0.13095851331003,13.7787238328882));
#56747=CARTESIAN_POINT('Ctrl Pts',(-1.65440164952627,-0.206607521168572,
13.7839684999097));
#56748=CARTESIAN_POINT('Ctrl Pts',(-1.64514477056455,-0.270607275773206,
13.7885992513743));
#56749=CARTESIAN_POINT('Ctrl Pts',(-1.61097126101745,-0.437656990091769,
13.800952900476));
#56750=CARTESIAN_POINT('Ctrl Pts',(-1.57989789606257,-0.539164379848463,
13.8087181971043));
#56751=CARTESIAN_POINT('Ctrl Pts',(-1.51745878080532,-0.690047952664943,
13.8203210207799));
#56752=CARTESIAN_POINT('Ctrl Pts',(-1.49279640673099,-0.741894565033315,
13.824324417634));
#56753=CARTESIAN_POINT('Ctrl Pts',(-1.45735579329292,-0.807442670830319,
13.8294057940845));
#56754=CARTESIAN_POINT('Ctrl Pts',(-1.44897435276337,-0.822388556608074,
13.8305660001918));
#56755=CARTESIAN_POINT('Ctrl Pts',(-1.43502372122993,-0.846389882078534,
13.8324323821163));
#56756=CARTESIAN_POINT('Ctrl Pts',(-1.42959601266344,-0.855525664489342,
13.8331435723364));
#56757=CARTESIAN_POINT('Ctrl Pts',(-1.41898565994668,-0.873001774523313,
13.8345057892088));
#56758=CARTESIAN_POINT('Ctrl Pts',(-1.41381597911393,-0.88134941180789,
13.8351572513455));
#56759=CARTESIAN_POINT('Ctrl Pts',(-1.4016317106287,-0.900640603279529,
13.8366648967803));
#56760=CARTESIAN_POINT('Ctrl Pts',(-1.3945621835962,-0.911548836044693,
13.8375190114648));
#56761=CARTESIAN_POINT('Ctrl Pts',(-1.37119902967193,-0.946689953675526,
13.8402769861834));
#56762=CARTESIAN_POINT('Ctrl Pts',(-1.35439529193294,-0.97057828426904,
13.8421617669755));
#56763=CARTESIAN_POINT('Ctrl Pts',(-1.31264535720652,-1.02673290900314,
13.8466290331867));
#56764=CARTESIAN_POINT('Ctrl Pts',(-1.28712528665374,-1.05854954755507,
13.8491903354024));
#56765=CARTESIAN_POINT('Ctrl Pts',(-1.21288904200386,-1.14444271028742,
13.8562448222403));
#56766=CARTESIAN_POINT('Ctrl Pts',(-1.1617602368724,-1.19631207883954,13.8606671679549));
#56767=CARTESIAN_POINT('Ctrl Pts',(-1.04224443942692,-1.3026470017796,13.8704446402259));
#56768=CARTESIAN_POINT('Ctrl Pts',(-0.972640954062778,-1.35540710744694,
13.8757952959062));
#56769=CARTESIAN_POINT('Ctrl Pts',(-0.885925216762125,-1.41100766923844,
13.8824781461167));
#56770=CARTESIAN_POINT('Ctrl Pts',(-0.8724910691607,-1.41935387481402,13.8835140458672));
#56771=CARTESIAN_POINT('Ctrl Pts',(-0.852844605016776,-1.43117528541889,
13.8850329205947));
#56772=CARTESIAN_POINT('Ctrl Pts',(-0.846725163287895,-1.43480420655579,
13.8855065630757));
#56773=CARTESIAN_POINT('Ctrl Pts',(-0.835848762816267,-1.44116026538775,
13.8863497028104));
#56774=CARTESIAN_POINT('Ctrl Pts',(-0.831101308808723,-1.44390327864392,
13.886718176476));
#56775=CARTESIAN_POINT('Ctrl Pts',(-0.820771194398557,-1.44980404919066,
13.8875210206744));
#56776=CARTESIAN_POINT('Ctrl Pts',(-0.815183900759726,-1.45295297208106,
13.8879559011228));
#56777=CARTESIAN_POINT('Ctrl Pts',(-0.799220160707728,-1.46182885592752,
13.8891999427054));
#56778=CARTESIAN_POINT('Ctrl Pts',(-0.788800839435235,-1.46747732009287,
13.8900137309961));
#56779=CARTESIAN_POINT('Ctrl Pts',(-0.764917469109515,-1.48009700042222,
13.8918817392855));
#56780=CARTESIAN_POINT('Ctrl Pts',(-0.751416870193818,-1.48699647490331,
13.8929395452345));
#56781=CARTESIAN_POINT('Ctrl Pts',(-0.607749287548945,-1.55796167874946,
13.9042019219814));
#56782=CARTESIAN_POINT('Ctrl Pts',(-0.469839880225167,-1.60494788488956,
13.9149939478272));
#56783=CARTESIAN_POINT('Ctrl Pts',(-0.263141831534131,-1.64639967878009,
13.9300527313247));
#56784=CARTESIAN_POINT('Ctrl Pts',(-0.197987113674817,-1.65549949821642,
13.9346583385637));
#56785=CARTESIAN_POINT('Ctrl Pts',(-0.114812973027509,-1.66213335224514,
13.9403532567623));
#56786=CARTESIAN_POINT('Ctrl Pts',(-0.0971468685908385,-1.66325939868617,
13.9415526200734));
#56787=CARTESIAN_POINT('Ctrl Pts',(-0.068730293876874,-1.66461636888101,
13.9434661008017));
#56788=CARTESIAN_POINT('Ctrl Pts',(-0.0579901021721132,-1.66502512481235,
13.9441857082034));
#56789=CARTESIAN_POINT('Ctrl Pts',(-0.0374682900296803,-1.66560734187425,
13.9455540792577));
#56790=CARTESIAN_POINT('Ctrl Pts',(-0.0276876677031915,-1.66579863431472,
13.94620337125));
#56791=CARTESIAN_POINT('Ctrl Pts',(-0.00517194848982917,-1.66604064155266,
13.9476917751412));
#56792=CARTESIAN_POINT('Ctrl Pts',(0.00756328461740996,-1.66603150632131,
13.9485289887587));
#56793=CARTESIAN_POINT('Ctrl Pts',(0.0479863421841862,-1.66553898150288,
13.9511726802899));
#56794=CARTESIAN_POINT('Ctrl Pts',(0.0756636928236562,-1.66451132037318,
13.9529622757695));
#56795=CARTESIAN_POINT('Ctrl Pts',(0.169981547628219,-1.65865166371449,
13.9590055428783));
#56796=CARTESIAN_POINT('Ctrl Pts',(0.236353362100754,-1.65050217985981,
13.9631610528561));
#56797=CARTESIAN_POINT('Ctrl Pts',(0.368968746489921,-1.62605250914784,
13.9714504377125));
#56798=CARTESIAN_POINT('Ctrl Pts',(0.435056534029288,-1.60963052189566,
13.9755748475033));
#56799=CARTESIAN_POINT('Ctrl Pts',(0.571112886112889,-1.56682822395221,
13.984335735421));
#56800=CARTESIAN_POINT('Ctrl Pts',(0.640678368346614,-1.53969118887545,
13.9889738500163));
#56801=CARTESIAN_POINT('Ctrl Pts',(0.718679068260095,-1.5030605049748,13.9946104608379));
#56802=CARTESIAN_POINT('Ctrl Pts',(0.729123826646564,-1.49802166596762,
13.9953746859146));
#56803=CARTESIAN_POINT('Ctrl Pts',(0.745276134725738,-1.49002040974556,
13.9965725985625));
#56804=CARTESIAN_POINT('Ctrl Pts',(0.751020808986579,-1.48713317475332,
13.9970018399053));
#56805=CARTESIAN_POINT('Ctrl Pts',(0.761584862772429,-1.48174693107588,
13.9977973619751));
#56806=CARTESIAN_POINT('Ctrl Pts',(0.766408916516391,-1.47925753016715,
13.9981630527844));
#56807=CARTESIAN_POINT('Ctrl Pts',(0.777586659711129,-1.47342002333525,
13.9990159736937));
#56808=CARTESIAN_POINT('Ctrl Pts',(0.783930922955666,-1.47005438055086,
13.9995042705434));
#56809=CARTESIAN_POINT('Ctrl Pts',(0.804131556798847,-1.45916995965191,
14.0010720242152));
#56810=CARTESIAN_POINT('Ctrl Pts',(0.817902574273019,-1.45149573397758,
14.0021604185546));
#56811=CARTESIAN_POINT('Ctrl Pts',(0.893342255540834,-1.40804078040072,
14.0082236479097));
#56812=CARTESIAN_POINT('Ctrl Pts',(0.952768541965973,-1.36852816136779,
14.013373318905));
#56813=CARTESIAN_POINT('Ctrl Pts',(1.11351912187899,-1.24608845907502,14.0280629963583));
#56814=CARTESIAN_POINT('Ctrl Pts',(1.20788922694154,-1.1548490953192,14.0375907308053));
#56815=CARTESIAN_POINT('Ctrl Pts',(1.30857077993604,-1.03150584780667,14.0486098530869));
#56816=CARTESIAN_POINT('Ctrl Pts',(1.32595699847586,-1.00905897226283,14.0505528309424));
#56817=CARTESIAN_POINT('Ctrl Pts',(1.35029091686853,-0.975926334388468,
14.0533338785534));
#56818=CARTESIAN_POINT('Ctrl Pts',(1.35770231850719,-0.965589043137195,
14.0541897640057));
#56819=CARTESIAN_POINT('Ctrl Pts',(1.37061911500879,-0.947130126295397,
14.0556977193082));
#56820=CARTESIAN_POINT('Ctrl Pts',(1.37617243664457,-0.9390429522988,14.056351597411));
#56821=CARTESIAN_POINT('Ctrl Pts',(1.3876060593441,-0.922073146572204,14.0577098464854));
#56822=CARTESIAN_POINT('Ctrl Pts',(1.39347326710886,-0.91318219776115,14.0584137040025));
#56823=CARTESIAN_POINT('Ctrl Pts',(1.40862008826219,-0.889743319234936,
14.0602494997496));
#56824=CARTESIAN_POINT('Ctrl Pts',(1.417759825554,-0.875106188139725,14.0613762446505));
#56825=CARTESIAN_POINT('Ctrl Pts',(1.46138709288515,-0.802759759546435,
14.0668544369618));
#56826=CARTESIAN_POINT('Ctrl Pts',(1.49258943672587,-0.743137823823686,
14.0710864939885));
#56827=CARTESIAN_POINT('Ctrl Pts',(1.5494764243807,-0.61630317146352,14.0796939160186));
#56828=CARTESIAN_POINT('Ctrl Pts',(1.5745853162922,-0.548988321344521,14.0840504569113));
#56829=CARTESIAN_POINT('Ctrl Pts',(1.60171476774321,-0.458873435370217,
14.0898084522344));
#56830=CARTESIAN_POINT('Ctrl Pts',(1.60772351303908,-0.437355807994128,
14.0911783185495));
#56831=CARTESIAN_POINT('Ctrl Pts',(1.62970795671963,-0.352040950860208,
14.0966110233857));
#56832=CARTESIAN_POINT('Ctrl Pts',(1.64233116413986,-0.287449308485304,
14.1007260023808));
#56833=CARTESIAN_POINT('Ctrl Pts',(1.65263440578785,-0.210919736968887,
14.1057783854534));
#56834=CARTESIAN_POINT('Ctrl Pts',(1.65404759293201,-0.199534851672858,
14.1065345770714));
#56835=CARTESIAN_POINT('Ctrl Pts',(1.65606597753578,-0.181775852875196,
14.1077225388363));
#56836=CARTESIAN_POINT('Ctrl Pts',(1.65675222693959,-0.17541105365782,14.1081499791475));
#56837=CARTESIAN_POINT('Ctrl Pts',(1.65795301339992,-0.163637774595942,
14.1089439971056));
#56838=CARTESIAN_POINT('Ctrl Pts',(1.65847779879922,-0.158230539557421,
14.1093100049644));
#56839=CARTESIAN_POINT('Ctrl Pts',(1.65963871188628,-0.145628026669224,
14.1101660988646));
#56840=CARTESIAN_POINT('Ctrl Pts',(1.66025449844327,-0.138431108063503,
14.1106572791763));
#56841=CARTESIAN_POINT('Ctrl Pts',(1.66208334677203,-0.115285632797208,
14.1122438014421));
#56842=CARTESIAN_POINT('Ctrl Pts',(1.66311349816753,-0.0993240859317914,
14.1133483728752));
#56843=CARTESIAN_POINT('Ctrl Pts',(1.6650364676999,-0.0609363305812858,
14.1160261990991));
#56844=CARTESIAN_POINT('Ctrl Pts',(1.66570619735426,-0.0385024323218801,
14.1176085644583));
#56845=CARTESIAN_POINT('Ctrl Pts',(1.66656100022466,0.0501504940092083,
14.1239140517943));
#56846=CARTESIAN_POINT('Ctrl Pts',(1.66325127128114,0.116339770687247,14.1287347263514));
#56847=CARTESIAN_POINT('Ctrl Pts',(1.64279723960893,0.30229442939699,14.1423526692694));
#56848=CARTESIAN_POINT('Ctrl Pts',(1.6165449451845,0.42066285258121,14.1510796441945));
#56849=CARTESIAN_POINT('Ctrl Pts',(1.57096126496172,0.555047362847885,14.160841290152));
#56850=CARTESIAN_POINT('Ctrl Pts',(1.5638409425753,0.574802963632138,14.1622736291101));
#56851=CARTESIAN_POINT('Ctrl Pts',(1.55186599204742,0.606156578215076,14.1645433733652));
#56852=CARTESIAN_POINT('Ctrl Pts',(1.54725048896099,0.617842855432122,14.1653885865108));
#56853=CARTESIAN_POINT('Ctrl Pts',(1.53880490694127,0.638538378067501,14.1668843492923));
#56854=CARTESIAN_POINT('Ctrl Pts',(1.53502684296416,0.647568066151652,14.1675366098915));
#56855=CARTESIAN_POINT('Ctrl Pts',(1.52694217293726,0.666422278413724,14.1688980356776));
#56856=CARTESIAN_POINT('Ctrl Pts',(1.52261980791339,0.676239589412489,14.1696066305005));
#56857=CARTESIAN_POINT('Ctrl Pts',(1.51095510017821,0.702054478327146,14.1714695970835));
#56858=CARTESIAN_POINT('Ctrl Pts',(1.50345340713519,0.717978896851077,14.1726184829249));
#56859=CARTESIAN_POINT('Ctrl Pts',(1.46371062020843,0.798988394382672,14.1784663329392));
#56860=CARTESIAN_POINT('Ctrl Pts',(1.42748878356235,0.862037655032408,14.1830241775081));
#56861=CARTESIAN_POINT('Ctrl Pts',(1.33066376198011,1.00763955504913,14.19382042707));
#56862=CARTESIAN_POINT('Ctrl Pts',(1.26635479479252,1.08735809071863,14.1999583155859));
#56863=CARTESIAN_POINT('Ctrl Pts',(1.15864948543114,1.19826213614846,14.2095693458024));
#56864=CARTESIAN_POINT('Ctrl Pts',(1.12040092141735,1.23409942210474,14.2128806359686));
#56865=CARTESIAN_POINT('Ctrl Pts',(1.07212832918019,1.27523282470831,14.2170343202856));
#56866=CARTESIAN_POINT('Ctrl Pts',(1.06365352622961,1.28231005279961,14.2177626676304));
#56867=CARTESIAN_POINT('Ctrl Pts',(1.05022992805273,1.29329534557193,14.218916107369));
#56868=CARTESIAN_POINT('Ctrl Pts',(1.04532804091898,1.29726058918095,14.2193372629176));
#56869=CARTESIAN_POINT('Ctrl Pts',(1.03610584054368,1.3046344201951,14.2201297776281));
#56870=CARTESIAN_POINT('Ctrl Pts',(1.03179100376537,1.30804954195551,14.220500667775));
#56871=CARTESIAN_POINT('Ctrl Pts',(1.02162364722663,1.31601522899526,14.2213747619966));
#56872=CARTESIAN_POINT('Ctrl Pts',(1.01575759268414,1.32054816920395,14.2218791594218));
#56873=CARTESIAN_POINT('Ctrl Pts',(0.996279948621298,1.33539277766861,14.2235537149904));
#56874=CARTESIAN_POINT('Ctrl Pts',(0.98254057598484,1.34553393371724,14.2247345350109));
#56875=CARTESIAN_POINT('Ctrl Pts',(0.94871391290658,1.36970735488041,14.2276360762472));
#56876=CARTESIAN_POINT('Ctrl Pts',(0.928468573089017,1.3835108628743,14.2293678936929));
#56877=CARTESIAN_POINT('Ctrl Pts',(0.842806475686264,1.4391891992739,14.2366536703101));
#56878=CARTESIAN_POINT('Ctrl Pts',(0.774808085372231,1.47690888559529,14.2423325778821));
#56879=CARTESIAN_POINT('Ctrl Pts',(0.609402569674346,1.55408512573538,14.2556021897228));
#56880=CARTESIAN_POINT('Ctrl Pts',(0.510387408529094,1.58935949182553,14.2631255045931));
#56881=CARTESIAN_POINT('Ctrl Pts',(0.385850853920188,1.62087338626537,14.2719685751625));
#56882=CARTESIAN_POINT('Ctrl Pts',(0.362882682655123,1.62616963227339,14.273575739125));
#56883=CARTESIAN_POINT('Ctrl Pts',(0.327946063431739,1.63344856451324,14.2759857608915));
#56884=CARTESIAN_POINT('Ctrl Pts',(0.316056440094031,1.63579068757721,14.2767999352857));
#56885=CARTESIAN_POINT('Ctrl Pts',(0.294588630619136,1.63977679975059,14.2782595294737));
#56886=CARTESIAN_POINT('Ctrl Pts',(0.285019712736391,1.64146708297987,14.2789063910446));
#56887=CARTESIAN_POINT('Ctrl Pts',(0.264479204257985,1.64491038783715,14.2802872034649));
#56888=CARTESIAN_POINT('Ctrl Pts',(0.253503714716543,1.64663757705837,14.2810203090113));
#56889=CARTESIAN_POINT('Ctrl Pts',(0.223320981858193,1.65107843213516,14.283024009865));
#56890=CARTESIAN_POINT('Ctrl Pts',(0.204081958792875,1.65356670717591,14.2842875011597));
#56891=CARTESIAN_POINT('Ctrl Pts',(0.161122038762,1.65836168315444,14.2870813461343));
#56892=CARTESIAN_POINT('Ctrl Pts',(0.13738607460186,1.66049659288428,14.2886063990721));
#56893=CARTESIAN_POINT('Ctrl Pts',(0.0611651235402701,1.66570654906469,
14.293454237166));
#56894=CARTESIAN_POINT('Ctrl Pts',(0.00857596109655154,1.66680729428791,
14.2967231293628));
#56895=CARTESIAN_POINT('Ctrl Pts',(-0.139988420360405,1.66288400056109,
14.3058718144097));
#56896=CARTESIAN_POINT('Ctrl Pts',(-0.235592695276462,1.65205165053418,
14.3116506832653));
#56897=CARTESIAN_POINT('Ctrl Pts',(-0.38023238356863,1.62284752450269,14.3208300942808));
#56898=CARTESIAN_POINT('Ctrl Pts',(-0.430232065686764,1.61031363517197,
14.3240889071116));
#56899=CARTESIAN_POINT('Ctrl Pts',(-0.49008808860655,1.5923223297312,14.3281828946092));
#56900=CARTESIAN_POINT('Ctrl Pts',(-0.50057912825653,1.58905546059781,14.3289077941412));
#56901=CARTESIAN_POINT('Ctrl Pts',(-0.517026285111783,1.58375484886205,
14.330056956114));
#56902=CARTESIAN_POINT('Ctrl Pts',(-0.523004722428193,1.58179064918334,
14.3304773292493));
#56903=CARTESIAN_POINT('Ctrl Pts',(-0.534192553735803,1.57804455832385,
14.3312692504196));
#56904=CARTESIAN_POINT('Ctrl Pts',(-0.539404416768615,1.57627065701313,
14.3316403385264));
#56905=CARTESIAN_POINT('Ctrl Pts',(-0.551633579712859,1.57204060661297,
14.3325160938859));
#56906=CARTESIAN_POINT('Ctrl Pts',(-0.558643329468597,1.56956328329489,
14.3330219685981));
#56907=CARTESIAN_POINT('Ctrl Pts',(-0.581814836249913,1.56119933125588,
14.3347065757807));
#56908=CARTESIAN_POINT('Ctrl Pts',(-0.597901394769871,1.55510955245316,
14.3358961403127));
#56909=CARTESIAN_POINT('Ctrl Pts',(-0.636890889592165,1.53965520639481,
14.3388236547314));
#56910=CARTESIAN_POINT('Ctrl Pts',(-0.659684653274981,1.53002751191172,
14.340572944235));
#56911=CARTESIAN_POINT('Ctrl Pts',(-0.754432703746267,1.48749680646883,
14.3479813631546));
#56912=CARTESIAN_POINT('Ctrl Pts',(-0.824208677126646,1.44999815623618,
14.3537689631674));
#56913=CARTESIAN_POINT('Ctrl Pts',(-0.977898075333685,1.35271400981485,
14.3669885791716));
#56914=CARTESIAN_POINT('Ctrl Pts',(-1.0594817289804,1.28981578590912,14.3743570592595));
#56915=CARTESIAN_POINT('Ctrl Pts',(-1.15210803301264,1.20364641015806,14.3830672093403));
#56916=CARTESIAN_POINT('Ctrl Pts',(-1.1691133195215,1.18713594279958,14.3846834905366));
#56917=CARTESIAN_POINT('Ctrl Pts',(-1.19429208677732,1.16162381970452,14.3871043335213));
#56918=CARTESIAN_POINT('Ctrl Pts',(-1.20272825581565,1.15288691694172,14.3879203644517));
#56919=CARTESIAN_POINT('Ctrl Pts',(-1.21774235343396,1.13699341092075,14.3893819694509));
#56920=CARTESIAN_POINT('Ctrl Pts',(-1.22435454320049,1.12987008777023,14.3900290024176));
#56921=CARTESIAN_POINT('Ctrl Pts',(-1.23837845071978,1.11449442888469,14.3914087802236));
#56922=CARTESIAN_POINT('Ctrl Pts',(-1.24577088568864,1.10622508089439,14.3921406925872));
#56923=CARTESIAN_POINT('Ctrl Pts',(-1.26532010631377,1.08391235862654,14.3940891825104));
#56924=CARTESIAN_POINT('Ctrl Pts',(-1.27732577785194,1.06973822719028,14.3952995215685));
#56925=CARTESIAN_POINT('Ctrl Pts',(-1.33622300240261,0.997797334196229,
14.4013130821882));
#56926=CARTESIAN_POINT('Ctrl Pts',(-1.37944767345773,0.937132607897802,
14.4059695985546));
#56927=CARTESIAN_POINT('Ctrl Pts',(-1.45919537957205,0.807671111200176,
14.4153407664011));
#56928=CARTESIAN_POINT('Ctrl Pts',(-1.49524379293925,0.738802848579732,
14.4200377675521));
#56929=CARTESIAN_POINT('Ctrl Pts',(-1.53963306760386,0.637325035428461,
14.426848803303));
#56930=CARTESIAN_POINT('Ctrl Pts',(-1.55199565619263,0.60659812014485,14.4288983265017));
#56931=CARTESIAN_POINT('Ctrl Pts',(-1.56343129324813,0.575533310323967,
14.4309760522469));
#56932=CARTESIAN_POINT('Origin',(0.,0.,11.));
#56933=CARTESIAN_POINT('',(-1.56343130033034,0.575533291085225,15.1319018884674));
#56934=CARTESIAN_POINT('',(-1.56343130047997,0.575533290678746,14.9377828634576));
#56935=CARTESIAN_POINT('',(-1.56343130033213,0.575533291080363,11.));
#56936=CARTESIAN_POINT('Ctrl Pts',(-1.56343130047997,0.575533290678746,
14.9377828634576));
#56937=CARTESIAN_POINT('Ctrl Pts',(-1.56119071929035,0.581619810468057,
14.9373638967573));
#56938=CARTESIAN_POINT('Ctrl Pts',(-1.55891453933277,0.587693398516454,
14.9369460164377));
#56939=CARTESIAN_POINT('Ctrl Pts',(-1.5159297592197,0.700383605125528,14.9291951767874));
#56940=CARTESIAN_POINT('Ctrl Pts',(-1.46440746572649,0.802555128926979,
14.9222388432018));
#56941=CARTESIAN_POINT('Ctrl Pts',(-1.36459812965856,0.958359889818218,
14.9109387732747));
#56942=CARTESIAN_POINT('Ctrl Pts',(-1.32258914364437,1.01554825229322,14.9066081872519));
#56943=CARTESIAN_POINT('Ctrl Pts',(-1.26209494950135,1.08775735834899,14.9006547150445));
#56944=CARTESIAN_POINT('Ctrl Pts',(-1.2467475356055,1.10531452701706,14.8991653183197));
#56945=CARTESIAN_POINT('Ctrl Pts',(-1.22019586404586,1.1344324378979,14.8966117709185));
#56946=CARTESIAN_POINT('Ctrl Pts',(-1.20918299905693,1.14616374529065,14.895559007437));
#56947=CARTESIAN_POINT('Ctrl Pts',(-1.19310305825202,1.16280299257818,14.8940276352668));
#56948=CARTESIAN_POINT('Ctrl Pts',(-1.18817163436539,1.16784154318891,14.8935587504951));
#56949=CARTESIAN_POINT('Ctrl Pts',(-1.18316472569949,1.17289267869015,14.8930832570029));
#56950=CARTESIAN_POINT('Ctrl Pts',(-1.18312095950884,1.17293682653218,14.8930791006817));
#56951=CARTESIAN_POINT('Ctrl Pts',(-1.18303320412538,1.17302533725404,14.8930707669485));
#56952=CARTESIAN_POINT('Ctrl Pts',(-1.18298921490891,1.17306970010836,14.8930665895347));
#56953=CARTESIAN_POINT('Ctrl Pts',(-1.18290100108526,1.17315865319896,14.893058212441));
#56954=CARTESIAN_POINT('Ctrl Pts',(-1.18285677643809,1.17320324342315,14.8930540127577));
#56955=CARTESIAN_POINT('Ctrl Pts',(-1.18276807906039,1.17329266389225,14.8930455899209));
#56956=CARTESIAN_POINT('Ctrl Pts',(-1.18272360630839,1.17333749410324,14.8930413667657));
#56957=CARTESIAN_POINT('Ctrl Pts',(-1.18263439973514,1.17342740746785,14.8930328957531));
#56958=CARTESIAN_POINT('Ctrl Pts',(-1.18258966588265,1.17347249059412,14.8930286478932));
#56959=CARTESIAN_POINT('Ctrl Pts',(-1.18249992380736,1.17356292301601,14.8930201262093));
#56960=CARTESIAN_POINT('Ctrl Pts',(-1.18245491555522,1.17360827227896,14.8930158523831));
#56961=CARTESIAN_POINT('Ctrl Pts',(-1.18236461104836,1.17369925052128,14.8930072774734));
#56962=CARTESIAN_POINT('Ctrl Pts',(-1.18231931475618,1.17374487947263,14.893002976387));
#56963=CARTESIAN_POINT('Ctrl Pts',(-1.1822284201758,1.17383643098889,14.8929943456297));
#56964=CARTESIAN_POINT('Ctrl Pts',(-1.18218282186103,1.17388235351111,14.8929900159568));
#56965=CARTESIAN_POINT('Ctrl Pts',(-1.18209130887984,1.17397450641662,14.8929813266651));
#56966=CARTESIAN_POINT('Ctrl Pts',(-1.18204539417557,1.17402073676479,14.8929769670431));
#56967=CARTESIAN_POINT('Ctrl Pts',(-1.18195323366682,1.17411351995043,14.8929682164545));
#56968=CARTESIAN_POINT('Ctrl Pts',(-1.18190698782841,1.17416007274485,14.8929638254851));
#56969=CARTESIAN_POINT('Ctrl Pts',(-1.18181414989579,1.17425351584555,14.8929550107643));
#56970=CARTESIAN_POINT('Ctrl Pts',(-1.1817675577584,1.1743004061139,14.8929505870094));
#56971=CARTESIAN_POINT('Ctrl Pts',(-1.18167401163958,1.17439453960422,14.8929417052391));
#56972=CARTESIAN_POINT('Ctrl Pts',(-1.18162705761285,1.17444178278611,14.8929372472201));
#56973=CARTESIAN_POINT('Ctrl Pts',(-1.17775077340809,1.17834147038727,14.8925692199534));
#56974=CARTESIAN_POINT('Ctrl Pts',(-1.17390280303041,1.18217499251098,14.8922041882005));
#56975=CARTESIAN_POINT('Ctrl Pts',(-1.16547610263683,1.19048833884486,14.8914053733555));
#56976=CARTESIAN_POINT('Ctrl Pts',(-1.1608903355894,1.19496052488093,14.8909710563879));
#56977=CARTESIAN_POINT('Ctrl Pts',(-1.14800692105719,1.20738069019672,14.8897522600449));
#56978=CARTESIAN_POINT('Ctrl Pts',(-1.13965285726535,1.21526925761242,14.8889635410344));
#56979=CARTESIAN_POINT('Ctrl Pts',(-1.08239567901584,1.26822643349726,14.8835725626291));
#56980=CARTESIAN_POINT('Ctrl Pts',(-1.03091838467032,1.31041367479355,14.8788001175138));
#56981=CARTESIAN_POINT('Ctrl Pts',(-0.960908678429106,1.36110557287357,
14.8725330709332));
#56982=CARTESIAN_POINT('Ctrl Pts',(-0.944543885471565,1.37251255084979,
14.871082739937));
#56983=CARTESIAN_POINT('Ctrl Pts',(-0.872300961751523,1.42096496927852,
14.8647525158031));
#56984=CARTESIAN_POINT('Ctrl Pts',(-0.814417563714064,1.45491418242093,
14.8598688589706));
#56985=CARTESIAN_POINT('Ctrl Pts',(-0.689676328623525,1.51829275598098,
14.8498386804689));
#56986=CARTESIAN_POINT('Ctrl Pts',(-0.622606194331361,1.5470069473104,14.8447177880508));
#56987=CARTESIAN_POINT('Ctrl Pts',(-0.537248746449711,1.57709545681651,
14.8385413420599));
#56988=CARTESIAN_POINT('Ctrl Pts',(-0.520543116617423,1.58268796690588,
14.8373478623052));
#56989=CARTESIAN_POINT('Ctrl Pts',(-0.493524694113243,1.59125877380488,
14.8354414816637));
#56990=CARTESIAN_POINT('Ctrl Pts',(-0.483266730166625,1.59440408483508,
14.83472316307));
#56991=CARTESIAN_POINT('Ctrl Pts',(-0.463595124293845,1.60022852590215,
14.8333558154089));
#56992=CARTESIAN_POINT('Ctrl Pts',(-0.454186896777559,1.60292421659555,
14.8327062715908));
#56993=CARTESIAN_POINT('Ctrl Pts',(-0.432654068322825,1.60888909932573,
14.8312294021716));
#56994=CARTESIAN_POINT('Ctrl Pts',(-0.420515070017832,1.61210445288449,
14.8304038456708));
#56995=CARTESIAN_POINT('Ctrl Pts',(-0.388007222263089,1.62032288972042,
14.8282108778127));
#56996=CARTESIAN_POINT('Ctrl Pts',(-0.36757790448454,1.62507920377154,14.8268513350737));
#56997=CARTESIAN_POINT('Ctrl Pts',(-0.228427438951965,1.65471747580724,
14.8177044268828));
#56998=CARTESIAN_POINT('Ctrl Pts',(-0.107384922339684,1.6669557136625,14.8103389668518));
#56999=CARTESIAN_POINT('Ctrl Pts',(0.0798639467822497,1.6653906855874,14.7988961289787));
#57000=CARTESIAN_POINT('Ctrl Pts',(0.145708434319443,1.66092509836027,14.7948548845936));
#57001=CARTESIAN_POINT('Ctrl Pts',(0.233318455357688,1.64973324371481,14.7892642550525));
#57002=CARTESIAN_POINT('Ctrl Pts',(0.255466652901598,1.64644889578562,14.7878322305986));
#57003=CARTESIAN_POINT('Ctrl Pts',(0.2932835923487,1.64005964653999,14.7853447362173));
#57004=CARTESIAN_POINT('Ctrl Pts',(0.308986626402209,1.6371738235804,14.7842992041221));
#57005=CARTESIAN_POINT('Ctrl Pts',(0.33172458872782,1.63265639233715,14.7827636886263));
#57006=CARTESIAN_POINT('Ctrl Pts',(0.338794752024681,1.63120391410737,14.7822831863418));
#57007=CARTESIAN_POINT('Ctrl Pts',(0.351168740220887,1.62857791412775,14.7814365195677));
#57008=CARTESIAN_POINT('Ctrl Pts',(0.35647660217653,1.62742432616046,14.7810714803424));
#57009=CARTESIAN_POINT('Ctrl Pts',(0.368030709218323,1.62485396791104,14.7802727159857));
#57010=CARTESIAN_POINT('Ctrl Pts',(0.3742743563177,1.62342715349771,14.7798384575881));
#57011=CARTESIAN_POINT('Ctrl Pts',(0.391692190664877,1.61934096564819,14.7786199800375));
#57012=CARTESIAN_POINT('Ctrl Pts',(0.402847079646358,1.61660203742527,14.7778315246483));
#57013=CARTESIAN_POINT('Ctrl Pts',(0.478240548479853,1.59726146451807,14.7724515069581));
#57014=CARTESIAN_POINT('Ctrl Pts',(0.541459609394626,1.57695203859994,14.7676905341672));
#57015=CARTESIAN_POINT('Ctrl Pts',(0.623680596698855,1.54501033967742,14.7612952815514));
#57016=CARTESIAN_POINT('Ctrl Pts',(0.643911123140471,1.53668893507944,14.7597045007325));
#57017=CARTESIAN_POINT('Ctrl Pts',(0.729990828381493,1.49928347143604,14.7528735711166));
#57018=CARTESIAN_POINT('Ctrl Pts',(0.794085165422625,1.4663449345767,14.747633243334));
#57019=CARTESIAN_POINT('Ctrl Pts',(0.913254450216431,1.39499064206188,14.7377100375322));
#57020=CARTESIAN_POINT('Ctrl Pts',(0.968541415644979,1.35718907286088,14.733022336996));
#57021=CARTESIAN_POINT('Ctrl Pts',(1.03502487268179,1.30559429575693,14.727282732168));
#57022=CARTESIAN_POINT('Ctrl Pts',(1.04847427601915,1.2948183978652,14.726115731719));
#57023=CARTESIAN_POINT('Ctrl Pts',(1.06995899840976,1.27705015362701,14.7242412010459));
#57024=CARTESIAN_POINT('Ctrl Pts',(1.07809840911248,1.27018627867144,14.7235285748441));
#57025=CARTESIAN_POINT('Ctrl Pts',(1.09361072472019,1.25684837432017,14.7221653962301));
#57026=CARTESIAN_POINT('Ctrl Pts',(1.10099330754597,1.25038633910277,14.7215143918069));
#57027=CARTESIAN_POINT('Ctrl Pts',(1.11782159380567,1.23539179710259,14.720024968328));
#57028=CARTESIAN_POINT('Ctrl Pts',(1.12722753586224,1.2268154324332,14.7191884264979));
#57029=CARTESIAN_POINT('Ctrl Pts',(1.1573313490158,1.19872814443488,14.7164967653255));
#57030=CARTESIAN_POINT('Ctrl Pts',(1.17762879679031,1.17879412369778,14.7146597031325));
#57031=CARTESIAN_POINT('Ctrl Pts',(1.28831388571848,1.06437690692791,14.7044879638225));
#57032=CARTESIAN_POINT('Ctrl Pts',(1.36784186686909,0.960032240792337,14.6966271618862));
#57033=CARTESIAN_POINT('Ctrl Pts',(1.47061269457183,0.786088402341992,14.6842310485955));
#57034=CARTESIAN_POINT('Ctrl Pts',(1.50289085576768,0.722463439807858,14.6798120802158));
#57035=CARTESIAN_POINT('Ctrl Pts',(1.53720864387568,0.642490503140005,14.6741657065929));
#57036=CARTESIAN_POINT('Ctrl Pts',(1.54321837672034,0.627918353748305,14.673133197917));
#57037=CARTESIAN_POINT('Ctrl Pts',(1.55166361781409,0.606586833549017,14.6716133629124));
#57038=CARTESIAN_POINT('Ctrl Pts',(1.55426379402255,0.599893009906963,14.6711352490191));
#57039=CARTESIAN_POINT('Ctrl Pts',(1.55875332685467,0.588110136737703,14.670291206066));
#57040=CARTESIAN_POINT('Ctrl Pts',(1.56066120875769,0.583028350186222,14.6699263781181));
#57041=CARTESIAN_POINT('Ctrl Pts',(1.56477459095764,0.571907173541513,14.6691261307225));
#57042=CARTESIAN_POINT('Ctrl Pts',(1.56696994413406,0.565864406324,14.668690160204));
#57043=CARTESIAN_POINT('Ctrl Pts',(1.57302693945468,0.548886810765506,14.6674623491777));
#57044=CARTESIAN_POINT('Ctrl Pts',(1.57680937567146,0.53792439738774,14.6666661723987));
#57045=CARTESIAN_POINT('Ctrl Pts',(1.60410867830984,0.456041742701895,14.6606987128849));
#57046=CARTESIAN_POINT('Ctrl Pts',(1.62294263487886,0.38365791475213,14.6553132367539));
#57047=CARTESIAN_POINT('Ctrl Pts',(1.64950545813521,0.243520926872342,14.6449501419635));
#57048=CARTESIAN_POINT('Ctrl Pts',(1.65806294248567,0.176064029496761,14.6399890388297));
#57049=CARTESIAN_POINT('Ctrl Pts',(1.66681823323159,0.0416295507768519,
14.6302851313641));
#57050=CARTESIAN_POINT('Ctrl Pts',(1.66714782882214,-0.0252197761618907,
14.6255486597509));
#57051=CARTESIAN_POINT('Ctrl Pts',(1.66193482324454,-0.119563231094888,
14.6190145500985));
#57052=CARTESIAN_POINT('Ctrl Pts',(1.65971803046675,-0.147169770323015,
14.6171203253036));
#57053=CARTESIAN_POINT('Ctrl Pts',(1.65547858585899,-0.187373437147428,
14.6143861771779));
#57054=CARTESIAN_POINT('Ctrl Pts',(1.65399802776413,-0.200021731237748,
14.6135295271603));
#57055=CARTESIAN_POINT('Ctrl Pts',(1.65112401156462,-0.22235372374239,14.6120229066161));
#57056=CARTESIAN_POINT('Ctrl Pts',(1.64979002337648,-0.2320443186311,14.611371101424));
#57057=CARTESIAN_POINT('Ctrl Pts',(1.64681145788011,-0.252355934055075,
14.6100088019326));
#57058=CARTESIAN_POINT('Ctrl Pts',(1.64514929557366,-0.262973952437762,
14.6092988938812));
#57059=CARTESIAN_POINT('Ctrl Pts',(1.64047809545194,-0.291034146972347,
14.6074282852827));
#57060=CARTESIAN_POINT('Ctrl Pts',(1.63729360250342,-0.308446031978015,
14.6062731545515));
#57061=CARTESIAN_POINT('Ctrl Pts',(1.62098145371994,-0.390247601018884,
14.6008681961091));
#57062=CARTESIAN_POINT('Ctrl Pts',(1.60432849790091,-0.453878417222404,
14.596731117554));
#57063=CARTESIAN_POINT('Ctrl Pts',(1.53898268065541,-0.654327718377892,
14.5836720918014));
#57064=CARTESIAN_POINT('Ctrl Pts',(1.47618292509608,-0.785802678070321,
14.5751055504761));
#57065=CARTESIAN_POINT('Ctrl Pts',(1.38890212190533,-0.920183072215023,
14.5648178372127));
#57066=CARTESIAN_POINT('Ctrl Pts',(1.38046859518806,-0.932787442576402,
14.5638359939151));
#57067=CARTESIAN_POINT('Ctrl Pts',(1.36513844151433,-0.955035895427134,
14.5620691827171));
#57068=CARTESIAN_POINT('Ctrl Pts',(1.35830861327989,-0.964724943921282,
14.5612880730264));
#57069=CARTESIAN_POINT('Ctrl Pts',(1.34762510889843,-0.979542599537536,
14.5600739878309));
#57070=CARTESIAN_POINT('Ctrl Pts',(1.34384406736867,-0.984723442189037,
14.5596457584298));
#57071=CARTESIAN_POINT('Ctrl Pts',(1.33677558344973,-0.994292261168575,
14.5588476092693));
#57072=CARTESIAN_POINT('Ctrl Pts',(1.33349628260819,-0.998685997780765,
14.5584782392593));
#57073=CARTESIAN_POINT('Ctrl Pts',(1.3259126432943,-1.00874291108409,14.5576261863434));
#57074=CARTESIAN_POINT('Ctrl Pts',(1.3215936737399,-1.01439477285512,14.5571425144779));
#57075=CARTESIAN_POINT('Ctrl Pts',(1.3075595114807,-1.03251830603933,14.5555763780396));
#57076=CARTESIAN_POINT('Ctrl Pts',(1.29770328353408,-1.04487897427588,14.5544848699085));
#57077=CARTESIAN_POINT('Ctrl Pts',(1.23226323804921,-1.12459293804642,14.5473016490876));
#57078=CARTESIAN_POINT('Ctrl Pts',(1.17163737316485,-1.18762156472463,14.5409475611298));
#57079=CARTESIAN_POINT('Ctrl Pts',(1.01862569984769,-1.32352830155669,14.5260499413465));
#57080=CARTESIAN_POINT('Ctrl Pts',(0.922890444938109,-1.39197974819097,
14.5175642678565));
#57081=CARTESIAN_POINT('Ctrl Pts',(0.797592185649575,-1.46291159257379,
14.5076199060098));
#57082=CARTESIAN_POINT('Ctrl Pts',(0.774131366441445,-1.47546073854387,
14.5058017689212));
#57083=CARTESIAN_POINT('Ctrl Pts',(0.739184881645519,-1.49309038756018,
14.5031557354706));
#57084=CARTESIAN_POINT('Ctrl Pts',(0.727927259349844,-1.49861106184631,
14.5023126034722));
#57085=CARTESIAN_POINT('Ctrl Pts',(0.707799430191143,-1.50820130445134,
14.5008211718781));
#57086=CARTESIAN_POINT('Ctrl Pts',(0.698953886342473,-1.51232095794956,
14.5001711629913));
#57087=CARTESIAN_POINT('Ctrl Pts',(0.680198016468127,-1.52085645516787,
14.4988040741707));
#57088=CARTESIAN_POINT('Ctrl Pts',(0.670279687775431,-1.52525369967497,
14.498087655793));
#57089=CARTESIAN_POINT('Ctrl Pts',(0.643632682167299,-1.53675739529548,
14.4961797450383));
#57090=CARTESIAN_POINT('Ctrl Pts',(0.626829185090151,-1.54368764213444,
14.4949942368378));
#57091=CARTESIAN_POINT('Ctrl Pts',(0.540873073695879,-1.57750336658963,
14.489013326476));
#57092=CARTESIAN_POINT('Ctrl Pts',(0.470089132984541,-1.60002460979704,
14.4843647891147));
#57093=CARTESIAN_POINT('Ctrl Pts',(0.290731531638775,-1.64415374541834,
14.4729736319766));
#57094=CARTESIAN_POINT('Ctrl Pts',(0.181078439071984,-1.6598114896284,14.4663565762054));
#57095=CARTESIAN_POINT('Ctrl Pts',(0.0417232087857899,-1.66572979897458,
14.4576153558356));
#57096=CARTESIAN_POINT('Ctrl Pts',(0.012730862512881,-1.66620356511176,
14.455777631832));
#57097=CARTESIAN_POINT('Ctrl Pts',(-0.0355745694098858,-1.66573216374658,
14.4526623285535));
#57098=CARTESIAN_POINT('Ctrl Pts',(-0.0548860620305085,-1.66520768469757,
14.4514026535183));
#57099=CARTESIAN_POINT('Ctrl Pts',(-0.0819567641449366,-1.66400109366379,
14.4496113933152));
#57100=CARTESIAN_POINT('Ctrl Pts',(-0.0897277782912462,-1.66360015350894,
14.449094240045));
#57101=CARTESIAN_POINT('Ctrl Pts',(-0.103041778674237,-1.66281967112757,
14.448202714152));
#57102=CARTESIAN_POINT('Ctrl Pts',(-0.108586304897514,-1.66246680579926,
14.4478298041162));
#57103=CARTESIAN_POINT('Ctrl Pts',(-0.120235311393509,-1.66166691400585,
14.4470427185696));
#57104=CARTESIAN_POINT('Ctrl Pts',(-0.126339171814687,-1.66121397593284,
14.4466282442403));
#57105=CARTESIAN_POINT('Ctrl Pts',(-0.142897429857614,-1.65989348216293,
14.4454985460248));
#57106=CARTESIAN_POINT('Ctrl Pts',(-0.15334614435679,-1.65896081733869,
14.4447799016536));
#57107=CARTESIAN_POINT('Ctrl Pts',(-0.204492566660586,-1.65390811932029,
14.4412360681509));
#57108=CARTESIAN_POINT('Ctrl Pts',(-0.245034652740965,-1.64838911920957,
14.4383462639574));
#57109=CARTESIAN_POINT('Ctrl Pts',(-0.375753840304435,-1.62566566420576,
14.4288473142388));
#57110=CARTESIAN_POINT('Ctrl Pts',(-0.464723771855776,-1.60250161286187,
14.4221083930404));
#57111=CARTESIAN_POINT('Ctrl Pts',(-0.63999880388398,-1.54103410098925,
14.4086693362809));
#57112=CARTESIAN_POINT('Ctrl Pts',(-0.725887727091457,-1.50249024603493,
14.4019996520587));
#57113=CARTESIAN_POINT('Ctrl Pts',(-0.824309271557369,-1.44790007738957,
14.3943078786776));
#57114=CARTESIAN_POINT('Ctrl Pts',(-0.84038730672206,-1.43862769065992,
14.3930491349002));
#57115=CARTESIAN_POINT('Ctrl Pts',(-0.865684221334993,-1.42346981569469,
14.3910643245122));
#57116=CARTESIAN_POINT('Ctrl Pts',(-0.875005474744924,-1.41775911786363,
14.3903320151705));
#57117=CARTESIAN_POINT('Ctrl Pts',(-0.892526162237403,-1.40678639037462,
14.3889534388744));
#57118=CARTESIAN_POINT('Ctrl Pts',(-0.900736917818019,-1.40154340289076,
14.3883065097141));
#57119=CARTESIAN_POINT('Ctrl Pts',(-0.919288295974045,-1.38946703308628,
14.3868425402342));
#57120=CARTESIAN_POINT('Ctrl Pts',(-0.929599677992207,-1.38258962084153,
14.386027180012));
#57121=CARTESIAN_POINT('Ctrl Pts',(-0.956296068654092,-1.36435015586475,
14.3839110911912));
#57122=CARTESIAN_POINT('Ctrl Pts',(-0.972555847329067,-1.35280770878348,
14.3826171772229));
#57123=CARTESIAN_POINT('Ctrl Pts',(-1.09582719699795,-1.26192859892555,
14.3727562074008));
#57124=CARTESIAN_POINT('Ctrl Pts',(-1.19318199866672,-1.17030831958512,
14.3647163989273));
#57125=CARTESIAN_POINT('Ctrl Pts',(-1.3322484808992,-1.00383013736745,14.3514356915794));
#57126=CARTESIAN_POINT('Ctrl Pts',(-1.38098169462825,-0.935653117165252,
14.3462702150255));
#57127=CARTESIAN_POINT('Ctrl Pts',(-1.43088923417224,-0.853387043778903,
14.3399875984063));
#57128=CARTESIAN_POINT('Ctrl Pts',(-1.43727582983547,-0.842586264280778,
14.3391617500215));
#57129=CARTESIAN_POINT('Ctrl Pts',(-1.4468137621537,-0.82603205221215,14.3378928392095));
#57130=CARTESIAN_POINT('Ctrl Pts',(-1.45005428707857,-0.820330161884658,
14.3374552182932));
#57131=CARTESIAN_POINT('Ctrl Pts',(-1.45593387245327,-0.809840997406341,
14.3366488679771));
#57132=CARTESIAN_POINT('Ctrl Pts',(-1.4585831416257,-0.805059686090085,
14.3362807915933));
#57133=CARTESIAN_POINT('Ctrl Pts',(-1.46458789157623,-0.794095581678951,
14.3354355941896));
#57134=CARTESIAN_POINT('Ctrl Pts',(-1.46792776296666,-0.787904539393444,
14.3349575325043));
#57135=CARTESIAN_POINT('Ctrl Pts',(-1.4782510814726,-0.768474962626304,
14.3334551292887));
#57136=CARTESIAN_POINT('Ctrl Pts',(-1.48509516926469,-0.755163775220494,
14.3324228299294));
#57137=CARTESIAN_POINT('Ctrl Pts',(-1.53862939173661,-0.647501131951625,
14.3240600131066));
#57138=CARTESIAN_POINT('Ctrl Pts',(-1.57645633955487,-0.549017307145089,
14.316344318012));
#57139=CARTESIAN_POINT('Ctrl Pts',(-1.63446330171472,-0.341065839003679,
14.3006488236942));
#57140=CARTESIAN_POINT('Ctrl Pts',(-1.65350533917686,-0.231785534366187,
14.2927206925709));
#57141=CARTESIAN_POINT('Ctrl Pts',(-1.66305993220523,-0.101021954849681,
14.2837357873647));
#57142=CARTESIAN_POINT('Ctrl Pts',(-1.66417421190964,-0.0806103615335162,
14.2823466474091));
#57143=CARTESIAN_POINT('Ctrl Pts',(-1.66532187845883,-0.0488609195891628,
14.2802057277429));
#57144=CARTESIAN_POINT('Ctrl Pts',(-1.66561564446994,-0.0375351064723029,
14.2794459181799));
#57145=CARTESIAN_POINT('Ctrl Pts',(-1.66593112461483,-0.017482209441617,
14.278107286252));
#57146=CARTESIAN_POINT('Ctrl Pts',(-1.66599984091722,-0.00875640526475396,
14.2775270211396));
#57147=CARTESIAN_POINT('Ctrl Pts',(-1.66600020737263,0.0113795055583354,
14.2761929251591));
#57148=CARTESIAN_POINT('Ctrl Pts',(-1.66588320253356,0.0227892627417358,
14.2754406380613));
#57149=CARTESIAN_POINT('Ctrl Pts',(-1.66522147424093,0.0550202157232996,
14.2733252433562));
#57150=CARTESIAN_POINT('Ctrl Pts',(-1.6644035055733,0.0758341327895048,
14.2719706532173));
#57151=CARTESIAN_POINT('Ctrl Pts',(-1.65690917093362,0.204829257923058,
14.2636362407428));
#57152=CARTESIAN_POINT('Ctrl Pts',(-1.64007957644306,0.312163349893217,
14.2569890429078));
#57153=CARTESIAN_POINT('Ctrl Pts',(-1.59906991625028,0.470744190249016,
14.2469855902215));
#57154=CARTESIAN_POINT('Ctrl Pts',(-1.58254342204313,0.523615361484824,
14.2436133494779));
#57155=CARTESIAN_POINT('Ctrl Pts',(-1.56343134771032,0.575533162377876,
14.2401853336637));
#57156=CARTESIAN_POINT('',(-1.66599925405382,0.00153210873033471,14.4716226783165));
#57157=CARTESIAN_POINT('Ctrl Pts',(-1.56343129324813,0.575533310323967,
14.4309760522469));
#57158=CARTESIAN_POINT('Ctrl Pts',(-1.57677209618433,0.539293133754934,
14.4333999250567));
#57159=CARTESIAN_POINT('Ctrl Pts',(-1.58885135719543,0.502593098001554,
14.4358621957485));
#57160=CARTESIAN_POINT('Ctrl Pts',(-1.60288200634149,0.454378071893856,
14.439146856625));
#57161=CARTESIAN_POINT('Ctrl Pts',(-1.60600216048062,0.443223646242346,
14.4399101728418));
#57162=CARTESIAN_POINT('Ctrl Pts',(-1.61067217749139,0.425831462946423,
14.4411069599331));
#57163=CARTESIAN_POINT('Ctrl Pts',(-1.61230274453565,0.419615484318913,
14.4415359978152));
#57164=CARTESIAN_POINT('Ctrl Pts',(-1.61524443112633,0.408130988191647,
14.4423313485267));
#57165=CARTESIAN_POINT('Ctrl Pts',(-1.61656581024057,0.402865304878655,
14.4426970737048));
#57166=CARTESIAN_POINT('Ctrl Pts',(-1.61957647236361,0.390614509447594,
14.4435503466289));
#57167=CARTESIAN_POINT('Ctrl Pts',(-1.62124631214617,0.38362486283522,14.4440389641873));
#57168=CARTESIAN_POINT('Ctrl Pts',(-1.62467717231388,0.368841335600024,
14.4450758717672));
#57169=CARTESIAN_POINT('Ctrl Pts',(-1.62642744286349,0.361045166246974,
14.4456247079493));
#57170=CARTESIAN_POINT('Ctrl Pts',(-1.63298720533843,0.330810243027963,
14.4477602133763));
#57171=CARTESIAN_POINT('Ctrl Pts',(-1.63738871873334,0.30828670492056,14.4493659728305));
#57172=CARTESIAN_POINT('Ctrl Pts',(-1.65765738191466,0.191837047830531,
14.4577209459689));
#57173=CARTESIAN_POINT('Ctrl Pts',(-1.66591168597341,0.0967731178363305,
14.464706639791));
#57174=CARTESIAN_POINT('Ctrl Pts',(-1.66599929514542,0.00153250610393629,
14.4716227213688));
#57175=CARTESIAN_POINT('Ctrl Pts',(-1.6659992955061,0.00153211396245487,
14.4716227498449));
#57176=CARTESIAN_POINT('Ctrl Pts',(-1.66607010972176,-0.0754702737889355,
14.4772144272921));
#57177=CARTESIAN_POINT('Ctrl Pts',(-1.66080232591833,-0.152394421586609,
14.4827483996111));
#57178=CARTESIAN_POINT('Ctrl Pts',(-1.64568388868304,-0.261490397897914,
14.4904529449018));
#57179=CARTESIAN_POINT('Ctrl Pts',(-1.64016079294015,-0.294152219386785,
14.4927418217603));
#57180=CARTESIAN_POINT('Ctrl Pts',(-1.63117691918578,-0.339085851975443,
14.4958670201869));
#57181=CARTESIAN_POINT('Ctrl Pts',(-1.62854405384367,-0.351513352372362,
14.4967288697825));
#57182=CARTESIAN_POINT('Ctrl Pts',(-1.62317579314133,-0.375496087778437,
14.4983875187229));
#57183=CARTESIAN_POINT('Ctrl Pts',(-1.62045850316515,-0.387054543381548,
14.4991848400579));
#57184=CARTESIAN_POINT('Ctrl Pts',(-1.61552105335458,-0.407092784463793,
14.5005638129027));
#57185=CARTESIAN_POINT('Ctrl Pts',(-1.61335713857959,-0.415585800317818,
14.5011472417712));
#57186=CARTESIAN_POINT('Ctrl Pts',(-1.60833774361406,-0.434655862903503,
14.502455117978));
#57187=CARTESIAN_POINT('Ctrl Pts',(-1.60544473227513,-0.445222683556907,
14.5031783258944));
#57188=CARTESIAN_POINT('Ctrl Pts',(-1.59734023988666,-0.473717972479032,
14.5051250615301));
#57189=CARTESIAN_POINT('Ctrl Pts',(-1.59193118357728,-0.491588966312082,
14.5063421613897));
#57190=CARTESIAN_POINT('Ctrl Pts',(-1.5599033965559,-0.591327103316351,
14.5131199682385));
#57191=CARTESIAN_POINT('Ctrl Pts',(-1.52726977317752,-0.671130514199535,
14.5184774713513));
#57192=CARTESIAN_POINT('Ctrl Pts',(-1.44380304531921,-0.837225440257637,
14.5298868643198));
#57193=CARTESIAN_POINT('Ctrl Pts',(-1.39107945833932,-0.922176310024921,
14.535889535982));
#57194=CARTESIAN_POINT('Ctrl Pts',(-1.31356270904562,-1.02516201649674,
14.5439815501698));
#57195=CARTESIAN_POINT('Ctrl Pts',(-1.29544271213704,-1.04796570903423,
14.5458315163021));
#57196=CARTESIAN_POINT('Ctrl Pts',(-1.26553669003437,-1.08364051546153,
14.5488415248341));
#57197=CARTESIAN_POINT('Ctrl Pts',(-1.25412936494299,-1.09682239132879,
14.5499802779102));
#57198=CARTESIAN_POINT('Ctrl Pts',(-1.23743114165975,-1.11551713415926,
14.5516380902831));
#57199=CARTESIAN_POINT('Ctrl Pts',(-1.23230544303942,-1.12117688005384,
14.5521457791724));
#57200=CARTESIAN_POINT('Ctrl Pts',(-1.22339861173999,-1.13087685248107,
14.5530263542751));
#57201=CARTESIAN_POINT('Ctrl Pts',(-1.21963595220224,-1.13493381389021,
14.5533978659125));
#57202=CARTESIAN_POINT('Ctrl Pts',(-1.21162257271466,-1.14348809910577,
14.5541882018034));
#57203=CARTESIAN_POINT('Ctrl Pts',(-1.20736705408819,-1.14798043758478,
14.5546073679631));
#57204=CARTESIAN_POINT('Ctrl Pts',(-1.19561685918445,-1.16024692810146,
14.5557630124033));
#57205=CARTESIAN_POINT('Ctrl Pts',(-1.18807162549734,-1.16797191981294,
14.5565031710568));
#57206=CARTESIAN_POINT('Ctrl Pts',(-1.14843634436777,-1.20777001811595,
14.5603787522978));
#57207=CARTESIAN_POINT('Ctrl Pts',(-1.11512370828706,-1.23859306335655,
14.5635936987366));
#57208=CARTESIAN_POINT('Ctrl Pts',(-0.996874982331963,-1.33936423712399,
14.5747501486809));
#57209=CARTESIAN_POINT('Ctrl Pts',(-0.906290141437564,-1.40224691533985,
14.5828521166776));
#57210=CARTESIAN_POINT('Ctrl Pts',(-0.746775929912785,-1.49102119349974,
14.5959362552252));
#57211=CARTESIAN_POINT('Ctrl Pts',(-0.681144875635934,-1.52212442034724,
14.6010332013231));
#57212=CARTESIAN_POINT('Ctrl Pts',(-0.597327296600504,-1.55533460225163,
14.6071856990013));
#57213=CARTESIAN_POINT('Ctrl Pts',(-0.580866269635608,-1.56155692892208,
14.6083778599861));
#57214=CARTESIAN_POINT('Ctrl Pts',(-0.554218026583178,-1.57115034546383,
14.6102826792893));
#57215=CARTESIAN_POINT('Ctrl Pts',(-0.544091821678499,-1.57468572354225,
14.6110007388934));
#57216=CARTESIAN_POINT('Ctrl Pts',(-0.524660124979875,-1.58126011809069,
14.6123679357983));
#57217=CARTESIAN_POINT('Ctrl Pts',(-0.515360646064193,-1.58431537872759,
14.6130175846647));
#57218=CARTESIAN_POINT('Ctrl Pts',(-0.494062087273214,-1.59110545340586,
14.6144951605525));
#57219=CARTESIAN_POINT('Ctrl Pts',(-0.482046500779604,-1.5947868495233,
14.6153213128614));
#57220=CARTESIAN_POINT('Ctrl Pts',(-0.44983851909473,-1.60425761860508,
14.6175169116141));
#57221=CARTESIAN_POINT('Ctrl Pts',(-0.429575964593264,-1.60980177473706,
14.6188784592535));
#57222=CARTESIAN_POINT('Ctrl Pts',(-0.291734405852252,-1.64472928905196,
14.628020198793));
#57223=CARTESIAN_POINT('Ctrl Pts',(-0.171356548710252,-1.66159085754469,
14.6353794512661));
#57224=CARTESIAN_POINT('Ctrl Pts',(0.0446280021943476,-1.66810241068831,
14.6485837883545));
#57225=CARTESIAN_POINT('Ctrl Pts',(0.139517854804287,-1.66285503701495,
14.6543987134009));
#57226=CARTESIAN_POINT('Ctrl Pts',(0.245195739703589,-1.64790055934746,
14.6613776387719));
#57227=CARTESIAN_POINT('Ctrl Pts',(0.256942896019237,-1.64610981790285,
14.6621605931074));
#57228=CARTESIAN_POINT('Ctrl Pts',(0.275005595981684,-1.64315828226117,
14.6633769556955));
#57229=CARTESIAN_POINT('Ctrl Pts',(0.281335546297896,-1.64208633308998,
14.6638055901363));
#57230=CARTESIAN_POINT('Ctrl Pts',(0.293058904599432,-1.64003125986257,
14.6646041022298));
#57231=CARTESIAN_POINT('Ctrl Pts',(0.298453846172952,-1.63905806894606,
14.6649734258042));
#57232=CARTESIAN_POINT('Ctrl Pts',(0.310829805629302,-1.63676244908864,
14.6658248727309));
#57233=CARTESIAN_POINT('Ctrl Pts',(0.317807245887715,-1.63542197387879,
14.6663079795765));
#57234=CARTESIAN_POINT('Ctrl Pts',(0.340235789932005,-1.63096415120732,
14.6678703255545));
#57235=CARTESIAN_POINT('Ctrl Pts',(0.355650766555677,-1.62767224664835,
14.6689585490329));
#57236=CARTESIAN_POINT('Ctrl Pts',(0.454686699188658,-1.60504894353253,
14.6760334601717));
#57237=CARTESIAN_POINT('Ctrl Pts',(0.536747511112746,-1.57950037386838,
14.6822739848453));
#57238=CARTESIAN_POINT('Ctrl Pts',(0.684976868919276,-1.52046077225588,
14.6938884379796));
#57239=CARTESIAN_POINT('Ctrl Pts',(0.751604377672313,-1.48865260034702,
14.6992492185595));
#57240=CARTESIAN_POINT('Ctrl Pts',(0.851687623457646,-1.43243438213573,
14.7074235982992));
#57241=CARTESIAN_POINT('Ctrl Pts',(0.886714250555539,-1.41102032754759,
14.7103106604339));
#57242=CARTESIAN_POINT('Ctrl Pts',(0.945366705111057,-1.37211465523097,
14.7151868772352));
#57243=CARTESIAN_POINT('Ctrl Pts',(0.96938522592302,-1.35525248817611,14.7171966095338));
#57244=CARTESIAN_POINT('Ctrl Pts',(1.00340357305664,-1.33000257181772,14.7200637224803));
#57245=CARTESIAN_POINT('Ctrl Pts',(1.01376883397787,-1.32211888249016,14.7209402153563));
#57246=CARTESIAN_POINT('Ctrl Pts',(1.03178822823877,-1.3080770321896,14.7224694398955));
#57247=CARTESIAN_POINT('Ctrl Pts',(1.03948219938889,-1.3019712878299,14.7231241913594));
#57248=CARTESIAN_POINT('Ctrl Pts',(1.05537873580484,-1.28912544750986,14.7244809852469));
#57249=CARTESIAN_POINT('Ctrl Pts',(1.06357179766593,-1.28237425715964,14.7251825424673));
#57250=CARTESIAN_POINT('Ctrl Pts',(1.08478171138486,-1.26455390456639,14.72700512477));
#57251=CARTESIAN_POINT('Ctrl Pts',(1.0976940079385,-1.2533618149281,14.728121096596));
#57252=CARTESIAN_POINT('Ctrl Pts',(1.15280558425405,-1.20408724515266,14.7329161397536));
#57253=CARTESIAN_POINT('Ctrl Pts',(1.19321511787951,-1.16405563247742,14.7365130449766));
#57254=CARTESIAN_POINT('Ctrl Pts',(1.30299594852364,-1.04356418656821,14.746664105659));
#57255=CARTESIAN_POINT('Ctrl Pts',(1.36682418255457,-0.958444574142309,
14.7530409311685));
#57256=CARTESIAN_POINT('Ctrl Pts',(1.45322893397506,-0.816852665890636,
14.7632758235878));
#57257=CARTESIAN_POINT('Ctrl Pts',(1.48157122851813,-0.764243275375606,
14.7670122975575));
#57258=CARTESIAN_POINT('Ctrl Pts',(1.51322103877211,-0.697086288838903,
14.7718403478763));
#57259=CARTESIAN_POINT('Ctrl Pts',(1.51924403710868,-0.683860166143343,
14.7727939521289));
#57260=CARTESIAN_POINT('Ctrl Pts',(1.52789137805668,-0.664192950392203,
14.7742184653774));
#57261=CARTESIAN_POINT('Ctrl Pts',(1.53064983270592,-0.657811085194333,
14.7746817109449));
#57262=CARTESIAN_POINT('Ctrl Pts',(1.53529815767669,-0.646869330088177,
14.7754779692443));
#57263=CARTESIAN_POINT('Ctrl Pts',(1.53720783634039,-0.642318013160207,
14.7758097839184));
#57264=CARTESIAN_POINT('Ctrl Pts',(1.54154432496139,-0.631852795903634,
14.7765742015799));
#57265=CARTESIAN_POINT('Ctrl Pts',(1.54395729000703,-0.625933498633533,
14.7770075975889));
#57266=CARTESIAN_POINT('Ctrl Pts',(1.55058973455484,-0.609391597688285,
14.7782213233504));
#57267=CARTESIAN_POINT('Ctrl Pts',(1.55473395352052,-0.598739475897147,
14.7790058385461));
#57268=CARTESIAN_POINT('Ctrl Pts',(1.58142081902552,-0.527999024511015,
14.784231251723));
#57269=CARTESIAN_POINT('Ctrl Pts',(1.60058250564716,-0.466699680377038,
14.7888308202969));
#57270=CARTESIAN_POINT('Ctrl Pts',(1.62185328582796,-0.381704045948198,
14.7951788000757));
#57271=CARTESIAN_POINT('Ctrl Pts',(1.6270659334762,-0.358834895795534,14.7968841874953));
#57272=CARTESIAN_POINT('Ctrl Pts',(1.64314462818012,-0.280716527768322,
14.8026886661328));
#57273=CARTESIAN_POINT('Ctrl Pts',(1.65169277482749,-0.225027615424539,
14.8067897584466));
#57274=CARTESIAN_POINT('Ctrl Pts',(1.66568768263496,-0.0877869598424337,
14.8167223612981));
#57275=CARTESIAN_POINT('Ctrl Pts',(1.66798950416059,-0.00605385503372676,
14.8224843318956));
#57276=CARTESIAN_POINT('Ctrl Pts',(1.66346729498448,0.0935920234690066,
14.8292964695389));
#57277=CARTESIAN_POINT('Ctrl Pts',(1.6623535857015,0.111640087663716,14.8305221483701));
#57278=CARTESIAN_POINT('Ctrl Pts',(1.66010340728635,0.140463327788435,14.8324672649783));
#57279=CARTESIAN_POINT('Ctrl Pts',(1.65915530277145,0.151251314715752,14.8331925215497));
#57280=CARTESIAN_POINT('Ctrl Pts',(1.65715260023084,0.171745637690258,14.8345653222362));
#57281=CARTESIAN_POINT('Ctrl Pts',(1.65611774196164,0.181453399535798,14.8352134549247));
#57282=CARTESIAN_POINT('Ctrl Pts',(1.65355466122131,0.20364463730525,14.8366904292869));
#57283=CARTESIAN_POINT('Ctrl Pts',(1.65197028678698,0.216121127977426,14.8375174745102));
#57284=CARTESIAN_POINT('Ctrl Pts',(1.64742325238133,0.24894884672207,14.8396855622441));
#57285=CARTESIAN_POINT('Ctrl Pts',(1.6442247389431,0.269265608783011,14.8410192153679));
#57286=CARTESIAN_POINT('Ctrl Pts',(1.61440148967487,0.438268647032832,14.8520590300703));
#57287=CARTESIAN_POINT('Ctrl Pts',(1.56804810957986,0.58275060981159,14.8610656696918));
#57288=CARTESIAN_POINT('Ctrl Pts',(1.47639288644112,0.774325470044577,14.8741575439071));
#57289=CARTESIAN_POINT('Ctrl Pts',(1.44689846356851,0.828129881449129,14.877988942799));
#57290=CARTESIAN_POINT('Ctrl Pts',(1.40673678012072,0.892672452180107,14.8829308125711));
#57291=CARTESIAN_POINT('Ctrl Pts',(1.39879874257973,0.905060504493886,14.8838959881868));
#57292=CARTESIAN_POINT('Ctrl Pts',(1.38685089555989,0.92317355319401,14.8853345186604));
#57293=CARTESIAN_POINT('Ctrl Pts',(1.38296720620833,0.928981441149657,14.8857999914108));
#57294=CARTESIAN_POINT('Ctrl Pts',(1.37627571890856,0.93885331345002,14.8865987089707));
#57295=CARTESIAN_POINT('Ctrl Pts',(1.37348619677984,0.942929512160158,14.8869307339714));
#57296=CARTESIAN_POINT('Ctrl Pts',(1.36705889698197,0.952232388447557,14.8876936766206));
#57297=CARTESIAN_POINT('Ctrl Pts',(1.36340933394882,0.957450538738162,14.8881253699619));
#57298=CARTESIAN_POINT('Ctrl Pts',(1.35318867830356,0.971887112798959,14.8893298520007));
#57299=CARTESIAN_POINT('Ctrl Pts',(1.34655354777308,0.98105947045385,14.8901067286173));
#57300=CARTESIAN_POINT('Ctrl Pts',(1.30456944878151,1.03786967665884,14.8949877666505));
#57301=CARTESIAN_POINT('Ctrl Pts',(1.26679399989211,1.08365416496005,14.8992276229039));
#57302=CARTESIAN_POINT('Ctrl Pts',(1.12479950994088,1.23816136749632,14.9144043264441));
#57303=CARTESIAN_POINT('Ctrl Pts',(1.00835667963723,1.33471011059004,14.9254652015533));
#57304=CARTESIAN_POINT('Ctrl Pts',(0.856888718317735,1.4290109501614,14.9378058044863));
#57305=CARTESIAN_POINT('Ctrl Pts',(0.832896287738831,1.44312664259181,14.9397099163805));
#57306=CARTESIAN_POINT('Ctrl Pts',(0.797404173761675,1.46282787328466,14.9424555094821));
#57307=CARTESIAN_POINT('Ctrl Pts',(0.786177172158093,1.46889219239937,14.9433139155349));
#57308=CARTESIAN_POINT('Ctrl Pts',(0.766218821745587,1.47937840691593,14.9448225498853));
#57309=CARTESIAN_POINT('Ctrl Pts',(0.757516225975488,1.48385340517615,14.9454746289481));
#57310=CARTESIAN_POINT('Ctrl Pts',(0.739184617367353,1.49307647092038,14.9468364560966));
#57311=CARTESIAN_POINT('Ctrl Pts',(0.729548093566089,1.49780867764991,14.947545627002));
#57312=CARTESIAN_POINT('Ctrl Pts',(0.703954974341639,1.51007108562996,14.9494118959159));
#57313=CARTESIAN_POINT('Ctrl Pts',(0.687923069819701,1.51744165564607,14.9505634720172));
#57314=CARTESIAN_POINT('Ctrl Pts',(0.611746011949572,1.55100811763459,14.9559580423633));
#57315=CARTESIAN_POINT('Ctrl Pts',(0.550201463549296,1.5738930052545,14.9600886250358));
#57316=CARTESIAN_POINT('Ctrl Pts',(0.348572303948392,1.63558847049831,14.973150647575));
#57317=CARTESIAN_POINT('Ctrl Pts',(0.204742883871241,1.65973554132485,14.9817245848424));
#57318=CARTESIAN_POINT('Ctrl Pts',(0.0444306400704773,1.66547684905283,
14.9920227524561));
#57319=CARTESIAN_POINT('Ctrl Pts',(0.0292284189010689,1.66581297884413,
14.9930071325472));
#57320=CARTESIAN_POINT('Ctrl Pts',(0.00214577637284439,1.66604096752735,
14.994778094679));
#57321=CARTESIAN_POINT('Ctrl Pts',(-0.00973308183318889,1.66601391264209,
14.9955607924571));
#57322=CARTESIAN_POINT('Ctrl Pts',(-0.0280289915889216,1.66577657063434,
14.9967768402769));
#57323=CARTESIAN_POINT('Ctrl Pts',(-0.0344471001956311,1.66565620746902,
14.9972054203839));
#57324=CARTESIAN_POINT('Ctrl Pts',(-0.0463449329190276,1.66536428552764,
14.9980038874605));
#57325=CARTESIAN_POINT('Ctrl Pts',(-0.0518246988095145,1.66520276653938,
14.9983732209639));
#57326=CARTESIAN_POINT('Ctrl Pts',(-0.0644056767335511,1.66476977660643,
14.999224762513));
#57327=CARTESIAN_POINT('Ctrl Pts',(-0.0715060294726993,1.66447991379128,
14.9997079548539));
#57328=CARTESIAN_POINT('Ctrl Pts',(-0.0943558767970944,1.66340062495418,
15.0012708583614));
#57329=CARTESIAN_POINT('Ctrl Pts',(-0.110095547572428,1.66243303501844,
15.0023595624817));
#57330=CARTESIAN_POINT('Ctrl Pts',(-0.211658466737472,1.6547409105016,15.0094531284478));
#57331=CARTESIAN_POINT('Ctrl Pts',(-0.296857512588311,1.64159666458377,
15.0157133058776));
#57332=CARTESIAN_POINT('Ctrl Pts',(-0.452265443450762,1.60512403026894,
15.027333341642));
#57333=CARTESIAN_POINT('Ctrl Pts',(-0.522693418721993,1.58359092005621,
15.0326803090264));
#57334=CARTESIAN_POINT('Ctrl Pts',(-0.629789569983826,1.54291968285747,
15.0408377073797));
#57335=CARTESIAN_POINT('Ctrl Pts',(-0.66756018517107,1.52695772950736,15.0437211977033));
#57336=CARTESIAN_POINT('Ctrl Pts',(-0.731268861183344,1.49721781344463,
15.0485921042314));
#57337=CARTESIAN_POINT('Ctrl Pts',(-0.757500967938394,1.48411852627406,
15.0506000378084));
#57338=CARTESIAN_POINT('Ctrl Pts',(-0.794863927705322,1.46421200444325,
15.0534650888684));
#57339=CARTESIAN_POINT('Ctrl Pts',(-0.806280771680242,1.45795637501331,
15.0543412802621));
#57340=CARTESIAN_POINT('Ctrl Pts',(-0.826180589174423,1.44674741810042,
15.0558701603443));
#57341=CARTESIAN_POINT('Ctrl Pts',(-0.834695133932594,1.4418517601343,15.0565248659942));
#57342=CARTESIAN_POINT('Ctrl Pts',(-0.852323529573463,1.43150736511785,
15.0578817356757));
#57343=CARTESIAN_POINT('Ctrl Pts',(-0.86142960536506,1.42604620516515,15.0585834130294));
#57344=CARTESIAN_POINT('Ctrl Pts',(-0.885058895574051,1.41156614784214,
15.06040668276));
#57345=CARTESIAN_POINT('Ctrl Pts',(-0.899496837419093,1.40240996615437,
15.0615232146471));
#57346=CARTESIAN_POINT('Ctrl Pts',(-0.961399203605009,1.36180369540898,
15.0663249862226));
#57347=CARTESIAN_POINT('Ctrl Pts',(-1.00737760771395,1.32815252042373,15.0699277580662));
#57348=CARTESIAN_POINT('Ctrl Pts',(-1.1338423176092,1.22524081725169,15.0800808614251));
#57349=CARTESIAN_POINT('Ctrl Pts',(-1.20955033757919,1.15056556981926,15.0864545188659));
#57350=CARTESIAN_POINT('Ctrl Pts',(-1.31593705187389,1.0234383871181,15.0966832876255));
#57351=CARTESIAN_POINT('Ctrl Pts',(-1.35174151264472,0.975658659439617,
15.1004166933089));
#57352=CARTESIAN_POINT('Ctrl Pts',(-1.39297758113941,0.913991517523786,
15.1052410645524));
#57353=CARTESIAN_POINT('Ctrl Pts',(-1.40089400857755,0.901810943209442,
15.1061942916805));
#57354=CARTESIAN_POINT('Ctrl Pts',(-1.41236141940444,0.883651256967204,
15.10761834808));
#57355=CARTESIAN_POINT('Ctrl Pts',(-1.41603611859186,0.877750550830753,
15.1080815210105));
#57356=CARTESIAN_POINT('Ctrl Pts',(-1.4222566277471,0.867621142475052,15.1088776992591));
#57357=CARTESIAN_POINT('Ctrl Pts',(-1.4248207428189,0.863403852107385,15.1092095072288));
#57358=CARTESIAN_POINT('Ctrl Pts',(-1.43066312924325,0.853697769946753,
15.109973973578));
#57359=CARTESIAN_POINT('Ctrl Pts',(-1.43392850152452,0.848201580326376,
15.1104074255489));
#57360=CARTESIAN_POINT('Ctrl Pts',(-1.44294536763373,0.83282374672994,15.1116214574555));
#57361=CARTESIAN_POINT('Ctrl Pts',(-1.44862676022256,0.822901706542715,
15.1124062260964));
#57362=CARTESIAN_POINT('Ctrl Pts',(-1.48558600484684,0.756786739895782,
15.117641165683));
#57363=CARTESIAN_POINT('Ctrl Pts',(-1.51368652309156,0.698887130427848,
15.1222506589328));
#57364=CARTESIAN_POINT('Ctrl Pts',(-1.54716141035095,0.618362642153892,
15.128569107624));
#57365=CARTESIAN_POINT('Ctrl Pts',(-1.55551768061514,0.597030571873839,
15.1302347640674));
#57366=CARTESIAN_POINT('Ctrl Pts',(-1.56343130033034,0.575533291085225,
15.1319018884674));
#57367=CARTESIAN_POINT('Origin',(0.,0.,11.));
#57368=CARTESIAN_POINT('',(-1.5634313003304,0.575533291085054,15.8337663187435));
#57369=CARTESIAN_POINT('',(-1.56343131209646,0.575533259122642,15.6388155835246));
#57370=CARTESIAN_POINT('',(-1.56343130033213,0.575533291080363,11.));
#57371=CARTESIAN_POINT('',(-1.66599941198745,-0.00147660206947851,14.9787479457986));
#57372=CARTESIAN_POINT('Ctrl Pts',(-1.56343131209642,0.575533259122747,
15.6388155835246));
#57373=CARTESIAN_POINT('Ctrl Pts',(-1.55177222105231,0.607205082983509,
15.6363706320662));
#57374=CARTESIAN_POINT('Ctrl Pts',(-1.53914439133288,0.638539834474232,
15.6339365106143));
#57375=CARTESIAN_POINT('Ctrl Pts',(-1.49910450291894,0.729778033426274,
15.6268187785043));
#57376=CARTESIAN_POINT('Ctrl Pts',(-1.46909540592463,0.788448442551207,
15.62220506387));
#57377=CARTESIAN_POINT('Ctrl Pts',(-1.42670587109312,0.860453277364878,
15.6165020785214));
#57378=CARTESIAN_POINT('Ctrl Pts',(-1.417480561216,0.875567464976233,15.6153023522287));
#57379=CARTESIAN_POINT('Ctrl Pts',(-1.40227040247757,0.899616165400458,
15.6133884546029));
#57380=CARTESIAN_POINT('Ctrl Pts',(-1.39643717372203,0.908644460681454,
15.6126687886807));
#57381=CARTESIAN_POINT('Ctrl Pts',(-1.38512938178619,0.925779817708487,
15.611300407942));
#57382=CARTESIAN_POINT('Ctrl Pts',(-1.37967001471364,0.933896317921136,
15.6106511638684));
#57383=CARTESIAN_POINT('Ctrl Pts',(-1.36694101323808,0.95246540811069,15.6091630140976));
#57384=CARTESIAN_POINT('Ctrl Pts',(-1.3596223510197,0.962883775379662,15.6083260047986));
#57385=CARTESIAN_POINT('Ctrl Pts',(-1.33601814616774,0.995679371640372,
15.6056835536315));
#57386=CARTESIAN_POINT('Ctrl Pts',(-1.31929361415321,1.01773591836838,15.603894971513));
#57387=CARTESIAN_POINT('Ctrl Pts',(-1.26075086499363,1.09107309347279,15.5978938959737));
#57388=CARTESIAN_POINT('Ctrl Pts',(-1.21642957067679,1.14027786025765,15.5937772486746));
#57389=CARTESIAN_POINT('Ctrl Pts',(-1.12508377966516,1.23028242452983,15.585892447453));
#57390=CARTESIAN_POINT('Ctrl Pts',(-1.07847250180136,1.27134001546368,15.5821242435449));
#57391=CARTESIAN_POINT('Ctrl Pts',(-0.965883369033863,1.3598569092897,15.5733467078555));
#57392=CARTESIAN_POINT('Ctrl Pts',(-0.89851651284192,1.40527791427588,15.5683244154611));
#57393=CARTESIAN_POINT('Ctrl Pts',(-0.818016099911846,1.45139286509422,
15.5622567743807));
#57394=CARTESIAN_POINT('Ctrl Pts',(-0.807852211388698,1.45707459466636,
15.5614894830119));
#57395=CARTESIAN_POINT('Ctrl Pts',(-0.79197609607278,1.46573235472965,15.5602877832376));
#57396=CARTESIAN_POINT('Ctrl Pts',(-0.786304525505393,1.46878271440629,
15.5598578658583));
#57397=CARTESIAN_POINT('Ctrl Pts',(-0.775775068640214,1.47436734362632,
15.5590582918021));
#57398=CARTESIAN_POINT('Ctrl Pts',(-0.770922193799072,1.47691062323338,
15.558689203669));
#57399=CARTESIAN_POINT('Ctrl Pts',(-0.759666171328936,1.48273905322255,
15.5578318365845));
#57400=CARTESIAN_POINT('Ctrl Pts',(-0.75325422162104,1.48600668390545,15.557342508434));
#57401=CARTESIAN_POINT('Ctrl Pts',(-0.732654983581548,1.4963368049058,15.5557679788455));
#57402=CARTESIAN_POINT('Ctrl Pts',(-0.718388500173889,1.50323819662533,
15.5546737346606));
#57403=CARTESIAN_POINT('Ctrl Pts',(-0.638644111847153,1.54042003960233,
15.548545157333));
#57404=CARTESIAN_POINT('Ctrl Pts',(-0.571356938738306,1.5666235683454,15.5433321522475));
#57405=CARTESIAN_POINT('Ctrl Pts',(-0.375360212018787,1.6286402808487,15.5283853722561));
#57406=CARTESIAN_POINT('Ctrl Pts',(-0.243726813805456,1.6534734145658,15.5186716264791));
#57407=CARTESIAN_POINT('Ctrl Pts',(-0.0846055884013189,1.66405309198635,
15.5076655187007));
#57408=CARTESIAN_POINT('Ctrl Pts',(-0.0586479894757322,1.66517006442747,
15.5058909770305));
#57409=CARTESIAN_POINT('Ctrl Pts',(-0.020253121680027,1.66592320889176,
15.5032956296234));
#57410=CARTESIAN_POINT('Ctrl Pts',(-0.00783005576397834,1.66602792041299,
15.5024604136669));
#57411=CARTESIAN_POINT('Ctrl Pts',(0.0143379179613808,1.6659668010121,15.5009777929786));
#57412=CARTESIAN_POINT('Ctrl Pts',(0.0240822686485433,1.66585443818851,
15.5003287521227));
#57413=CARTESIAN_POINT('Ctrl Pts',(0.0447369180402899,1.66543499473685,
15.498958433904));
#57414=CARTESIAN_POINT('Ctrl Pts',(0.0556463542761696,1.66510618470226,
15.4982378649583));
#57415=CARTESIAN_POINT('Ctrl Pts',(0.0850155802516916,1.66393202986098,
15.4963061553773));
#57416=CARTESIAN_POINT('Ctrl Pts',(0.103466176324512,1.66288671999325,15.4951012696376));
#57417=CARTESIAN_POINT('Ctrl Pts',(0.213170929633009,1.65483838318132,15.4879820355488));
#57418=CARTESIAN_POINT('Ctrl Pts',(0.303744371465109,1.64063233264572,15.482301009781));
#57419=CARTESIAN_POINT('Ctrl Pts',(0.477586682812849,1.5984668254241,15.4713379173617));
#57420=CARTESIAN_POINT('Ctrl Pts',(0.560715860005859,1.57123566220749,15.4660639019779));
#57421=CARTESIAN_POINT('Ctrl Pts',(0.684874659348441,1.51945037555949,15.4576672169387));
#57422=CARTESIAN_POINT('Ctrl Pts',(0.727630959862287,1.49944491071121,15.4546724292722));
#57423=CARTESIAN_POINT('Ctrl Pts',(0.77914325382367,1.47262031195348,15.4508662246192));
#57424=CARTESIAN_POINT('Ctrl Pts',(0.788760346589713,1.46749170126251,15.4501468372356));
#57425=CARTESIAN_POINT('Ctrl Pts',(0.803776381540334,1.45929369490174,15.4490086248032));
#57426=CARTESIAN_POINT('Ctrl Pts',(0.809209862197859,1.45628773093741,15.4485936559644));
#57427=CARTESIAN_POINT('Ctrl Pts',(0.819447164821849,1.45054916756653,15.4478056614391));
#57428=CARTESIAN_POINT('Ctrl Pts',(0.824254351564816,1.44782295315993,15.4474330320016));
#57429=CARTESIAN_POINT('Ctrl Pts',(0.835631869106725,1.4412955968682,15.4465449991739));
#57430=CARTESIAN_POINT('Ctrl Pts',(0.842189891359466,1.43747340827862,15.4460282847164));
#57431=CARTESIAN_POINT('Ctrl Pts',(0.864323501526135,1.42436990535316,15.4442684418211));
#57432=CARTESIAN_POINT('Ctrl Pts',(0.87977299415682,1.41487955477236,15.443013163481));
#57433=CARTESIAN_POINT('Ctrl Pts',(0.917478723021633,1.39086127692496,15.4398883065606));
#57434=CARTESIAN_POINT('Ctrl Pts',(0.939547653743055,1.37604954436624,15.4380054516535));
#57435=CARTESIAN_POINT('Ctrl Pts',(1.03569190375755,1.30813035111853,15.4295903083518));
#57436=CARTESIAN_POINT('Ctrl Pts',(1.10568968850922,1.24952496514812,15.4229001777864));
#57437=CARTESIAN_POINT('Ctrl Pts',(1.23897747256315,1.11791780119275,15.409335103788));
#57438=CARTESIAN_POINT('Ctrl Pts',(1.30144265605379,1.04453726580949,15.4024985045623));
#57439=CARTESIAN_POINT('Ctrl Pts',(1.36809146079988,0.950911287168516,15.3946396863951));
#57440=CARTESIAN_POINT('Ctrl Pts',(1.37869152558984,0.935476481840212,15.3933691609651));
#57441=CARTESIAN_POINT('Ctrl Pts',(1.3951422524286,0.910635306285139,15.3913629782561));
#57442=CARTESIAN_POINT('Ctrl Pts',(1.40116292582691,0.901344013735505,15.3906209970282));
#57443=CARTESIAN_POINT('Ctrl Pts',(1.41224566449318,0.883861348935565,15.3892401792337));
#57444=CARTESIAN_POINT('Ctrl Pts',(1.41733016613232,0.875684822208499,15.3886005318789));
#57445=CARTESIAN_POINT('Ctrl Pts',(1.42865773017875,0.857111511584895,15.3871611082498));
#57446=CARTESIAN_POINT('Ctrl Pts',(1.43485877840326,0.846689643441299,15.3863628891065));
#57447=CARTESIAN_POINT('Ctrl Pts',(1.45319682672366,0.815089420620319,15.3839701146297));
#57448=CARTESIAN_POINT('Ctrl Pts',(1.46498307457946,0.793710571305735,15.3823881112902));
#57449=CARTESIAN_POINT('Ctrl Pts',(1.49116642231064,0.743645306132968,15.3787608699421));
#57450=CARTESIAN_POINT('Ctrl Pts',(1.50521310275329,0.71478622326705,15.3767272932658));
#57451=CARTESIAN_POINT('Ctrl Pts',(1.55392885379468,0.606884288466213,15.3693005980556));
#57452=CARTESIAN_POINT('Ctrl Pts',(1.58327531897998,0.525588997670174,15.3640542976308));
#57453=CARTESIAN_POINT('Ctrl Pts',(1.63002277261097,0.355859360144928,15.3532976158503));
#57454=CARTESIAN_POINT('Ctrl Pts',(1.6468199975481,0.267562899889985,15.3478005009654));
#57455=CARTESIAN_POINT('Ctrl Pts',(1.65810979065067,0.162712899987816,15.3409579379313));
#57456=CARTESIAN_POINT('Ctrl Pts',(1.65957247012197,0.147046720814122,15.3399272521456));
#57457=CARTESIAN_POINT('Ctrl Pts',(1.66137280831201,0.124285153722511,15.3384146607224));
#57458=CARTESIAN_POINT('Ctrl Pts',(1.66188736283359,0.117204079752066,15.3379419806333));
#57459=CARTESIAN_POINT('Ctrl Pts',(1.66271894086449,0.104650701030899,15.3370999173494));
#57460=CARTESIAN_POINT('Ctrl Pts',(1.66305424164536,0.0991798044272329,
15.3367315482994));
#57461=CARTESIAN_POINT('Ctrl Pts',(1.66372382786011,0.0872942244005637,
15.3359281517071));
#57462=CARTESIAN_POINT('Ctrl Pts',(1.66404801236243,0.0808793303274497,
15.3354926071388));
#57463=CARTESIAN_POINT('Ctrl Pts',(1.66486688344881,0.0625765696376846,
15.3342447127187));
#57464=CARTESIAN_POINT('Ctrl Pts',(1.66527131189861,0.0506853449523531,
15.3334276920026));
#57465=CARTESIAN_POINT('Ctrl Pts',(1.66590312541228,0.0235576766965499,
15.3315510303681));
#57466=CARTESIAN_POINT('Ctrl Pts',(1.66604889464,0.00832054946410637,15.3304877580062));
#57467=CARTESIAN_POINT('Ctrl Pts',(1.66538239538062,-0.152235772448115,
15.3192012849236));
#57468=CARTESIAN_POINT('Ctrl Pts',(1.64576940446321,-0.296851605038883,
15.3083906614042));
#57469=CARTESIAN_POINT('Ctrl Pts',(1.59046774197011,-0.500252120552606,
15.2933371410284));
#57470=CARTESIAN_POINT('Ctrl Pts',(1.56958736964694,-0.562349756946722,
15.2887515387907));
#57471=CARTESIAN_POINT('Ctrl Pts',(1.53850861289902,-0.639420241636941,
15.2830802278255));
#57472=CARTESIAN_POINT('Ctrl Pts',(1.53165379754557,-0.65567040756555,15.2818853707825));
#57473=CARTESIAN_POINT('Ctrl Pts',(1.52021390206232,-0.681631053313367,
15.2799773330015));
#57474=CARTESIAN_POINT('Ctrl Pts',(1.51579088730033,-0.691411018257144,
15.2792587176339));
#57475=CARTESIAN_POINT('Ctrl Pts',(1.50715536638607,-0.710024262663021,
15.2778911441648));
#57476=CARTESIAN_POINT('Ctrl Pts',(1.50295895894282,-0.71886447032848,15.2772416681038));
#57477=CARTESIAN_POINT('Ctrl Pts',(1.49311071067528,-0.739147667269043,
15.2757513016974));
#57478=CARTESIAN_POINT('Ctrl Pts',(1.4874047377871,-0.75056380770618,15.2749123275373));
#57479=CARTESIAN_POINT('Ctrl Pts',(1.46883234885912,-0.786678480135729,
15.2722567509974));
#57480=CARTESIAN_POINT('Ctrl Pts',(1.45547720843322,-0.811121285830036,
15.2704572535854));
#57481=CARTESIAN_POINT('Ctrl Pts',(1.40491734491293,-0.898383188327327,
15.2640089691905));
#57482=CARTESIAN_POINT('Ctrl Pts',(1.3642058792517,-0.959077159396175,15.25948187035));
#57483=CARTESIAN_POINT('Ctrl Pts',(1.23965898809748,-1.12070126200046,15.2469654666995));
#57484=CARTESIAN_POINT('Ctrl Pts',(1.14772461936356,-1.21467841656095,15.2391475890823));
#57485=CARTESIAN_POINT('Ctrl Pts',(1.0340588926637,-1.30633220382947,15.229660795745));
#57486=CARTESIAN_POINT('Ctrl Pts',(1.02223952680406,-1.31560173742588,15.2286758756794));
#57487=CARTESIAN_POINT('Ctrl Pts',(1.00469556309671,-1.32898173447869,15.227213469946));
#57488=CARTESIAN_POINT('Ctrl Pts',(0.999067253605341,-1.33321800294267,
15.2267442463408));
#57489=CARTESIAN_POINT('Ctrl Pts',(0.989023581819373,-1.34067827729617,
15.2259064652248));
#57490=CARTESIAN_POINT('Ctrl Pts',(0.984618977322235,-1.34391642467398,
15.2255388911628));
#57491=CARTESIAN_POINT('Ctrl Pts',(0.974901499512459,-1.35098703843999,
15.2247275055846));
#57492=CARTESIAN_POINT('Ctrl Pts',(0.969582002964589,-1.35480981972763,
15.2242830858361));
#57493=CARTESIAN_POINT('Ctrl Pts',(0.954038403877937,-1.36584158166964,
15.2229840784848));
#57494=CARTESIAN_POINT('Ctrl Pts',(0.943755737530097,-1.37296671001649,
15.2221242262529));
#57495=CARTESIAN_POINT('Ctrl Pts',(0.8596195262646,-1.42987516570604,15.2150907605256));
#57496=CARTESIAN_POINT('Ctrl Pts',(0.781969825852857,-1.47377356927853,
15.2086205781583));
#57497=CARTESIAN_POINT('Ctrl Pts',(0.58626384852657,-1.56457767545267,15.1929165860141));
#57498=CARTESIAN_POINT('Ctrl Pts',(0.465603492474386,-1.60462878300476,
15.1837488367089));
#57499=CARTESIAN_POINT('Ctrl Pts',(0.321410008702082,-1.63483181811235,
15.1736205306028));
#57500=CARTESIAN_POINT('Ctrl Pts',(0.301191611579758,-1.63867725496382,
15.1722173732211));
#57501=CARTESIAN_POINT('Ctrl Pts',(0.268506812889848,-1.64426832933593,
15.1699755121219));
#57502=CARTESIAN_POINT('Ctrl Pts',(0.256083365696785,-1.64624893995544,
15.1691294924123));
#57503=CARTESIAN_POINT('Ctrl Pts',(0.233980938909702,-1.64951636079465,
15.1676348309199));
#57504=CARTESIAN_POINT('Ctrl Pts',(0.224310968791953,-1.65085914013045,
15.1669844531109));
#57505=CARTESIAN_POINT('Ctrl Pts',(0.203893602002611,-1.65351159821838,
15.1656184620696));
#57506=CARTESIAN_POINT('Ctrl Pts',(0.193144081939528,-1.65480167371155,
15.1649034938252));
#57507=CARTESIAN_POINT('Ctrl Pts',(0.164422349999496,-1.65796494886197,
15.1630038921315));
#57508=CARTESIAN_POINT('Ctrl Pts',(0.146430633537744,-1.65965074395051,
15.1618251495231));
#57509=CARTESIAN_POINT('Ctrl Pts',(0.0472475442518117,-1.66731853994715,
15.1553827849607));
#57510=CARTESIAN_POINT('Ctrl Pts',(-0.0342755666667078,-1.66763638566252,
15.1502999042185));
#57511=CARTESIAN_POINT('Ctrl Pts',(-0.16602539576011,-1.6584801190757,15.1421777622315));
#57512=CARTESIAN_POINT('Ctrl Pts',(-0.21636093555196,-1.65266716942266,
15.1390947927211));
#57513=CARTESIAN_POINT('Ctrl Pts',(-0.351979994730006,-1.63070238828391,
15.1306972645686));
#57514=CARTESIAN_POINT('Ctrl Pts',(-0.436382153565351,-1.61016987802433,
15.1253742762429));
#57515=CARTESIAN_POINT('Ctrl Pts',(-0.533860854200183,-1.57822688011173,
15.1187199027992));
#57516=CARTESIAN_POINT('Ctrl Pts',(-0.548859047682911,-1.5730738055022,
15.1176812424208));
#57517=CARTESIAN_POINT('Ctrl Pts',(-0.570482611465693,-1.56529751618548,
15.1161590648939));
#57518=CARTESIAN_POINT('Ctrl Pts',(-0.577168828538687,-1.56284447815699,
15.1156849373639));
#57519=CARTESIAN_POINT('Ctrl Pts',(-0.588974858963148,-1.55842699089454,
15.1148412806736));
#57520=CARTESIAN_POINT('Ctrl Pts',(-0.59410100479565,-1.55648002406102,
15.1144727800796));
#57521=CARTESIAN_POINT('Ctrl Pts',(-0.605196632161427,-1.5522029820382,
15.1136703039472));
#57522=CARTESIAN_POINT('Ctrl Pts',(-0.611162218560856,-1.54986380052357,
15.1132358224526));
#57523=CARTESIAN_POINT('Ctrl Pts',(-0.62809858031899,-1.54310985417194,
15.1119939889164));
#57524=CARTESIAN_POINT('Ctrl Pts',(-0.639035786828177,-1.53861271666942,
15.111182034248));
#57525=CARTESIAN_POINT('Ctrl Pts',(-0.736029689118294,-1.49751841560116,
15.1038977632658));
#57526=CARTESIAN_POINT('Ctrl Pts',(-0.818901942218588,-1.45385590038076,
15.097093661109));
#57527=CARTESIAN_POINT('Ctrl Pts',(-1.00134058761238,-1.33716823178392,
15.0813290763024));
#57528=CARTESIAN_POINT('Ctrl Pts',(-1.09736863966334,-1.25956125883623,
15.072436700925));
#57529=CARTESIAN_POINT('Ctrl Pts',(-1.19858732368091,-1.15731391661627,
15.0625428972173));
#57530=CARTESIAN_POINT('Ctrl Pts',(-1.21291753097372,-1.14228639338515,
15.0611269147318));
#57531=CARTESIAN_POINT('Ctrl Pts',(-1.23541766086807,-1.11779040312,15.0588779019051));
#57532=CARTESIAN_POINT('Ctrl Pts',(-1.2437680257883,-1.10849145007598,15.0580372868624));
#57533=CARTESIAN_POINT('Ctrl Pts',(-1.25846419328916,-1.09175065420514,
15.0565467750719));
#57534=CARTESIAN_POINT('Ctrl Pts',(-1.26485051368203,-1.08434533327415,
15.0558952089094));
#57535=CARTESIAN_POINT('Ctrl Pts',(-1.27812608494293,-1.06867463420606,
15.0545323457399));
#57536=CARTESIAN_POINT('Ctrl Pts',(-1.28500122979276,-1.06039785524023,
15.0538216442932));
#57537=CARTESIAN_POINT('Ctrl Pts',(-1.3004985727496,-1.04136899700575,15.0522079146647));
#57538=CARTESIAN_POINT('Ctrl Pts',(-1.30906857449013,-1.03057528183028,
15.0513069913391));
#57539=CARTESIAN_POINT('Ctrl Pts',(-1.34775275171899,-0.980592205532774,
15.0471984674815));
#57540=CARTESIAN_POINT('Ctrl Pts',(-1.37624941168536,-0.94017914460346,
15.0440537276212));
#57541=CARTESIAN_POINT('Ctrl Pts',(-1.45222990873424,-0.821551267728504,
15.0352272624263));
#57542=CARTESIAN_POINT('Ctrl Pts',(-1.4951275765765,-0.740616453615575,
15.0296841960466));
#57543=CARTESIAN_POINT('Ctrl Pts',(-1.53305135900488,-0.652175104969901,
15.0237979377102));
#57544=CARTESIAN_POINT('Ctrl Pts',(-1.53491576265105,-0.647774990462892,
15.0235054848448));
#57545=CARTESIAN_POINT('Ctrl Pts',(-1.56681858847348,-0.571571158424203,
15.0184466161955));
#57546=CARTESIAN_POINT('Ctrl Pts',(-1.59180421959823,-0.497765513129217,
15.0136420231226));
#57547=CARTESIAN_POINT('Ctrl Pts',(-1.61554026550909,-0.407228099627312,
15.0075694629696));
#57548=CARTESIAN_POINT('Ctrl Pts',(-1.61932526842642,-0.391906500674153,
15.0065357084898));
#57549=CARTESIAN_POINT('Ctrl Pts',(-1.62449845592095,-0.369609653937734,
15.0050194272483));
#57550=CARTESIAN_POINT('Ctrl Pts',(-1.62606066465718,-0.362675116095122,
15.0045461889907));
#57551=CARTESIAN_POINT('Ctrl Pts',(-1.62874900461103,-0.35037513473146,
15.0037035117437));
#57552=CARTESIAN_POINT('Ctrl Pts',(-1.62989310038275,-0.345013818742599,
15.003335092459));
#57553=CARTESIAN_POINT('Ctrl Pts',(-1.63231902194102,-0.333364352626106,
15.0025320533508));
#57554=CARTESIAN_POINT('Ctrl Pts',(-1.63359096533703,-0.327074510607255,
15.0020969207898));
#57555=CARTESIAN_POINT('Ctrl Pts',(-1.63615204349318,-0.31402210817978,
15.0011909610798));
#57556=CARTESIAN_POINT('Ctrl Pts',(-1.63743566122322,-0.307258596595455,
15.000719850296));
#57557=CARTESIAN_POINT('Ctrl Pts',(-1.64064908818197,-0.289734505427428,
14.999495259328));
#57558=CARTESIAN_POINT('Ctrl Pts',(-1.64251493148324,-0.278962720389059,
14.9987386739575));
#57559=CARTESIAN_POINT('Ctrl Pts',(-1.65865690094451,-0.179990185347439,
14.9917564806084));
#57560=CARTESIAN_POINT('Ctrl Pts',(-1.66592020868823,-0.0908032192984881,
14.9852504582999));
#57561=CARTESIAN_POINT('Ctrl Pts',(-1.66599934620511,-0.00147595533024592,
14.9787480137938));
#57562=CARTESIAN_POINT('Ctrl Pts',(-1.66599934563946,-0.00147659367806648,
14.9787480602614));
#57563=CARTESIAN_POINT('Ctrl Pts',(-1.66610314052083,0.115632267753273,
14.970223295913));
#57564=CARTESIAN_POINT('Ctrl Pts',(-1.65385865480111,0.232450507843818,
14.9617624831313));
#57565=CARTESIAN_POINT('Ctrl Pts',(-1.62572354081887,0.364554152468414,
14.9524446927836));
#57566=CARTESIAN_POINT('Ctrl Pts',(-1.62171048484689,0.38201035004935,14.95121779562));
#57567=CARTESIAN_POINT('Ctrl Pts',(-1.61462003461837,0.410724018759949,
14.9492064580283));
#57568=CARTESIAN_POINT('Ctrl Pts',(-1.6117045585485,0.422019553761331,14.9484169717574));
#57569=CARTESIAN_POINT('Ctrl Pts',(-1.60577249778044,0.444043760741052,
14.9468807894801));
#57570=CARTESIAN_POINT('Ctrl Pts',(-1.60276643538076,0.454774603673521,
14.9461337994409));
#57571=CARTESIAN_POINT('Ctrl Pts',(-1.59693920745817,0.474800486290135,
14.9447422749769));
#57572=CARTESIAN_POINT('Ctrl Pts',(-1.59414399926716,0.484102520681658,
14.9440969310153));
#57573=CARTESIAN_POINT('Ctrl Pts',(-1.58769339545456,0.504907258900075,
14.9426555927583));
#57574=CARTESIAN_POINT('Ctrl Pts',(-1.58399400653956,0.516395834712217,
14.9418610710722));
#57575=CARTESIAN_POINT('Ctrl Pts',(-1.57483194207221,0.543823700837499,
14.9399669358166));
#57576=CARTESIAN_POINT('Ctrl Pts',(-1.56925173545991,0.559722128444655,
14.9388712276951));
#57577=CARTESIAN_POINT('Ctrl Pts',(-1.56343130047997,0.575533290678746,
14.9377828634576));
#57578=CARTESIAN_POINT('Ctrl Pts',(-1.56343130033034,0.575533291085225,
15.1319018884674));
#57579=CARTESIAN_POINT('Ctrl Pts',(-1.56361616135984,0.57503111766761,15.131940832256));
#57580=CARTESIAN_POINT('Ctrl Pts',(-1.56380078084195,0.574528854099077,
15.1319797768693));
#57581=CARTESIAN_POINT('Ctrl Pts',(-1.58799554347857,0.508608117607534,
15.1370903380066));
#57582=CARTESIAN_POINT('Ctrl Pts',(-1.60787910392355,0.441744119318942,
15.1421646437731));
#57583=CARTESIAN_POINT('Ctrl Pts',(-1.63386700579967,0.328880053710135,
15.1504511840247));
#57584=CARTESIAN_POINT('Ctrl Pts',(-1.64234636377242,0.283518137176467,
15.153710363797));
#57585=CARTESIAN_POINT('Ctrl Pts',(-1.65349195996309,0.206252539600368,
15.1591338921667));
#57586=CARTESIAN_POINT('Ctrl Pts',(-1.65714180010835,0.174519535944458,
15.161325577219));
#57587=CARTESIAN_POINT('Ctrl Pts',(-1.66102950745032,0.129297731720683,
15.1644001437324));
#57588=CARTESIAN_POINT('Ctrl Pts',(-1.66201931706476,0.115882423954891,
15.1653061940844));
#57589=CARTESIAN_POINT('Ctrl Pts',(-1.66345473009269,0.0925859279795217,
15.1668695338818));
#57590=CARTESIAN_POINT('Ctrl Pts',(-1.66397500639951,0.0827102077369872,
15.1675291232221));
#57591=CARTESIAN_POINT('Ctrl Pts',(-1.66480936250623,0.063642466787182,
15.1687968193843));
#57592=CARTESIAN_POINT('Ctrl Pts',(-1.6651353196239,0.0544513558431828,
15.1694052734281));
#57593=CARTESIAN_POINT('Ctrl Pts',(-1.66579791750518,0.0300692769474208,
15.1710127574103));
#57594=CARTESIAN_POINT('Ctrl Pts',(-1.66600288474831,0.0148753640508772,
15.1720076618229));
#57595=CARTESIAN_POINT('Ctrl Pts',(-1.66599141262338,-0.0449168762953361,
15.1758984239819));
#57596=CARTESIAN_POINT('Ctrl Pts',(-1.66419214261104,-0.0894984125453231,
15.1787452250402));
#57597=CARTESIAN_POINT('Ctrl Pts',(-1.65447971146818,-0.209898876319166,
15.1863433868392));
#57598=CARTESIAN_POINT('Ctrl Pts',(-1.64315124127635,-0.285334476225436,
15.1910031942807));
#57599=CARTESIAN_POINT('Ctrl Pts',(-1.60398435113785,-0.462445840440378,
15.2020801555452));
#57600=CARTESIAN_POINT('Ctrl Pts',(-1.57159591876881,-0.562762903924878,
15.2084629755019));
#57601=CARTESIAN_POINT('Ctrl Pts',(-1.52404955292086,-0.673092222856647,
15.2162692432924));
#57602=CARTESIAN_POINT('Ctrl Pts',(-1.51793908235321,-0.686761300788102,
15.2172510817204));
#57603=CARTESIAN_POINT('Ctrl Pts',(-1.50868784009518,-0.706729440802907,
15.2187097746519));
#57604=CARTESIAN_POINT('Ctrl Pts',(-1.50568985276522,-0.713094358522818,
15.2191784270216));
#57605=CARTESIAN_POINT('Ctrl Pts',(-1.50029097012475,-0.724370685617352,
15.2200156191681));
#57606=CARTESIAN_POINT('Ctrl Pts',(-1.49790609030435,-0.729289536626178,
15.220383181474));
#57607=CARTESIAN_POINT('Ctrl Pts',(-1.49260683036372,-0.74008368449563,
15.2211950715736));
#57608=CARTESIAN_POINT('Ctrl Pts',(-1.48968199070575,-0.745953465692557,
15.2216400127325));
#57609=CARTESIAN_POINT('Ctrl Pts',(-1.48106128491802,-0.763001219460017,
15.2229419892763));
#57610=CARTESIAN_POINT('Ctrl Pts',(-1.47527386582907,-0.774132022226061,
15.2238043245399));
#57611=CARTESIAN_POINT('Ctrl Pts',(-1.42995469326256,-0.858939191178976,
15.230463056535));
#57612=CARTESIAN_POINT('Ctrl Pts',(-1.38505648227977,-0.929603388047205,
15.2365212459306));
#57613=CARTESIAN_POINT('Ctrl Pts',(-1.25531384855932,-1.10340888526968,
15.2523031532071));
#57614=CARTESIAN_POINT('Ctrl Pts',(-1.16302820362113,-1.20029279239507,
15.2619704010721));
#57615=CARTESIAN_POINT('Ctrl Pts',(-1.044793441589,-1.29782885296469,15.2724979066783));
#57616=CARTESIAN_POINT('Ctrl Pts',(-1.02919534293735,-1.31023283155317,
15.273855660094));
#57617=CARTESIAN_POINT('Ctrl Pts',(-1.0035428472475,-1.32989145701371,15.2760397065342));
#57618=CARTESIAN_POINT('Ctrl Pts',(-0.993623837151769,-1.33731866746045,
15.2768727194598));
#57619=CARTESIAN_POINT('Ctrl Pts',(-0.975760075226436,-1.35038630644674,
15.2783529303569));
#57620=CARTESIAN_POINT('Ctrl Pts',(-0.967847063925048,-1.35606893955259,
15.2790017438661));
#57621=CARTESIAN_POINT('Ctrl Pts',(-0.950947963222408,-1.36798154894886,
15.2803731168512));
#57622=CARTESIAN_POINT('Ctrl Pts',(-0.941949436799228,-1.3741931505919,
15.2810949541027));
#57623=CARTESIAN_POINT('Ctrl Pts',(-0.917505101561957,-1.39071392125247,
15.2830338245257));
#57624=CARTESIAN_POINT('Ctrl Pts',(-0.901946728412277,-1.40085437008657,
15.2842445208855));
#57625=CARTESIAN_POINT('Ctrl Pts',(-0.80636672785814,-1.46089766725242,
15.2915488419405));
#57626=CARTESIAN_POINT('Ctrl Pts',(-0.722392148678671,-1.50419488081408,
15.2973933048079));
#57627=CARTESIAN_POINT('Ctrl Pts',(-0.54980268009964,-1.57537459087858,
15.3088263182101));
#57628=CARTESIAN_POINT('Ctrl Pts',(-0.461635419337567,-1.60342716694281,
15.3144007079377));
#57629=CARTESIAN_POINT('Ctrl Pts',(-0.332536864355155,-1.63296706330143,
15.3227190177802));
#57630=CARTESIAN_POINT('Ctrl Pts',(-0.293162758188266,-1.64049297987491,
15.3252774797753));
#57631=CARTESIAN_POINT('Ctrl Pts',(-0.243251161177065,-1.64817888946851,
15.3285907958126));
#57632=CARTESIAN_POINT('Ctrl Pts',(-0.232928588017561,-1.64966937241577,
15.3292798018988));
#57633=CARTESIAN_POINT('Ctrl Pts',(-0.21654010206061,-1.65187883576524,
15.3303806159117));
#57634=CARTESIAN_POINT('Ctrl Pts',(-0.210482855429853,-1.65266157104735,
15.3307889766175));
#57635=CARTESIAN_POINT('Ctrl Pts',(-0.198902204518846,-1.65409335952586,
15.331572799926));
#57636=CARTESIAN_POINT('Ctrl Pts',(-0.193379675546292,-1.65474808543996,
15.3319479480327));
#57637=CARTESIAN_POINT('Ctrl Pts',(-0.180090778258695,-1.65625612659678,
15.3328538176313));
#57638=CARTESIAN_POINT('Ctrl Pts',(-0.172321547705302,-1.65708247332934,
15.3333859977557));
#57639=CARTESIAN_POINT('Ctrl Pts',(-0.145123392740526,-1.65978197168793,
15.3352573525776));
#57640=CARTESIAN_POINT('Ctrl Pts',(-0.125668443500807,-1.66136821710382,
15.3366107707493));
#57641=CARTESIAN_POINT('Ctrl Pts',(-0.076840719859529,-1.66448684848598,
15.3400374689082));
#57642=CARTESIAN_POINT('Ctrl Pts',(-0.0474473920416858,-1.66558383425887,
15.3421272809172));
#57643=CARTESIAN_POINT('Ctrl Pts',(0.0963539027338841,-1.6671412476357,
15.3524388117315));
#57644=CARTESIAN_POINT('Ctrl Pts',(0.210574837179333,-1.65659424850831,
15.3608733439559));
#57645=CARTESIAN_POINT('Ctrl Pts',(0.391573247987135,-1.62084482159528,
15.3740845559402));
#57646=CARTESIAN_POINT('Ctrl Pts',(0.459409253531182,-1.60293887422585,
15.3790058446962));
#57647=CARTESIAN_POINT('Ctrl Pts',(0.542921182261424,-1.57515506310888,
15.3850149435742));
#57648=CARTESIAN_POINT('Ctrl Pts',(0.559826647023912,-1.56922625894704,
15.3862290386469));
#57649=CARTESIAN_POINT('Ctrl Pts',(0.586759934676838,-1.55928999024948,
15.3881602369433));
#57650=CARTESIAN_POINT('Ctrl Pts',(0.596849736355327,-1.55545584840314,
15.3888830132001));
#57651=CARTESIAN_POINT('Ctrl Pts',(0.616001174482712,-1.54796447673093,
15.3902538509961));
#57652=CARTESIAN_POINT('Ctrl Pts',(0.625069247711218,-1.54432506639398,
15.3909024747662));
#57653=CARTESIAN_POINT('Ctrl Pts',(0.64579758603769,-1.5357933966104,15.3923843670322));
#57654=CARTESIAN_POINT('Ctrl Pts',(0.657435317248927,-1.5308477055225,15.393215795302));
#57655=CARTESIAN_POINT('Ctrl Pts',(0.69391401204112,-1.51485261569091,15.3958211418802));
#57656=CARTESIAN_POINT('Ctrl Pts',(0.718542229232651,-1.50332707785994,
15.3975788833002));
#57657=CARTESIAN_POINT('Ctrl Pts',(0.813063371919907,-1.45623911801496,
15.4043359912983));
#57658=CARTESIAN_POINT('Ctrl Pts',(0.880696079452157,-1.41636178492724,
15.4091891916242));
#57659=CARTESIAN_POINT('Ctrl Pts',(1.01902951311069,-1.32104408387472,15.4194814262418));
#57660=CARTESIAN_POINT('Ctrl Pts',(1.08856215675058,-1.26436122821991,15.4248882478937));
#57661=CARTESIAN_POINT('Ctrl Pts',(1.18499499386729,-1.171871986873,15.4332504183841));
#57662=CARTESIAN_POINT('Ctrl Pts',(1.21556672089116,-1.14012889386062,15.436053697404));
#57663=CARTESIAN_POINT('Ctrl Pts',(1.25195208085808,-1.09922083844663,15.4396433894396));
#57664=CARTESIAN_POINT('Ctrl Pts',(1.25898505224871,-1.09115859888617,15.4403498111022));
#57665=CARTESIAN_POINT('Ctrl Pts',(1.26994827796263,-1.07834382058579,15.4414720759996));
#57666=CARTESIAN_POINT('Ctrl Pts',(1.2739307697762,-1.07363607187405,15.4418842400137));
#57667=CARTESIAN_POINT('Ctrl Pts',(1.28144163280502,-1.06465676956197,15.442670392491));
#57668=CARTESIAN_POINT('Ctrl Pts',(1.28497494707483,-1.06038958731908,15.4430440190084));
#57669=CARTESIAN_POINT('Ctrl Pts',(1.29335619278066,-1.05016415963807,15.4439392943375));
#57670=CARTESIAN_POINT('Ctrl Pts',(1.29818428276112,-1.0441899088713,15.4444623142954));
#57671=CARTESIAN_POINT('Ctrl Pts',(1.3146160015383,-1.02356728570179,15.4462669497862));
#57672=CARTESIAN_POINT('Ctrl Pts',(1.32601390710347,-1.00875778326753,15.4475615359026));
#57673=CARTESIAN_POINT('Ctrl Pts',(1.35368100202988,-0.971530177355729,
15.4508062309763));
#57674=CARTESIAN_POINT('Ctrl Pts',(1.36964445898344,-0.948892524567445,
15.452770866562));
#57675=CARTESIAN_POINT('Ctrl Pts',(1.4331485099955,-0.853894889023707,15.4609497533487));
#57676=CARTESIAN_POINT('Ctrl Pts',(1.47557720258271,-0.778281844100804,
15.4672988997019));
#57677=CARTESIAN_POINT('Ctrl Pts',(1.55351359134398,-0.609877807786816,
15.4807476175074));
#57678=CARTESIAN_POINT('Ctrl Pts',(1.58700629749733,-0.516500350930187,
15.4877922953916));
#57679=CARTESIAN_POINT('Ctrl Pts',(1.61677329856461,-0.402437323488599,
15.4958523597803));
#57680=CARTESIAN_POINT('Ctrl Pts',(1.6212256194518,-0.384108369944496,15.4971319966596));
#57681=CARTESIAN_POINT('Ctrl Pts',(1.62777959314886,-0.35497957903697,15.4991418974932));
#57682=CARTESIAN_POINT('Ctrl Pts',(1.63008706800584,-0.344228218134433,
15.4998786779808));
#57683=CARTESIAN_POINT('Ctrl Pts',(1.63404094310774,-0.324873669350474,
15.5011961979069));
#57684=CARTESIAN_POINT('Ctrl Pts',(1.63572624309877,-0.316278939288609,
15.5017781554477));
#57685=CARTESIAN_POINT('Ctrl Pts',(1.63952565043933,-0.296059509554514,
15.5031401434138));
#57686=CARTESIAN_POINT('Ctrl Pts',(1.64158404701692,-0.284424718083948,
15.503918381723));
#57687=CARTESIAN_POINT('Ctrl Pts',(1.64725422119827,-0.250260114800376,
15.5061883109003));
#57688=CARTESIAN_POINT('Ctrl Pts',(1.65052724552913,-0.227676278102937,
15.5076693316686));
#57689=CARTESIAN_POINT('Ctrl Pts',(1.66350310555647,-0.123041340112761,
15.5144520701939));
#57690=CARTESIAN_POINT('Ctrl Pts',(1.66755857594905,-0.0404037355153956,
15.5195776968399));
#57691=CARTESIAN_POINT('Ctrl Pts',(1.66401260858061,0.0995352561302625,
15.528160021742));
#57692=CARTESIAN_POINT('Ctrl Pts',(1.6596002720334,0.156754874360539,15.5316438346879));
#57693=CARTESIAN_POINT('Ctrl Pts',(1.64236578164872,0.290047389158333,15.5398919773014));
#57694=CARTESIAN_POINT('Ctrl Pts',(1.62719742072614,0.365675095095598,15.5446744492416));
#57695=CARTESIAN_POINT('Ctrl Pts',(1.60378997397939,0.451163361594568,15.5504719451597));
#57696=CARTESIAN_POINT('Ctrl Pts',(1.60060866897334,0.462322971283944,15.5512366563818));
#57697=CARTESIAN_POINT('Ctrl Pts',(1.59548355475557,0.479613996381464,15.5524351662606));
#57698=CARTESIAN_POINT('Ctrl Pts',(1.59362030021713,0.485769177991499,15.5528645114519));
#57699=CARTESIAN_POINT('Ctrl Pts',(1.59010328075809,0.497149467173237,15.5536636122648));
#57700=CARTESIAN_POINT('Ctrl Pts',(1.58845931419022,0.502377388186974,15.5540328057851));
#57701=CARTESIAN_POINT('Ctrl Pts',(1.58459283676959,0.514464310178104,15.5548912005595));
#57702=CARTESIAN_POINT('Ctrl Pts',(1.5823515728622,0.521317062651944,15.5553814599198));
#57703=CARTESIAN_POINT('Ctrl Pts',(1.57501853837099,0.543255093207375,15.5569620011035));
#57704=CARTESIAN_POINT('Ctrl Pts',(1.56975514904773,0.558281486560275,15.558061419231));
#57705=CARTESIAN_POINT('Ctrl Pts',(1.55660255824174,0.594173400221159,15.5607243063574));
#57706=CARTESIAN_POINT('Ctrl Pts',(1.54850816914736,0.614960082912384,15.5622967607548));
#57707=CARTESIAN_POINT('Ctrl Pts',(1.51500737247164,0.696132328839791,15.5685411125132));
#57708=CARTESIAN_POINT('Ctrl Pts',(1.48646674771988,0.755157775666766,15.5733089133505));
#57709=CARTESIAN_POINT('Ctrl Pts',(1.39506810007054,0.918809440581174,15.5869538678157));
#57710=CARTESIAN_POINT('Ctrl Pts',(1.32408918593116,1.01844193569244,15.5957620859157));
#57711=CARTESIAN_POINT('Ctrl Pts',(1.22891548996442,1.12506041555669,15.6055925319363));
#57712=CARTESIAN_POINT('Ctrl Pts',(1.21468142841152,1.14041366031784,15.6070204635948));
#57713=CARTESIAN_POINT('Ctrl Pts',(1.1914595094393,1.16453322974893,15.6092846298786));
#57714=CARTESIAN_POINT('Ctrl Pts',(1.18265580447379,1.17347290932298,15.6101286119361));
#57715=CARTESIAN_POINT('Ctrl Pts',(1.16680733683392,1.18920662306649,15.6116229736571));
#57716=CARTESIAN_POINT('Ctrl Pts',(1.15980220485253,1.19603955046502,15.6122750531022));
#57717=CARTESIAN_POINT('Ctrl Pts',(1.14498659836475,1.21023837904477,15.6136368748456));
#57718=CARTESIAN_POINT('Ctrl Pts',(1.13716428832194,1.21759132512249,15.61434604002));
#57719=CARTESIAN_POINT('Ctrl Pts',(1.11629987648073,1.23682733723651,15.6162122795394));
#57720=CARTESIAN_POINT('Ctrl Pts',(1.10313892233263,1.24857992660578,15.6173638323033));
#57721=CARTESIAN_POINT('Ctrl Pts',(1.03432386149207,1.30809338485769,15.6232596993818));
#57722=CARTESIAN_POINT('Ctrl Pts',(0.975743681172082,1.352353644106,15.6278599126304));
#57723=CARTESIAN_POINT('Ctrl Pts',(0.83249976794347,1.44641180458262,15.6384368342263));
#57724=CARTESIAN_POINT('Ctrl Pts',(0.745984384011499,1.49287279354739,15.6443308149655));
#57725=CARTESIAN_POINT('Ctrl Pts',(0.631770903264547,1.54178790590093,15.6520381779966));
#57726=CARTESIAN_POINT('Ctrl Pts',(0.607412321536898,1.55154586800623,15.6536787455991));
#57727=CARTESIAN_POINT('Ctrl Pts',(0.552608276617389,1.5720118097666,15.6573836339149));
#57728=CARTESIAN_POINT('Ctrl Pts',(0.522062788756211,1.58241813713555,15.6594578675558));
#57729=CARTESIAN_POINT('Ctrl Pts',(0.481963888388505,1.59479183204463,15.6622162615394));
#57730=CARTESIAN_POINT('Ctrl Pts',(0.472666298186928,1.59757213817262,15.6628582854483));
#57731=CARTESIAN_POINT('Ctrl Pts',(0.457631191862638,1.60192542886301,15.6639012343168));
#57732=CARTESIAN_POINT('Ctrl Pts',(0.451908449527273,1.60354923150448,15.664299307197));
#57733=CARTESIAN_POINT('Ctrl Pts',(0.440744141300227,1.60665254530285,15.6650782568018));
#57734=CARTESIAN_POINT('Ctrl Pts',(0.435303573703352,1.60813512942125,15.6654589562031));
#57735=CARTESIAN_POINT('Ctrl Pts',(0.421890245721668,1.61171728124755,15.6664000921706));
#57736=CARTESIAN_POINT('Ctrl Pts',(0.413909289399275,1.61378532251391,15.666962275919));
#57737=CARTESIAN_POINT('Ctrl Pts',(0.384137323976427,1.62126452064838,15.6690667986451));
#57738=CARTESIAN_POINT('Ctrl Pts',(0.362254040495224,1.62629395199782,15.6706283123874));
#57739=CARTESIAN_POINT('Ctrl Pts',(0.197699965571217,1.66062757513977,15.6824467648954));
#57740=CARTESIAN_POINT('Ctrl Pts',(0.0518380313566741,1.67155189733355,
15.6932822599853));
#57741=CARTESIAN_POINT('Ctrl Pts',(-0.158463322462585,1.65971893832539,
15.708320737297));
#57742=CARTESIAN_POINT('Ctrl Pts',(-0.223071719129287,1.65227675781392,
15.7128718494041));
#57743=CARTESIAN_POINT('Ctrl Pts',(-0.304435615465388,1.63804307392182,
15.7185087287761));
#57744=CARTESIAN_POINT('Ctrl Pts',(-0.321734750386793,1.63473329559382,
15.7197019335164));
#57745=CARTESIAN_POINT('Ctrl Pts',(-0.349483187294076,1.62896673095832,
15.7216080406818));
#57746=CARTESIAN_POINT('Ctrl Pts',(-0.35996650451912,1.62668227804572,15.7223263565386));
#57747=CARTESIAN_POINT('Ctrl Pts',(-0.379970243891386,1.6221203466728,15.7236938051796));
#57748=CARTESIAN_POINT('Ctrl Pts',(-0.389494054462821,1.61985993031703,
15.724343451796));
#57749=CARTESIAN_POINT('Ctrl Pts',(-0.41140094225353,1.61445609090268,15.7258348440392));
#57750=CARTESIAN_POINT('Ctrl Pts',(-0.423768992529285,1.61125387845079,
15.726674665631));
#57751=CARTESIAN_POINT('Ctrl Pts',(-0.463042919572187,1.6006019545044,15.7293355606454));
#57752=CARTESIAN_POINT('Ctrl Pts',(-0.48979978363936,1.59261786990147,15.7311394320014));
#57753=CARTESIAN_POINT('Ctrl Pts',(-0.588095900884025,1.56057506312904,
15.7377493515085));
#57754=CARTESIAN_POINT('Ctrl Pts',(-0.658178849962615,1.53233599965577,
15.7424236854143));
#57755=CARTESIAN_POINT('Ctrl Pts',(-0.80342682049788,1.4619989098313,15.7523158338598));
#57756=CARTESIAN_POINT('Ctrl Pts',(-0.87772689360696,1.41863655468647,15.7575040189252));
#57757=CARTESIAN_POINT('Ctrl Pts',(-0.988666687139947,1.34182672204963,
15.7659139182053));
#57758=CARTESIAN_POINT('Ctrl Pts',(-1.02772865427485,1.31214846722543,15.7690215649535));
#57759=CARTESIAN_POINT('Ctrl Pts',(-1.07377636659147,1.27384396065812,15.772946060816));
#57760=CARTESIAN_POINT('Ctrl Pts',(-1.08206331582573,1.26681217500199,15.7736632262553));
#57761=CARTESIAN_POINT('Ctrl Pts',(-1.095018414601,1.25559943197579,15.7748027970607));
#57762=CARTESIAN_POINT('Ctrl Pts',(-1.09973295692987,1.251472205888,15.7752214190555));
#57763=CARTESIAN_POINT('Ctrl Pts',(-1.10855045474257,1.24366485295932,15.7760120057806));
#57764=CARTESIAN_POINT('Ctrl Pts',(-1.11265856675455,1.23999084167605,15.7763835308096));
#57765=CARTESIAN_POINT('Ctrl Pts',(-1.11679516490339,1.23625424716575,15.7767608329646));
#57766=CARTESIAN_POINT('Ctrl Pts',(-1.11684201880059,1.23621191914185,15.776765106959));
#57767=CARTESIAN_POINT('Ctrl Pts',(-1.11693545101566,1.23612750240639,15.7767736306393));
#57768=CARTESIAN_POINT('Ctrl Pts',(-1.11698202936455,1.23608541372255,15.7767778803231));
#57769=CARTESIAN_POINT('Ctrl Pts',(-1.11707492429919,1.23600146334848,15.7767863566281));
#57770=CARTESIAN_POINT('Ctrl Pts',(-1.11712124090509,1.23595960169267,15.7767905832467));
#57771=CARTESIAN_POINT('Ctrl Pts',(-1.11721362582353,1.23587609335685,15.7767990146368));
#57772=CARTESIAN_POINT('Ctrl Pts',(-1.11725969415998,1.23583444670485,15.7768032194062));
#57773=CARTESIAN_POINT('Ctrl Pts',(-1.11735159571182,1.23575135661608,15.7768116082875));
#57774=CARTESIAN_POINT('Ctrl Pts',(-1.11739742894896,1.23570991320637,15.7768157923974));
#57775=CARTESIAN_POINT('Ctrl Pts',(-1.12265460424378,1.2309557293336,15.7772957648682));
#57776=CARTESIAN_POINT('Ctrl Pts',(-1.12783596631153,1.22621017637931,15.7777739638914));
#57777=CARTESIAN_POINT('Ctrl Pts',(-1.14488711497387,1.21039371762603,15.7793643304808));
#57778=CARTESIAN_POINT('Ctrl Pts',(-1.15662469990001,1.19918251846607,15.7804861450412));
#57779=CARTESIAN_POINT('Ctrl Pts',(-1.18490100450508,1.17137294811743,15.7832515650871));
#57780=CARTESIAN_POINT('Ctrl Pts',(-1.20125666179133,1.15459399472173,15.7849055649239));
#57781=CARTESIAN_POINT('Ctrl Pts',(-1.2660765272628,1.08522806737833,15.7916666894247));
#57782=CARTESIAN_POINT('Ctrl Pts',(-1.31148390390257,1.02989260290088,15.7968839343634));
#57783=CARTESIAN_POINT('Ctrl Pts',(-1.41925806813393,0.87982346978274,15.8103289024379));
#57784=CARTESIAN_POINT('Ctrl Pts',(-1.47578078979527,0.781320870746174,
15.8184820032896));
#57785=CARTESIAN_POINT('Ctrl Pts',(-1.53138047687393,0.656487360804334,
15.827886659614));
#57786=CARTESIAN_POINT('Ctrl Pts',(-1.54043628712573,0.634947211320445,
15.8294795787709));
#57787=CARTESIAN_POINT('Ctrl Pts',(-1.55348075342465,0.601996127229037,
15.8318726135231));
#57788=CARTESIAN_POINT('Ctrl Pts',(-1.5578029886287,0.590721296717067,15.8326838112989));
#57789=CARTESIAN_POINT('Ctrl Pts',(-1.56248027293879,0.578111827419007,
15.8335827743951));
#57790=CARTESIAN_POINT('Ctrl Pts',(-1.56295658424666,0.576822853297328,
15.8336745732498));
#57791=CARTESIAN_POINT('Ctrl Pts',(-1.5634313003304,0.575533291085054,15.8337663187435));
#57792=CARTESIAN_POINT('Origin',(0.,0.,11.));
#57793=CARTESIAN_POINT('',(-1.56343130033213,0.57553329108036,16.5321096688871));
#57794=CARTESIAN_POINT('',(-1.5634313003322,0.575533291080154,16.3407718992107));
#57795=CARTESIAN_POINT('',(-1.56343130033213,0.575533291080363,11.));
#57796=CARTESIAN_POINT('',(-1.66599956897413,0.00119840644346202,16.5714803634422));
#57797=CARTESIAN_POINT('Ctrl Pts',(-1.56343130033213,0.575533291080358,
16.5321096688871));
#57798=CARTESIAN_POINT('Ctrl Pts',(-1.58445950918258,0.518410340216824,
16.5361801898729));
#57799=CARTESIAN_POINT('Ctrl Pts',(-1.60232716192958,0.460203709933027,
16.5402507108586));
#57800=CARTESIAN_POINT('Ctrl Pts',(-1.61694683874032,0.40129654955867,16.5443212318443));
#57801=CARTESIAN_POINT('Ctrl Pts',(-1.63029117873162,0.347528112257761,
16.5480366639075));
#57802=CARTESIAN_POINT('Ctrl Pts',(-1.64093007365734,0.293176473642386,
16.5517520959706));
#57803=CARTESIAN_POINT('Ctrl Pts',(-1.64883476380889,0.238537044618418,
16.5554675280337));
#57804=CARTESIAN_POINT('Ctrl Pts',(-1.66019068866406,0.160041716119839,
16.5608051398192));
#57805=CARTESIAN_POINT('Ctrl Pts',(-1.6659423645046,0.0807228119652788,
16.5661427516047));
#57806=CARTESIAN_POINT('Ctrl Pts',(-1.66599956897358,0.00119840721805856,
16.5714803633902));
#57807=CARTESIAN_POINT('',(1.26907087985246,1.07935865304843,17.));
#57808=CARTESIAN_POINT('Ctrl Pts',(-1.66599956897413,0.00119840644346203,
16.5714803634422));
#57809=CARTESIAN_POINT('Ctrl Pts',(-1.66604263708935,-0.058673986420678,
16.5754989485644));
#57810=CARTESIAN_POINT('Ctrl Pts',(-1.66285394991176,-0.118667824823123,
16.5795175336867));
#57811=CARTESIAN_POINT('Ctrl Pts',(-1.65642067872897,-0.178399930154282,
16.5835361188089));
#57812=CARTESIAN_POINT('Ctrl Pts',(-1.64999457545002,-0.238065482409234,
16.5875502264529));
#57813=CARTESIAN_POINT('Ctrl Pts',(-1.64033110092478,-0.297469358720189,
16.5915643340969));
#57814=CARTESIAN_POINT('Ctrl Pts',(-1.62746943601073,-0.356229188656582,
16.5955784417409));
#57815=CARTESIAN_POINT('Ctrl Pts',(-1.61461702011814,-0.414946763493643,
16.5995896627782));
#57816=CARTESIAN_POINT('Ctrl Pts',(-1.59857108150669,-0.473020696127689,
16.6036008838155));
#57817=CARTESIAN_POINT('Ctrl Pts',(-1.57942222074496,-0.530076832748849,
16.6076121048528));
#57818=CARTESIAN_POINT('Ctrl Pts',(-1.56027956710547,-0.587114474566646,
16.6116220256488));
#57819=CARTESIAN_POINT('Ctrl Pts',(-1.53803615354127,-0.64313447551882,
16.6156319464449));
#57820=CARTESIAN_POINT('Ctrl Pts',(-1.51283233092265,-0.697778144194223,
16.6196418672409));
#57821=CARTESIAN_POINT('Ctrl Pts',(-1.48760918706544,-0.752463702680382,
16.6236548620403));
#57822=CARTESIAN_POINT('Ctrl Pts',(-1.45942131712902,-0.805770339496956,
16.6276678568398));
#57823=CARTESIAN_POINT('Ctrl Pts',(-1.42845651654735,-0.857361055992991,
16.6316808516392));
#57824=CARTESIAN_POINT('Ctrl Pts',(-1.39748096695344,-0.908969681509355,
16.6356952394956));
#57825=CARTESIAN_POINT('Ctrl Pts',(-1.36372686056116,-0.958860761762857,
16.6397096273519));
#57826=CARTESIAN_POINT('Ctrl Pts',(-1.32742536695106,-1.00672632585765,
16.6437240152083));
#57827=CARTESIAN_POINT('Ctrl Pts',(-1.29105750900536,-1.05467939506706,
16.6477457419413));
#57828=CARTESIAN_POINT('Ctrl Pts',(-1.25213330206962,-1.10059914757466,
16.6517674686743));
#57829=CARTESIAN_POINT('Ctrl Pts',(-1.21092354286444,-1.14421159465224,
16.6557891954073));
#57830=CARTESIAN_POINT('Ctrl Pts',(-1.17399601511252,-1.18329213966994,
16.65939301228));
#57831=CARTESIAN_POINT('Ctrl Pts',(-1.13523397431683,-1.2205203066986,16.6629968291527));
#57832=CARTESIAN_POINT('Ctrl Pts',(-1.09485449139006,-1.25572673885803,
16.6666006460254));
#57833=CARTESIAN_POINT('Ctrl Pts',(-1.04910619660825,-1.29561417970431,
16.6706836224451));
#57834=CARTESIAN_POINT('Ctrl Pts',(-1.00108366919819,-1.33307823890073,
16.6747665988648));
#57835=CARTESIAN_POINT('Ctrl Pts',(-0.951073693211118,-1.36785044141593,
16.6788495752846));
#57836=CARTESIAN_POINT('Ctrl Pts',(-0.900608099450398,-1.40293943739448,
16.6829697498151));
#57837=CARTESIAN_POINT('Ctrl Pts',(-0.848119000144949,-1.43528687187874,
16.6870899243456));
#57838=CARTESIAN_POINT('Ctrl Pts',(-0.793937348164885,-1.46465678136173,
16.6912100988761));
#57839=CARTESIAN_POINT('Ctrl Pts',(-0.740389486995609,-1.49368313582077,
16.6952820775938));
#57840=CARTESIAN_POINT('Ctrl Pts',(-0.685188917555343,-1.51980100130237,
16.6993540563115));
#57841=CARTESIAN_POINT('Ctrl Pts',(-0.628684192549413,-1.5428260388127,
16.7034260350292));
#57842=CARTESIAN_POINT('Ctrl Pts',(-0.57221301555606,-1.56583740588666,
16.7074955961298));
#57843=CARTESIAN_POINT('Ctrl Pts',(-0.51443968997464,-1.58575939410111,
16.7115651572303));
#57844=CARTESIAN_POINT('Ctrl Pts',(-0.455734440004197,-1.60245502907073,
16.7156347183309));
#57845=CARTESIAN_POINT('Ctrl Pts',(-0.397042420022204,-1.61914690146275,
16.7197033623031));
#57846=CARTESIAN_POINT('Ctrl Pts',(-0.337419383184623,-1.63261372476495,
16.7237720062753));
#57847=CARTESIAN_POINT('Ctrl Pts',(-0.277250486948461,-1.64276844609544,
16.7278406502476));
#57848=CARTESIAN_POINT('Ctrl Pts',(-0.215763711383714,-1.65314558628628,
16.7319984097283));
#57849=CARTESIAN_POINT('Ctrl Pts',(-0.15370741766246,-1.66006366939857,
16.7361561692091));
#57850=CARTESIAN_POINT('Ctrl Pts',(-0.0915009175646956,-1.66348537176761,
16.7403139286899));
#57851=CARTESIAN_POINT('Ctrl Pts',(-0.030549016544634,-1.66683806423206,
16.7443878332487));
#57852=CARTESIAN_POINT('Ctrl Pts',(0.0305465650727917,-1.66683417686648,
16.7484617378075));
#57853=CARTESIAN_POINT('Ctrl Pts',(0.0913913808401572,-1.66349139327744,
16.7525356423664));
#57854=CARTESIAN_POINT('Ctrl Pts',(0.154114788951663,-1.66004540076947,
16.7567353293081));
#57855=CARTESIAN_POINT('Ctrl Pts',(0.216571105926717,-1.65305096757422,
16.7609350162499));
#57856=CARTESIAN_POINT('Ctrl Pts',(0.27833681905625,-1.64258473606619,16.7651347031916));
#57857=CARTESIAN_POINT('Ctrl Pts',(0.340102532185782,-1.63211850455817,
16.7693343901334));
#57858=CARTESIAN_POINT('Ctrl Pts',(0.401177085533186,-1.61818067345858,
16.7735340770751));
#57859=CARTESIAN_POINT('Ctrl Pts',(0.461154195597915,-1.60090374722606,
16.7777337640169));
#57860=CARTESIAN_POINT('Ctrl Pts',(0.518754461466997,-1.58431149155853,
16.7817670207735));
#57861=CARTESIAN_POINT('Ctrl Pts',(0.575591792928433,-1.56456790261253,
16.7858002775301));
#57862=CARTESIAN_POINT('Ctrl Pts',(0.631291674499274,-1.54176094830162,
16.7898335342867));
#57863=CARTESIAN_POINT('Ctrl Pts',(0.688277733083706,-1.51842735408488,
16.7939599237751));
#57864=CARTESIAN_POINT('Ctrl Pts',(0.744072594574505,-1.49188719483812,
16.7980863132635));
#57865=CARTESIAN_POINT('Ctrl Pts',(0.798288913299178,-1.46228957833379,
16.8022127027519));
#57866=CARTESIAN_POINT('Ctrl Pts',(0.851135254615892,-1.43343985594869,
16.806234823627));
#57867=CARTESIAN_POINT('Ctrl Pts',(0.902481401571002,-1.40168564426234,
16.810256944502));
#57868=CARTESIAN_POINT('Ctrl Pts',(0.951988994920911,-1.36721357276377,
16.814279065377));
#57869=CARTESIAN_POINT('Ctrl Pts',(1.00146770267854,-1.33276161426474,16.8182988395142));
#57870=CARTESIAN_POINT('Ctrl Pts',(1.04910955271808,-1.29559523597842,16.8223186136514));
#57871=CARTESIAN_POINT('Ctrl Pts',(1.09460394209619,-1.25594514607425,16.8263383877886));
#57872=CARTESIAN_POINT('Ctrl Pts',(1.14008955967749,-1.21630270112449,16.830357386871));
#57873=CARTESIAN_POINT('Ctrl Pts',(1.18342814320243,-1.17417783877431,16.8343763859534));
#57874=CARTESIAN_POINT('Ctrl Pts',(1.22434282064919,-1.12984098771676,16.8383953850359));
#57875=CARTESIAN_POINT('Ctrl Pts',(1.26716079963126,-1.08344163972767,16.8426013431169));
#57876=CARTESIAN_POINT('Ctrl Pts',(1.30732337160491,-1.03461988625231,16.846807301198));
#57877=CARTESIAN_POINT('Ctrl Pts',(1.34455918892583,-0.983725870085312,
16.851013259279));
#57878=CARTESIAN_POINT('Ctrl Pts',(1.3801943417479,-0.93501964649934,16.855038414889));
#57879=CARTESIAN_POINT('Ctrl Pts',(1.41314900460982,-0.884416188042298,
16.859063570499));
#57880=CARTESIAN_POINT('Ctrl Pts',(1.44323049791081,-0.832251001741727,
16.8630887261089));
#57881=CARTESIAN_POINT('Ctrl Pts',(1.47333651729113,-0.780043284058683,
16.8671171635136));
#57882=CARTESIAN_POINT('Ctrl Pts',(1.50056447979353,-0.726271776394919,
16.8711456009183));
#57883=CARTESIAN_POINT('Ctrl Pts',(1.52476908460097,-0.671293705202969,
16.875174038323));
#57884=CARTESIAN_POINT('Ctrl Pts',(1.54901902426344,-0.616212660923562,
16.8792100209294));
#57885=CARTESIAN_POINT('Ctrl Pts',(1.57023414275995,-0.559921038899605,
16.8832460035358));
#57886=CARTESIAN_POINT('Ctrl Pts',(1.58831881229225,-0.502791557724004,
16.8872819861422));
#57887=CARTESIAN_POINT('Ctrl Pts',(1.59068604399918,-0.495313471436753,
16.8878102847643));
#57888=CARTESIAN_POINT('Ctrl Pts',(1.59299971048392,-0.48782104170286,16.8883385833864));
#57889=CARTESIAN_POINT('Ctrl Pts',(1.59525966256195,-0.480315114276783,
16.8888668820084));
#57890=CARTESIAN_POINT('Ctrl Pts',(1.61318955219974,-0.42076497970229,16.8930582699947));
#57891=CARTESIAN_POINT('Ctrl Pts',(1.62781101013488,-0.360109450417287,
16.897249657981));
#57892=CARTESIAN_POINT('Ctrl Pts',(1.6389970149018,-0.298738656927739,16.9014410459673));
#57893=CARTESIAN_POINT('Ctrl Pts',(1.65015919995767,-0.237498547681441,
16.9056235087249));
#57894=CARTESIAN_POINT('Ctrl Pts',(1.65790039706353,-0.175546669803257,
16.9098059714826));
#57895=CARTESIAN_POINT('Ctrl Pts',(1.66214386045146,-0.11328630616063,16.9139884342402));
#57896=CARTESIAN_POINT('Ctrl Pts',(1.66638197605736,-0.0511044055146698,
16.9181656260912));
#57897=CARTESIAN_POINT('Ctrl Pts',(1.66713107917674,0.0113847355010989,
16.9223428179422));
#57898=CARTESIAN_POINT('Ctrl Pts',(1.66436591304727,0.0737706410865663,
16.9265200097932));
#57899=CARTESIAN_POINT('Ctrl Pts',(1.66160341949632,0.136096249668811,16.9306931643196));
#57900=CARTESIAN_POINT('Ctrl Pts',(1.65533342493368,0.198318345883009,16.934866318846));
#57901=CARTESIAN_POINT('Ctrl Pts',(1.64558271333189,0.260026024819162,16.9390394733724));
#57902=CARTESIAN_POINT('Ctrl Pts',(1.63583856579119,0.321692162892365,16.9432098185817));
#57903=CARTESIAN_POINT('Ctrl Pts',(1.62261843225166,0.38284410133519,16.947380163791));
#57904=CARTESIAN_POINT('Ctrl Pts',(1.60600078445904,0.443077284812664,16.9515505090003));
#57905=CARTESIAN_POINT('Ctrl Pts',(1.58938439684669,0.503305900575694,16.9557205379562));
#57906=CARTESIAN_POINT('Ctrl Pts',(1.56937112107116,0.562615436229024,16.9598905669121));
#57907=CARTESIAN_POINT('Ctrl Pts',(1.5460899908123,0.620614002669949,16.964060595868));
#57908=CARTESIAN_POINT('Ctrl Pts',(1.52281185651521,0.678605105491798,16.9682300881985));
#57909=CARTESIAN_POINT('Ctrl Pts',(1.49626688725886,0.735285133471823,16.972399580529));
#57910=CARTESIAN_POINT('Ctrl Pts',(1.46663246192064,0.790281735611163,16.9765690728594));
#57911=CARTESIAN_POINT('Ctrl Pts',(1.43697562604361,0.845319928011596,16.9807417182988));
#57912=CARTESIAN_POINT('Ctrl Pts',(1.40422489523102,0.898671731071445,16.9849143637381));
#57913=CARTESIAN_POINT('Ctrl Pts',(1.3686034211478,0.949989829220572,16.9890870091775));
#57914=CARTESIAN_POINT('Ctrl Pts',(1.33754903567419,0.994728348406303,16.992724672785));
#57915=CARTESIAN_POINT('Ctrl Pts',(1.30431365841565,1.03792146822267,16.9963623363925));
#57916=CARTESIAN_POINT('Ctrl Pts',(1.26907087985245,1.07935865304843,17.));
#57917=CARTESIAN_POINT('',(-1.26912595136393,1.07929389860899,16.9999994389445));
#57918=CARTESIAN_POINT('Origin',(0.,0.,17.));
#57919=CARTESIAN_POINT('',(-1.66599973263063,0.000943861575540272,16.3785196366098));
#57920=CARTESIAN_POINT('Ctrl Pts',(-1.26912595136393,1.07929389860899,16.9999994389445));
#57921=CARTESIAN_POINT('Ctrl Pts',(-1.22994842185412,1.12536218406424,16.9959304579992));
#57922=CARTESIAN_POINT('Ctrl Pts',(-1.18817697004422,1.16939124983374,16.9918614770539));
#57923=CARTESIAN_POINT('Ctrl Pts',(-1.14405250554583,1.2110738476882,16.9877924961086));
#57924=CARTESIAN_POINT('Ctrl Pts',(-1.10000544393575,1.25268332616314,16.9837306529468));
#57925=CARTESIAN_POINT('Ctrl Pts',(-1.05361393425504,1.29195415756655,16.9796688097851));
#57926=CARTESIAN_POINT('Ctrl Pts',(-1.00515803396106,1.3286133097194,16.9756069666233));
#57927=CARTESIAN_POINT('Ctrl Pts',(-0.956749692797827,1.36523648116815,
16.9715491101325));
#57928=CARTESIAN_POINT('Ctrl Pts',(-0.906281384132347,1.39925274411531,
16.9674912536418));
#57929=CARTESIAN_POINT('Ctrl Pts',(-0.854067547829918,1.43042812603213,
16.963433397151));
#57930=CARTESIAN_POINT('Ctrl Pts',(-0.801885346769847,1.46158461945439,
16.9593779992283));
#57931=CARTESIAN_POINT('Ctrl Pts',(-0.747960155455131,1.48990338113144,
16.9553226013056));
#57932=CARTESIAN_POINT('Ctrl Pts',(-0.692635054495748,1.51519394180536,
16.951267203383));
#57933=CARTESIAN_POINT('Ctrl Pts',(-0.637322693849749,1.54047867854651,
16.9472127393409));
#57934=CARTESIAN_POINT('Ctrl Pts',(-0.580611531137159,1.56273638502247,
16.9431582752989));
#57935=CARTESIAN_POINT('Ctrl Pts',(-0.522866967902763,1.58182367344662,
16.9391038112569));
#57936=CARTESIAN_POINT('Ctrl Pts',(-0.465072383772699,1.60092749612456,
16.9350458350587));
#57937=CARTESIAN_POINT('Ctrl Pts',(-0.406243099257206,1.6168552492843,16.9309878588605));
#57938=CARTESIAN_POINT('Ctrl Pts',(-0.346760899012902,1.62951308031441,
16.9269298826623));
#57939=CARTESIAN_POINT('Ctrl Pts',(-0.287255151962042,1.64217592211241,
16.9228703000612));
#57940=CARTESIAN_POINT('Ctrl Pts',(-0.22709648298635,1.65156618061866,16.9188107174601));
#57941=CARTESIAN_POINT('Ctrl Pts',(-0.166675032253898,1.65764152747908,
16.914751134859));
#57942=CARTESIAN_POINT('Ctrl Pts',(-0.10613950514824,1.66372834466215,16.9106838877206));
#57943=CARTESIAN_POINT('Ctrl Pts',(-0.0453407203907892,1.66648771915369,
16.9066166405823));
#57944=CARTESIAN_POINT('Ctrl Pts',(0.0153287726306612,1.66592947891849,
16.9025493934439));
#57945=CARTESIAN_POINT('Ctrl Pts',(0.0725281121846614,1.66540316872245,
16.8987147833536));
#57946=CARTESIAN_POINT('Ctrl Pts',(0.12961217485131,1.66192841223509,16.8948801732632));
#57947=CARTESIAN_POINT('Ctrl Pts',(0.186257995909159,1.65555548350392,16.8910455631728));
#57948=CARTESIAN_POINT('Ctrl Pts',(0.246594300095448,1.64876735757865,16.8869611277012));
#57949=CARTESIAN_POINT('Ctrl Pts',(0.306678665411954,1.63866307257685,16.8828766922296));
#57950=CARTESIAN_POINT('Ctrl Pts',(0.366119211224653,1.62527312263885,16.878792256758));
#57951=CARTESIAN_POINT('Ctrl Pts',(0.426077211242961,1.61176660772296,16.874672264609));
#57952=CARTESIAN_POINT('Ctrl Pts',(0.485379598637478,1.59491692193667,16.8705522724599));
#57953=CARTESIAN_POINT('Ctrl Pts',(0.543629176032988,1.57480897856397,16.8664322803109));
#57954=CARTESIAN_POINT('Ctrl Pts',(0.601222363844623,1.55492762300826,16.8623587145919));
#57955=CARTESIAN_POINT('Ctrl Pts',(0.657785852831911,1.53186123201388,16.858285148873));
#57956=CARTESIAN_POINT('Ctrl Pts',(0.712948172994938,1.50574264156368,16.854211583154));
#57957=CARTESIAN_POINT('Ctrl Pts',(0.768078355465295,1.47963926786345,16.8501403907037));
#57958=CARTESIAN_POINT('Ctrl Pts',(0.82180852794464,1.45048743872728,16.8460691982534));
#57959=CARTESIAN_POINT('Ctrl Pts',(0.873787549594841,1.41846794753108,16.841998005803));
#57960=CARTESIAN_POINT('Ctrl Pts',(0.925755402865265,1.38645533614575,16.8379276881022));
#57961=CARTESIAN_POINT('Ctrl Pts',(0.975972418486816,1.35157655348069,16.8338573704014));
#57962=CARTESIAN_POINT('Ctrl Pts',(1.02411421476585,1.3140571049671,16.8297870527005));
#57963=CARTESIAN_POINT('Ctrl Pts',(1.07327199087348,1.27574584962835,16.8256308354073));
#57964=CARTESIAN_POINT('Ctrl Pts',(1.12026548795328,1.23468149423282,16.821474618114));
#57965=CARTESIAN_POINT('Ctrl Pts',(1.16478467374162,1.19114762469504,16.8173184008207));
#57966=CARTESIAN_POINT('Ctrl Pts',(1.2084410523779,1.14845746631973,16.8132427333835));
#57967=CARTESIAN_POINT('Ctrl Pts',(1.24971787740482,1.10339310045069,16.8091670659462));
#57968=CARTESIAN_POINT('Ctrl Pts',(1.28836173824702,1.05625755922555,16.805091398509));
#57969=CARTESIAN_POINT('Ctrl Pts',(1.32815121173139,1.00772466611202,16.8008949062877));
#57970=CARTESIAN_POINT('Ctrl Pts',(1.36514876678207,0.956996299983976,16.7966984140664));
#57971=CARTESIAN_POINT('Ctrl Pts',(1.39912564197979,0.904435424977723,16.7925019218451));
#57972=CARTESIAN_POINT('Ctrl Pts',(1.43310251717751,0.851874549971471,16.7883054296238));
#57973=CARTESIAN_POINT('Ctrl Pts',(1.46405848535841,0.797481706777552,16.7841089374025));
#57974=CARTESIAN_POINT('Ctrl Pts',(1.49181736902974,0.74164475152272,16.7799124451812));
#57975=CARTESIAN_POINT('Ctrl Pts',(1.51875202292534,0.687465733296311,16.7758405571725));
#57976=CARTESIAN_POINT('Ctrl Pts',(1.54278840870396,0.631702727019054,16.7717686691638));
#57977=CARTESIAN_POINT('Ctrl Pts',(1.5637384297878,0.574698288847972,16.7676967811551));
#57978=CARTESIAN_POINT('Ctrl Pts',(1.58494401817936,0.516998458976165,16.7635752205732));
#57979=CARTESIAN_POINT('Ctrl Pts',(1.60298711135448,0.458027136740834,16.7594536599913));
#57980=CARTESIAN_POINT('Ctrl Pts',(1.61772077496127,0.398165159523934,16.7553320994094));
#57981=CARTESIAN_POINT('Ctrl Pts',(1.63223606105954,0.339190436813987,16.7512716272408));
#57982=CARTESIAN_POINT('Ctrl Pts',(1.64353922624071,0.279351797244359,16.7472111550721));
#57983=CARTESIAN_POINT('Ctrl Pts',(1.65153912632907,0.219030852174293,16.7431506829035));
#57984=CARTESIAN_POINT('Ctrl Pts',(1.65953402056102,0.158747652324369,16.7390927515342));
#57985=CARTESIAN_POINT('Ctrl Pts',(1.66422968007249,0.0979832532653026,
16.7350348201648));
#57986=CARTESIAN_POINT('Ctrl Pts',(1.6655862263422,0.0371284610395597,16.7309768887955));
#57987=CARTESIAN_POINT('Ctrl Pts',(1.66694243148425,-0.0237110281677983,
16.7269199778651));
#57988=CARTESIAN_POINT('Ctrl Pts',(1.66496117857875,-0.084640352251613,
16.7228630669347));
#57989=CARTESIAN_POINT('Ctrl Pts',(1.65965465703569,-0.145266718073181,
16.7188061560042));
#57990=CARTESIAN_POINT('Ctrl Pts',(1.65420164838393,-0.20756668136684,16.714637253603));
#57991=CARTESIAN_POINT('Ctrl Pts',(1.64523705565621,-0.269546140949339,
16.7104683512018));
#57992=CARTESIAN_POINT('Ctrl Pts',(1.63283108802485,-0.33078488172765,16.7062994488006));
#57993=CARTESIAN_POINT('Ctrl Pts',(1.62074308199887,-0.390454090091595,
16.7022373942439));
#57994=CARTESIAN_POINT('Ctrl Pts',(1.60538821254725,-0.449419604041255,
16.6981753396871));
#57995=CARTESIAN_POINT('Ctrl Pts',(1.58688266513795,-0.507306029024575,
16.6941132851304));
#57996=CARTESIAN_POINT('Ctrl Pts',(1.5676469658471,-0.567476411417106,16.6898909588069));
#57997=CARTESIAN_POINT('Ctrl Pts',(1.5450069606227,-0.626480190402658,16.6856686324835));
#57998=CARTESIAN_POINT('Ctrl Pts',(1.51914792966687,-0.683919269935332,
16.68144630616));
#57999=CARTESIAN_POINT('Ctrl Pts',(1.49328889871103,-0.741358349468007,
16.6772239798366));
#58000=CARTESIAN_POINT('Ctrl Pts',(1.46421119230165,-0.797232218796164,
16.6730016535131));
#58001=CARTESIAN_POINT('Ctrl Pts',(1.43215137988136,-0.851174732416276,
16.6687793271897));
#58002=CARTESIAN_POINT('Ctrl Pts',(1.40118335205646,-0.903280254458425,
16.664700790567));
#58003=CARTESIAN_POINT('Ctrl Pts',(1.3673043206305,-0.953800681650137,16.6606222539444));
#58004=CARTESIAN_POINT('Ctrl Pts',(1.33070163494553,-1.00239171921624,16.6565437173218));
#58005=CARTESIAN_POINT('Ctrl Pts',(1.29372029069739,-1.0514854360837,16.6524229878166));
#58006=CARTESIAN_POINT('Ctrl Pts',(1.25395880785184,-1.0986091161508,16.6483022583115));
#58007=CARTESIAN_POINT('Ctrl Pts',(1.21165761114675,-1.14343422781993,16.6441815288063));
#58008=CARTESIAN_POINT('Ctrl Pts',(1.16990475502701,-1.18767828198039,16.6401142153604));
#58009=CARTESIAN_POINT('Ctrl Pts',(1.12567799822337,-1.22968262235875,16.6360469019145));
#58010=CARTESIAN_POINT('Ctrl Pts',(1.07924983827964,-1.26916341996347,16.6319795884686));
#58011=CARTESIAN_POINT('Ctrl Pts',(1.03285007551824,-1.30862006965,16.6279147627422));
#58012=CARTESIAN_POINT('Ctrl Pts',(0.984251968266631,-1.34555590618184,
16.6238499370159));
#58013=CARTESIAN_POINT('Ctrl Pts',(0.933763464755579,-1.37972525956716,
16.6197851112895));
#58014=CARTESIAN_POINT('Ctrl Pts',(0.883287115387296,-1.41388638733337,
16.6157212640923));
#58015=CARTESIAN_POINT('Ctrl Pts',(0.830921696685062,-1.44528206742015,
16.6116574168951));
#58016=CARTESIAN_POINT('Ctrl Pts',(0.777004998512594,-1.47370934457458,
16.6075935696979));
#58017=CARTESIAN_POINT('Ctrl Pts',(0.721782352132463,-1.50282517560763,
16.6034312896562));
#58018=CARTESIAN_POINT('Ctrl Pts',(0.664932764798376,-1.52882661656567,
16.5992690096146));
#58019=CARTESIAN_POINT('Ctrl Pts',(0.60684467049248,-1.55154617910485,16.5951067295729));
#58020=CARTESIAN_POINT('Ctrl Pts',(0.550058163190383,-1.57375666163915,
16.5910377142471));
#58021=CARTESIAN_POINT('Ctrl Pts',(0.492088600762408,-1.59283072759248,
16.5869686989213));
#58022=CARTESIAN_POINT('Ctrl Pts',(0.433315430431083,-1.60866209557829,
16.5828996835955));
#58023=CARTESIAN_POINT('Ctrl Pts',(0.372521576006573,-1.62503776282993,
16.5786907711959));
#58024=CARTESIAN_POINT('Ctrl Pts',(0.310868422187777,-1.63794352541022,
16.5744818587964));
#58025=CARTESIAN_POINT('Ctrl Pts',(0.248785745245518,-1.64731953578006,
16.5702729463968));
#58026=CARTESIAN_POINT('Ctrl Pts',(0.186703068303259,-1.6566955461499,16.5660640339973));
#58027=CARTESIAN_POINT('Ctrl Pts',(0.124191470175191,-1.66254182005321,
16.5618551215977));
#58028=CARTESIAN_POINT('Ctrl Pts',(0.0616817819915773,-1.66485775902037,
16.5576462091981));
#58029=CARTESIAN_POINT('Ctrl Pts',(0.00111348529636081,-1.66710177082986,
16.5535680148832));
#58030=CARTESIAN_POINT('Ctrl Pts',(-0.0597018689058509,-1.66604082959472,
16.5494898205682));
#58031=CARTESIAN_POINT('Ctrl Pts',(-0.120373454774682,-1.66164563953498,
16.5454116262532));
#58032=CARTESIAN_POINT('Ctrl Pts',(-0.181678476249575,-1.65720456193432,
16.5412908539596));
#58033=CARTESIAN_POINT('Ctrl Pts',(-0.242836186736639,-1.64935910138759,
16.537170081666));
#58034=CARTESIAN_POINT('Ctrl Pts',(-0.303440114899917,-1.63813311323272,
16.5330493093724));
#58035=CARTESIAN_POINT('Ctrl Pts',(-0.363253339565518,-1.62705359129494,
16.5289823010701));
#58036=CARTESIAN_POINT('Ctrl Pts',(-0.4225266283128,-1.61268132204695,16.5249152927678));
#58037=CARTESIAN_POINT('Ctrl Pts',(-0.480873786340675,-1.59509134585151,
16.5208482844654));
#58038=CARTESIAN_POINT('Ctrl Pts',(-0.539185467190902,-1.57751206499636,
16.5167837490509));
#58039=CARTESIAN_POINT('Ctrl Pts',(-0.596571644913312,-1.55671910379626,
16.5127192136364));
#58040=CARTESIAN_POINT('Ctrl Pts',(-0.652658965974062,-1.53283798039247,
16.5086546782219));
#58041=CARTESIAN_POINT('Ctrl Pts',(-0.708732996213481,-1.50896251601711,
16.5045911059665));
#58042=CARTESIAN_POINT('Ctrl Pts',(-0.763508310206096,-1.48200054257006,
16.5005275337111));
#58043=CARTESIAN_POINT('Ctrl Pts',(-0.816631266028351,-1.45212581250556,
16.4964639614557));
#58044=CARTESIAN_POINT('Ctrl Pts',(-0.871048449291931,-1.42152324840296,
16.4923013889349));
#58045=CARTESIAN_POINT('Ctrl Pts',(-0.923731189381291,-1.38786436356937,
16.4881388164141));
#58046=CARTESIAN_POINT('Ctrl Pts',(-0.974328052070879,-1.35138478863267,
16.4839762438934));
#58047=CARTESIAN_POINT('Ctrl Pts',(-1.02378487283793,-1.3157271667289,16.4799074619147));
#58048=CARTESIAN_POINT('Ctrl Pts',(-1.07124847497301,-1.27737503321648,
16.475838679936));
#58049=CARTESIAN_POINT('Ctrl Pts',(-1.11642386732308,-1.23658956346533,
16.4717698979574));
#58050=CARTESIAN_POINT('Ctrl Pts',(-1.16316128409206,-1.19439385915121,
16.4675604301656));
#58051=CARTESIAN_POINT('Ctrl Pts',(-1.20744890033411,-1.14959385170369,
16.4633509623737));
#58052=CARTESIAN_POINT('Ctrl Pts',(-1.24900330896305,-1.10251836002824,
16.4591414945819));
#58053=CARTESIAN_POINT('Ctrl Pts',(-1.29055771759198,-1.05544286835279,
16.4549320267901));
#58054=CARTESIAN_POINT('Ctrl Pts',(-1.32937860532145,-1.00609240745467,
16.4507225589984));
#58055=CARTESIAN_POINT('Ctrl Pts',(-1.36523182155122,-0.95482881891151,
16.4465130912066));
#58056=CARTESIAN_POINT('Ctrl Pts',(-1.40035050925344,-0.904615472778063,
16.4423898632142));
#58057=CARTESIAN_POINT('Ctrl Pts',(-1.43276572108851,-0.852361594770622,
16.4382666352219));
#58058=CARTESIAN_POINT('Ctrl Pts',(-1.4622365877862,-0.798385972659444,
16.4341434072296));
#58059=CARTESIAN_POINT('Ctrl Pts',(-1.49165868478443,-0.744499671805606,
16.4300270025382));
#58060=CARTESIAN_POINT('Ctrl Pts',(-1.5181458679218,-0.688897712197785,
16.4259105978467));
#58061=CARTESIAN_POINT('Ctrl Pts',(-1.54150011838769,-0.631928306859823,
16.4217941931553));
#58062=CARTESIAN_POINT('Ctrl Pts',(-1.56481949600417,-0.575043968927322,
16.4176839351291));
#58063=CARTESIAN_POINT('Ctrl Pts',(-1.58501504776261,-0.51679669915394,
16.413573677103));
#58064=CARTESIAN_POINT('Ctrl Pts',(-1.60193531728544,-0.457557908065854,
16.4094634190768));
#58065=CARTESIAN_POINT('Ctrl Pts',(-1.61884077099301,-0.398370987959132,
16.4053567600964));
#58066=CARTESIAN_POINT('Ctrl Pts',(-1.63247649805755,-0.338194745709455,
16.401250101116));
#58067=CARTESIAN_POINT('Ctrl Pts',(-1.64274022962142,-0.277417623779323,
16.3971434421355));
#58068=CARTESIAN_POINT('Ctrl Pts',(-1.65299927914237,-0.216668226764991,
16.3930386565043));
#58069=CARTESIAN_POINT('Ctrl Pts',(-1.65988930117611,-0.155318983035484,
16.3889338708731));
#58070=CARTESIAN_POINT('Ctrl Pts',(-1.66335908145097,-0.0937686842958181,
16.3848290852419));
#58071=CARTESIAN_POINT('Ctrl Pts',(-1.66513687631255,-0.0622324496759222,
16.3827259356979));
#58072=CARTESIAN_POINT('Ctrl Pts',(-1.66601762828668,-0.030643564989622,
16.3806227861538));
#58073=CARTESIAN_POINT('Ctrl Pts',(-1.66599973263063,0.000943861575540161,
16.3785196366098));
#58074=CARTESIAN_POINT('Ctrl Pts',(-1.66599977577897,0.000864352024730958,
16.3772626675068));
#58075=CARTESIAN_POINT('Ctrl Pts',(-1.66598176046584,0.0355880603993911,
16.3750662024614));
#58076=CARTESIAN_POINT('Ctrl Pts',(-1.66487815818066,0.0703044066738621,
16.3728974757554));
#58077=CARTESIAN_POINT('Ctrl Pts',(-1.65355857415653,0.249615190627302,
16.3617715086377));
#58078=CARTESIAN_POINT('Ctrl Pts',(-1.62559135098946,0.392435847117513,
16.353215676586));
#58079=CARTESIAN_POINT('Ctrl Pts',(-1.57468444189208,0.544201338787872,
16.3429390992582));
#58080=CARTESIAN_POINT('Ctrl Pts',(-1.56966340724548,0.558518523640452,
16.3419568924473));
#58081=CARTESIAN_POINT('Ctrl Pts',(-1.56410974302841,0.573687788191105,
16.3409005954565));
#58082=CARTESIAN_POINT('Ctrl Pts',(-1.56377092917891,0.5746106922007,16.3408362679555));
#58083=CARTESIAN_POINT('Ctrl Pts',(-1.5634313003322,0.575533291080154,16.3407718992107));
#58084=CARTESIAN_POINT('Origin',(0.,0.,11.));
#58085=CARTESIAN_POINT('Ctrl Pts',(-1.5634313003322,0.575533291080154,16.3407718992107));
#58086=CARTESIAN_POINT('Ctrl Pts',(-1.5596751818211,0.585736755135203,16.3400600143508));
#58087=CARTESIAN_POINT('Ctrl Pts',(-1.55581937928052,0.595902898087225,
16.3393430849936));
#58088=CARTESIAN_POINT('Ctrl Pts',(-1.54953271929507,0.612001177017325,
16.3381945028787));
#58089=CARTESIAN_POINT('Ctrl Pts',(-1.54716658128151,0.617958457471911,
16.337766540049));
#58090=CARTESIAN_POINT('Ctrl Pts',(-1.54271375868244,0.628983541257041,
16.3369688152863));
#58091=CARTESIAN_POINT('Ctrl Pts',(-1.5406363744731,0.63405488308338,16.3365996022725));
#58092=CARTESIAN_POINT('Ctrl Pts',(-1.53580697175768,0.645680632261762,
16.3357480258034));
#58093=CARTESIAN_POINT('Ctrl Pts',(-1.5330379906436,0.652227757754035,16.3352646742868));
#58094=CARTESIAN_POINT('Ctrl Pts',(-1.52398741590083,0.673251352442413,
16.3337008347677));
#58095=CARTESIAN_POINT('Ctrl Pts',(-1.51754222414108,0.687655858829796,
16.3326113405556));
#58096=CARTESIAN_POINT('Ctrl Pts',(-1.47506563651353,0.779081385328623,
16.3255903036547));
#58097=CARTESIAN_POINT('Ctrl Pts',(-1.43338959935601,0.853333434232536,
16.3194096914169));
#58098=CARTESIAN_POINT('Ctrl Pts',(-1.33810517651707,0.996272953350723,
16.3069050407079));
#58099=CARTESIAN_POINT('Ctrl Pts',(-1.28440454911611,1.06460927430752,16.3006011100336));
#58100=CARTESIAN_POINT('Ctrl Pts',(-1.20238508189192,1.15369095019632,16.2920412026584));
#58101=CARTESIAN_POINT('Ctrl Pts',(-1.17837503721039,1.17820424602859,16.2896433181791));
#58102=CARTESIAN_POINT('Ctrl Pts',(-1.1406777197705,1.21438557640963,16.2860384808385));
#58103=CARTESIAN_POINT('Ctrl Pts',(-1.1275314136631,1.22660137899651,16.2848091794439));
#58104=CARTESIAN_POINT('Ctrl Pts',(-1.10366785957624,1.24806792941671,16.2826262602532));
#58105=CARTESIAN_POINT('Ctrl Pts',(-1.0930254053607,1.2573988171632,16.2816693704768));
#58106=CARTESIAN_POINT('Ctrl Pts',(-1.07452386928761,1.2732078122323,16.2800337175353));
#58107=CARTESIAN_POINT('Ctrl Pts',(-1.06672206724027,1.27975142821405,16.2793522830947));
#58108=CARTESIAN_POINT('Ctrl Pts',(-1.05128618179399,1.29245874889821,16.2780199932486));
#58109=CARTESIAN_POINT('Ctrl Pts',(-1.04365668530581,1.29862734603498,16.2773689563997));
#58110=CARTESIAN_POINT('Ctrl Pts',(-1.02602338943884,1.31262843609015,16.2758810190201));
#58111=CARTESIAN_POINT('Ctrl Pts',(-1.01598351460997,1.3204146772117,16.2750459779494));
#58112=CARTESIAN_POINT('Ctrl Pts',(-0.983305106142277,1.34516440240364,
16.2723658183722));
#58113=CARTESIAN_POINT('Ctrl Pts',(-0.960322586195843,1.36166694997056,
16.270538518761));
#58114=CARTESIAN_POINT('Ctrl Pts',(-0.828766951679072,1.45114172645287,
16.2603706945963));
#58115=CARTESIAN_POINT('Ctrl Pts',(-0.712318860826929,1.51171136037505,
16.2525049832914));
#58116=CARTESIAN_POINT('Ctrl Pts',(-0.5232989193757,1.58328704946123,16.2401028110993));
#58117=CARTESIAN_POINT('Ctrl Pts',(-0.455074915546771,1.60422695859791,
16.2356823671256));
#58118=CARTESIAN_POINT('Ctrl Pts',(-0.370389081873657,1.62438189899929,
16.2300342330036));
#58119=CARTESIAN_POINT('Ctrl Pts',(-0.35499928173187,1.62781451385597,16.2290013757046));
#58120=CARTESIAN_POINT('Ctrl Pts',(-0.332529616665705,1.6324924741088,16.2274809407806));
#58121=CARTESIAN_POINT('Ctrl Pts',(-0.325486219314668,1.63391136242929,
16.2270025738289));
#58122=CARTESIAN_POINT('Ctrl Pts',(-0.313103139612887,1.63632268208565,
16.226158097851));
#58123=CARTESIAN_POINT('Ctrl Pts',(-0.307767451668835,1.63733462993636,
16.2257930906287));
#58124=CARTESIAN_POINT('Ctrl Pts',(-0.296101873344028,1.63948804455173,
16.2249924947713));
#58125=CARTESIAN_POINT('Ctrl Pts',(-0.289770390740234,1.64061893344611,
16.2245563552223));
#58126=CARTESIAN_POINT('Ctrl Pts',(-0.271997035398465,1.64368740457005,
16.2233278209827));
#58127=CARTESIAN_POINT('Ctrl Pts',(-0.260541495744583,1.64554209347455,
16.2225310837502));
#58128=CARTESIAN_POINT('Ctrl Pts',(-0.172913650200842,1.65879140546173,
16.216403845967));
#58129=CARTESIAN_POINT('Ctrl Pts',(-0.0960608530939728,1.66500981384815,
16.2108459440849));
#58130=CARTESIAN_POINT('Ctrl Pts',(0.0382465198165494,1.66654675091026,
16.201082994383));
#58131=CARTESIAN_POINT('Ctrl Pts',(0.0955535879539751,1.66424476838058,
16.1969006866591));
#58132=CARTESIAN_POINT('Ctrl Pts',(0.234929027541468,1.65142212402918,16.1867871594149));
#58133=CARTESIAN_POINT('Ctrl Pts',(0.316561551960156,1.6377359516911,16.1809183473741));
#58134=CARTESIAN_POINT('Ctrl Pts',(0.419014875669339,1.61260760863278,16.1736662188044));
#58135=CARTESIAN_POINT('Ctrl Pts',(0.441065139923292,1.60671665123273,16.1721116609777));
#58136=CARTESIAN_POINT('Ctrl Pts',(0.474338544037795,1.5970906529115,16.1697743013292));
#58137=CARTESIAN_POINT('Ctrl Pts',(0.485653688611424,1.59368632898281,16.1689809336961));
#58138=CARTESIAN_POINT('Ctrl Pts',(0.50529136332725,1.58754947731895,16.1676063333909));
#58139=CARTESIAN_POINT('Ctrl Pts',(0.513630214831017,1.5848711973619,16.1670233585435));
#58140=CARTESIAN_POINT('Ctrl Pts',(0.532389195516748,1.57868256314659,16.1657133631261));
#58141=CARTESIAN_POINT('Ctrl Pts',(0.542796542188667,1.57513453845384,16.1649876094402));
#58142=CARTESIAN_POINT('Ctrl Pts',(0.570955478127548,1.56522248614719,16.1630262024345));
#58143=CARTESIAN_POINT('Ctrl Pts',(0.588635713278688,1.55865956294998,16.1617971485567));
#58144=CARTESIAN_POINT('Ctrl Pts',(0.698772396141887,1.51563526677497,16.1541487860599));
#58145=CARTESIAN_POINT('Ctrl Pts',(0.787927247882166,1.47126049869444,16.1480087233898));
#58146=CARTESIAN_POINT('Ctrl Pts',(0.934029298937868,1.38142852256875,16.1375182314248));
#58147=CARTESIAN_POINT('Ctrl Pts',(0.992935519331589,1.33971406897554,16.1331457893078));
#58148=CARTESIAN_POINT('Ctrl Pts',(1.0772338415564,1.27139627062114,16.1264047918402));
#58149=CARTESIAN_POINT('Ctrl Pts',(1.10475525404588,1.24755629712246,16.1241171670876));
#58150=CARTESIAN_POINT('Ctrl Pts',(1.14813637325292,1.20741638597222,16.1203253707562));
#58151=CARTESIAN_POINT('Ctrl Pts',(1.1644828967793,1.19165889448185,16.1188506610842));
#58152=CARTESIAN_POINT('Ctrl Pts',(1.18634261120009,1.16970754298156,16.1168060870542));
#58153=CARTESIAN_POINT('Ctrl Pts',(1.19213991773492,1.16379849488765,16.1162566467879));
#58154=CARTESIAN_POINT('Ctrl Pts',(1.20181563649455,1.15378812444936,16.1153268962671));
#58155=CARTESIAN_POINT('Ctrl Pts',(1.20571777840392,1.14970974505162,16.1149483859604));
#58156=CARTESIAN_POINT('Ctrl Pts',(1.21317965095335,1.14183109410893,16.1142175427461));
#58157=CARTESIAN_POINT('Ctrl Pts',(1.21674240481423,1.13803384457583,16.1138654742685));
#58158=CARTESIAN_POINT('Ctrl Pts',(1.22637132325721,1.12767426173673,16.1129055922749));
#58159=CARTESIAN_POINT('Ctrl Pts',(1.23240247398457,1.12107983492308,16.1122952507489));
#58160=CARTESIAN_POINT('Ctrl Pts',(1.2555711095759,1.09533448785564,16.1099161056688));
#58161=CARTESIAN_POINT('Ctrl Pts',(1.27231668311415,1.07583759655167,16.1081222449568));
#58162=CARTESIAN_POINT('Ctrl Pts',(1.30944843376566,1.03052528691497,16.1039854241299));
#58163=CARTESIAN_POINT('Ctrl Pts',(1.32953449900069,1.0044776504301,16.1016301935625));
#58164=CARTESIAN_POINT('Ctrl Pts',(1.40791337936918,0.896363157284946,16.0919941636001));
#58165=CARTESIAN_POINT('Ctrl Pts',(1.45948876182478,0.809679781911558,16.0845993433231));
#58166=CARTESIAN_POINT('Ctrl Pts',(1.53411461682059,0.653661612804416,16.0722053704864));
#58167=CARTESIAN_POINT('Ctrl Pts',(1.56103175088294,0.586484110963284,16.0671271700023));
#58168=CARTESIAN_POINT('Ctrl Pts',(1.58896530001192,0.501053174593697,16.060993625145));
#58169=CARTESIAN_POINT('Ctrl Pts',(1.59416379785365,0.484259057889517,16.0598026750488));
#58170=CARTESIAN_POINT('Ctrl Pts',(1.60210314870812,0.457095637132175,16.0578994014729));
#58171=CARTESIAN_POINT('Ctrl Pts',(1.60501127650194,0.446777049745986,16.0571816900023));
#58172=CARTESIAN_POINT('Ctrl Pts',(1.61038352746254,0.426985575868721,16.0558149154284));
#58173=CARTESIAN_POINT('Ctrl Pts',(1.61286415561316,0.417517676315472,16.0551653431425));
#58174=CARTESIAN_POINT('Ctrl Pts',(1.61833978438064,0.39584130934438,16.0536876171827));
#58175=CARTESIAN_POINT('Ctrl Pts',(1.6212803614347,0.383619608362693,16.0528612415448));
#58176=CARTESIAN_POINT('Ctrl Pts',(1.63022116991452,0.344519020885195,16.0502380834013));
#58177=CARTESIAN_POINT('Ctrl Pts',(1.6356935876534,0.317523299662902,16.0484580664242));
#58178=CARTESIAN_POINT('Ctrl Pts',(1.66345772601487,0.160682930608727,16.0382704817449));
#58179=CARTESIAN_POINT('Ctrl Pts',(1.67095466772995,0.0286993695304271,
16.0303496073671));
#58180=CARTESIAN_POINT('Ctrl Pts',(1.6584078496364,-0.1742573439718,16.0178749314143));
#58181=CARTESIAN_POINT('Ctrl Pts',(1.6493885162593,-0.245351559196319,16.0134373434482));
#58182=CARTESIAN_POINT('Ctrl Pts',(1.63283471860549,-0.331143800783455,
16.0077686461894));
#58183=CARTESIAN_POINT('Ctrl Pts',(1.62962228781726,-0.346607255649431,
16.0067341646853));
#58184=CARTESIAN_POINT('Ctrl Pts',(1.62462909819665,-0.36903649523775,16.0052119904229));
#58185=CARTESIAN_POINT('Ctrl Pts',(1.62302220252905,-0.376040645242056,
16.0047335524248));
#58186=CARTESIAN_POINT('Ctrl Pts',(1.62012200309603,-0.388317091618687,
16.003889177361));
#58187=CARTESIAN_POINT('Ctrl Pts',(1.61884816913838,-0.393593791318744,
16.0035243449801));
#58188=CARTESIAN_POINT('Ctrl Pts',(1.61601022311097,-0.405102756810232,
16.0027243667008));
#58189=CARTESIAN_POINT('Ctrl Pts',(1.61443586365921,-0.411332132735254,
16.0022886723204));
#58190=CARTESIAN_POINT('Ctrl Pts',(1.60992362620736,-0.428760979550803,
16.0010623999002));
#58191=CARTESIAN_POINT('Ctrl Pts',(1.60690503843422,-0.439938903227747,
16.0002675023798));
#58192=CARTESIAN_POINT('Ctrl Pts',(1.58444817028227,-0.51978135681164,15.994533467335));
#58193=CARTESIAN_POINT('Ctrl Pts',(1.5607341073769,-0.587158758958952,15.989398778818));
#58194=CARTESIAN_POINT('Ctrl Pts',(1.50512389920432,-0.717731764814795,
15.9790949468929));
#58195=CARTESIAN_POINT('Ctrl Pts',(1.47337094637055,-0.780842794460663,
15.9739373366074));
#58196=CARTESIAN_POINT('Ctrl Pts',(1.39564020274277,-0.913606965214696,
15.9628523993985));
#58197=CARTESIAN_POINT('Ctrl Pts',(1.34823689778213,-0.982217065223451,
15.9569715181899));
#58198=CARTESIAN_POINT('Ctrl Pts',(1.28448399660806,-1.06112509274721,15.9500427957919));
#58199=CARTESIAN_POINT('Ctrl Pts',(1.27284405116492,-1.07505984330685,15.948811976492));
#58200=CARTESIAN_POINT('Ctrl Pts',(1.25389048461862,-1.09701060592593,15.9468606740721));
#58201=CARTESIAN_POINT('Ctrl Pts',(1.24672260254013,-1.10514993501778,15.9461343075227));
#58202=CARTESIAN_POINT('Ctrl Pts',(1.23295457486604,-1.12047947623846,15.9447605974681));
#58203=CARTESIAN_POINT('Ctrl Pts',(1.22636976049133,-1.1276827824464,15.944112653882));
#58204=CARTESIAN_POINT('Ctrl Pts',(1.21117532206315,-1.14401388314916,15.9426377502655));
#58205=CARTESIAN_POINT('Ctrl Pts',(1.20252504840967,-1.15310318180862,15.941812567842));
#58206=CARTESIAN_POINT('Ctrl Pts',(1.17518414830009,-1.18118939320463,15.9392481609189));
#58207=CARTESIAN_POINT('Ctrl Pts',(1.15613932053274,-1.19983672384999,15.9375243764412));
#58208=CARTESIAN_POINT('Ctrl Pts',(1.03963477330174,-1.30855859217155,15.9273213014175));
#58209=CARTESIAN_POINT('Ctrl Pts',(0.932147522466384,-1.38718049697853,
15.9193412140275));
#58210=CARTESIAN_POINT('Ctrl Pts',(0.753791854511078,-1.48745527859235,
15.9067898586047));
#58211=CARTESIAN_POINT('Ctrl Pts',(0.688911179517107,-1.51859289395451,
15.9023345646746));
#58212=CARTESIAN_POINT('Ctrl Pts',(0.607551768587619,-1.55135014199792,
15.8966446220115));
#58213=CARTESIAN_POINT('Ctrl Pts',(0.592789604758586,-1.5570506910133,15.8956081481134));
#58214=CARTESIAN_POINT('Ctrl Pts',(0.5712030121663,-1.56503509722877,15.8940835102819));
#58215=CARTESIAN_POINT('Ctrl Pts',(0.564440938953634,-1.56748657357542,
15.8936046388506));
#58216=CARTESIAN_POINT('Ctrl Pts',(0.552546779376451,-1.57171165911844,
15.8927597427969));
#58217=CARTESIAN_POINT('Ctrl Pts',(0.54742157821759,-1.57350408237768,15.8923948266762));
#58218=CARTESIAN_POINT('Ctrl Pts',(0.536215203118022,-1.57736187971095,
15.8915949845681));
#58219=CARTESIAN_POINT('Ctrl Pts',(0.530130916038701,-1.57941712413163,
15.8911595129657));
#58220=CARTESIAN_POINT('Ctrl Pts',(0.513057847479166,-1.58507456443021,
15.8899344480605));
#58221=CARTESIAN_POINT('Ctrl Pts',(0.502043469565574,-1.58859751532859,
15.889140548208));
#58222=CARTESIAN_POINT('Ctrl Pts',(0.423874931369722,-1.61270563703923,
15.883485408586));
#58223=CARTESIAN_POINT('Ctrl Pts',(0.355521480077651,-1.62913832481023,
15.8784346555065));
#58224=CARTESIAN_POINT('Ctrl Pts',(0.271100589546626,-1.6438673618563,15.8722146725655));
#58225=CARTESIAN_POINT('Ctrl Pts',(0.255821020050752,-1.64631437835075,
15.871089465356));
#58226=CARTESIAN_POINT('Ctrl Pts',(0.174602686720234,-1.6581634686579,15.865116755596));
#58227=CARTESIAN_POINT('Ctrl Pts',(0.108175231053316,-1.66381823013292,
15.860264030974));
#58228=CARTESIAN_POINT('Ctrl Pts',(-0.00743803082426778,-1.66670497116444,
15.8519694479799));
#58229=CARTESIAN_POINT('Ctrl Pts',(-0.0564949334702686,-1.66576404364807,
15.8484962016657));
#58230=CARTESIAN_POINT('Ctrl Pts',(-0.13873123792393,-1.66054877147338,
15.8427630185521));
#58231=CARTESIAN_POINT('Ctrl Pts',(-0.171950692152674,-1.65743832880728,
15.840471421896));
#58232=CARTESIAN_POINT('Ctrl Pts',(-0.218626712773681,-1.65164927982663,
15.8372839430274));
#58233=CARTESIAN_POINT('Ctrl Pts',(-0.23217601851265,-1.6497991692572,15.8363625095072));
#58234=CARTESIAN_POINT('Ctrl Pts',(-0.255519316212987,-1.64631844255846,
15.8347812580321));
#58235=CARTESIAN_POINT('Ctrl Pts',(-0.265324161874314,-1.64476674082864,
15.8341189919467));
#58236=CARTESIAN_POINT('Ctrl Pts',(-0.285349607611146,-1.64141380846098,
15.8327700388727));
#58237=CARTESIAN_POINT('Ctrl Pts',(-0.295568432132762,-1.63960452528795,
15.8320836380471));
#58238=CARTESIAN_POINT('Ctrl Pts',(-0.321465166518379,-1.63476942593702,
15.8303487245423));
#58239=CARTESIAN_POINT('Ctrl Pts',(-0.337117938792999,-1.63161345102511,
15.8293043715621));
#58240=CARTESIAN_POINT('Ctrl Pts',(-0.398959644253236,-1.61821670908877,
15.8251925211805));
#58241=CARTESIAN_POINT('Ctrl Pts',(-0.444751099002573,-1.60623510291768,
15.8221802675393));
#58242=CARTESIAN_POINT('Ctrl Pts',(-0.597031061031835,-1.55937691448192,
15.8121867814665));
#58243=CARTESIAN_POINT('Ctrl Pts',(-0.700490841514293,-1.51572274581293,
15.8054559209477));
#58244=CARTESIAN_POINT('Ctrl Pts',(-0.855679547479872,-1.43093368257201,
15.7945746612931));
#58245=CARTESIAN_POINT('Ctrl Pts',(-0.910701405319029,-1.39655998232127,
15.7905353160295));
#58246=CARTESIAN_POINT('Ctrl Pts',(-0.975890149919765,-1.35034156031706,
15.7853441489989));
#58247=CARTESIAN_POINT('Ctrl Pts',(-0.988085911639198,-1.34144329224654,
15.7843543409962));
#58248=CARTESIAN_POINT('Ctrl Pts',(-1.00580367672783,-1.32814336134475,
15.78288603253));
#58249=CARTESIAN_POINT('Ctrl Pts',(-1.01142169752578,-1.32387007280344,
15.7824158897241));
#58250=CARTESIAN_POINT('Ctrl Pts',(-1.0209308402924,-1.31654118648524,15.7816119918));
#58251=CARTESIAN_POINT('Ctrl Pts',(-1.02483578152973,-1.31350374814129,
15.7812795022457));
#58252=CARTESIAN_POINT('Ctrl Pts',(-1.03369696882739,-1.30654754810783,
15.7805195201553));
#58253=CARTESIAN_POINT('Ctrl Pts',(-1.03864437624081,-1.30261804655469,
15.7800912871219));
#58254=CARTESIAN_POINT('Ctrl Pts',(-1.05222245870807,-1.29170705951089,
15.7789054396665));
#58255=CARTESIAN_POINT('Ctrl Pts',(-1.0608057052323,-1.28466745478105,15.7781439304664));
#58256=CARTESIAN_POINT('Ctrl Pts',(-1.10990894679043,-1.24356749158952,
15.7737214589439));
#58257=CARTESIAN_POINT('Ctrl Pts',(-1.14885389302696,-1.20768023382744,
15.7699523183217));
#58258=CARTESIAN_POINT('Ctrl Pts',(-1.25745139389566,-1.0975961631655,15.7588004514543));
#58259=CARTESIAN_POINT('Ctrl Pts',(-1.3221060570547,-1.01879277679609,15.7513254851513));
#58260=CARTESIAN_POINT('Ctrl Pts',(-1.41983244181991,-0.874577733071923,
15.7388398444594));
#58261=CARTESIAN_POINT('Ctrl Pts',(-1.45654070032965,-0.811974236279621,
15.7337469722107));
#58262=CARTESIAN_POINT('Ctrl Pts',(-1.49694752205679,-0.731446235566926,
15.7275986137052));
#58263=CARTESIAN_POINT('Ctrl Pts',(-1.50458792349412,-0.715598142119026,
15.7264067374085));
#58264=CARTESIAN_POINT('Ctrl Pts',(-1.51647955078934,-0.68989910249403,
15.7245022936193));
#58265=CARTESIAN_POINT('Ctrl Pts',(-1.52088898600338,-0.680123298482586,
15.7237843279372));
#58266=CARTESIAN_POINT('Ctrl Pts',(-1.52914180125275,-0.661344954599427,
15.7224172613965));
#58267=CARTESIAN_POINT('Ctrl Pts',(-1.53300081982786,-0.652349822330814,
15.7217676494886));
#58268=CARTESIAN_POINT('Ctrl Pts',(-1.54163293519527,-0.631729222264729,
15.7202900929988));
#58269=CARTESIAN_POINT('Ctrl Pts',(-1.54635425325742,-0.620082619465765,
15.719463923651));
#58270=CARTESIAN_POINT('Ctrl Pts',(-1.5586148499656,-0.588826850632073,
15.7172681394584));
#58271=CARTESIAN_POINT('Ctrl Pts',(-1.56591592464048,-0.569126252011633,
15.7159064263993));
#58272=CARTESIAN_POINT('Ctrl Pts',(-1.61263746205119,-0.435343827427019,
15.7067963386614));
#58273=CARTESIAN_POINT('Ctrl Pts',(-1.63993309944968,-0.31740685036405,
15.6994650151364));
#58274=CARTESIAN_POINT('Ctrl Pts',(-1.66211310840186,-0.131671155714307,
15.6880352115809));
#58275=CARTESIAN_POINT('Ctrl Pts',(-1.66603723902746,-0.0653905900801613,
15.6839705638318));
#58276=CARTESIAN_POINT('Ctrl Pts',(-1.66598117318228,0.0337685101358439,
15.6776947913277));
#58277=CARTESIAN_POINT('Ctrl Pts',(-1.66499240476525,0.066584818794768,
15.6755855692984));
#58278=CARTESIAN_POINT('Ctrl Pts',(-1.66245306059566,0.109092223704411,
15.6727869395628));
#58279=CARTESIAN_POINT('Ctrl Pts',(-1.6617853260804,0.118831017128423,15.672141204225));
#58280=CARTESIAN_POINT('Ctrl Pts',(-1.66057206892032,0.134506271009967,
15.6710937088581));
#58281=CARTESIAN_POINT('Ctrl Pts',(-1.66008018471304,0.140446824583748,
15.6706948466149));
#58282=CARTESIAN_POINT('Ctrl Pts',(-1.65906169397268,0.151993422414892,
15.6699156890247));
#58283=CARTESIAN_POINT('Ctrl Pts',(-1.65853853093764,0.15759962742323,15.6695355827035));
#58284=CARTESIAN_POINT('Ctrl Pts',(-1.65718333082297,0.171367175554307,
15.6685978579932));
#58285=CARTESIAN_POINT('Ctrl Pts',(-1.65631941608769,0.179525167346422,
15.6680385195485));
#58286=CARTESIAN_POINT('Ctrl Pts',(-1.65289846811972,0.209699586210951,
15.665956817768));
#58287=CARTESIAN_POINT('Ctrl Pts',(-1.6499625220703,0.231669637581411,15.6644157921083));
#58288=CARTESIAN_POINT('Ctrl Pts',(-1.62966381919829,0.363480196932044,
15.6550426844342));
#58289=CARTESIAN_POINT('Ctrl Pts',(-1.60179071974468,0.471330247254834,
15.6468596831304));
#58290=CARTESIAN_POINT('Ctrl Pts',(-1.56343131209642,0.575533259122747,
15.6388155835246));
#58291=CARTESIAN_POINT('',(-1.66599949106555,-0.00130221707574717,15.8714803633902));
#58292=CARTESIAN_POINT('Ctrl Pts',(-1.5634313003304,0.575533291085054,15.8337663187435));
#58293=CARTESIAN_POINT('Ctrl Pts',(-1.56631175684939,0.567708555399402,
15.8343230070768));
#58294=CARTESIAN_POINT('Ctrl Pts',(-1.56913348118854,0.55986216761892,15.8348777298986));
#58295=CARTESIAN_POINT('Ctrl Pts',(-1.57558654127743,0.541486014195911,
15.8361688898208));
#58296=CARTESIAN_POINT('Ctrl Pts',(-1.57917144943652,0.530940294232612,
15.8369037696465));
#58297=CARTESIAN_POINT('Ctrl Pts',(-1.58875133243229,0.501803486817436,
15.8389180224672));
#58298=CARTESIAN_POINT('Ctrl Pts',(-1.59452565195486,0.483141317813025,
15.8401901606427));
#58299=CARTESIAN_POINT('Ctrl Pts',(-1.63175448761917,0.354873772701569,
15.8488207696302));
#58300=CARTESIAN_POINT('Ctrl Pts',(-1.65221372937049,0.242388691633483,
15.8558017586991));
#58301=CARTESIAN_POINT('Ctrl Pts',(-1.66437451528092,0.0854194373601954,
15.8654154696456));
#58302=CARTESIAN_POINT('Ctrl Pts',(-1.66603456238488,0.0420425528584947,
15.8680623906035));
#58303=CARTESIAN_POINT('Ctrl Pts',(-1.6659994546692,-0.00134797697576474,
15.8707383599279));
#58304=CARTESIAN_POINT('Ctrl Pts',(-1.66599949106555,-0.00130221707574717,
15.8714803633902));
#58305=CARTESIAN_POINT('Ctrl Pts',(-1.66593272647584,-0.0867179089486909,
15.8772098489549));
#58306=CARTESIAN_POINT('Ctrl Pts',(-1.65929579363609,-0.171882669676792,
15.8829393345197));
#58307=CARTESIAN_POINT('Ctrl Pts',(-1.64621084163618,-0.256019266617736,
15.8886688200845));
#58308=CARTESIAN_POINT('Ctrl Pts',(-1.63689876093366,-0.315896198589341,
15.8927462849436));
#58309=CARTESIAN_POINT('Ctrl Pts',(-1.62429637850684,-0.375388018068356,
15.8968237498028));
#58310=CARTESIAN_POINT('Ctrl Pts',(-1.60844905090086,-0.434105575472282,
15.9009012146619));
#58311=CARTESIAN_POINT('Ctrl Pts',(-1.59243305180001,-0.493448094915775,
15.9050220781375));
#58312=CARTESIAN_POINT('Ctrl Pts',(-1.57310261600574,-0.551999238257112,
15.9091429416131));
#58313=CARTESIAN_POINT('Ctrl Pts',(-1.55055832123582,-0.609364334734442,
15.9132638050887));
#58314=CARTESIAN_POINT('Ctrl Pts',(-1.52831291162266,-0.665968902837409,
15.9173300354548));
#58315=CARTESIAN_POINT('Ctrl Pts',(-1.50293853451633,-0.721418190930063,
15.9213962658208));
#58316=CARTESIAN_POINT('Ctrl Pts',(-1.4745821190571,-0.775347389340462,
15.9254624961868));
#58317=CARTESIAN_POINT('Ctrl Pts',(-1.44624305988114,-0.829243578979172,
15.9295262377106));
#58318=CARTESIAN_POINT('Ctrl Pts',(-1.41492581902222,-0.881621071495188,
15.9335899792343));
#58319=CARTESIAN_POINT('Ctrl Pts',(-1.38082444922466,-0.932137243341034,
15.9376537207581));
#58320=CARTESIAN_POINT('Ctrl Pts',(-1.34673128484919,-0.982641260058941,
15.9417164844702));
#58321=CARTESIAN_POINT('Ctrl Pts',(-1.30985560770955,-1.03128442108076,
15.9457792481824));
#58322=CARTESIAN_POINT('Ctrl Pts',(-1.27043508636807,-1.07775261137468,
15.9498420118945));
#58323=CARTESIAN_POINT('Ctrl Pts',(-1.23003880943716,-1.12537100452913,
15.9540053390763));
#58324=CARTESIAN_POINT('Ctrl Pts',(-1.18697034611114,-1.17070485539578,
15.9581686662581));
#58325=CARTESIAN_POINT('Ctrl Pts',(-1.14152804400468,-1.21345363518795,
15.9623319934399));
#58326=CARTESIAN_POINT('Ctrl Pts',(-1.09712681346015,-1.25522305132806,
15.9663999398568));
#58327=CARTESIAN_POINT('Ctrl Pts',(-1.05045981264175,-1.29452430883724,
15.9704678862737));
#58328=CARTESIAN_POINT('Ctrl Pts',(-1.00183941646775,-1.3311174942925,15.9745358326906));
#58329=CARTESIAN_POINT('Ctrl Pts',(-0.95150902336914,-1.36899767531988,
15.9787468502548));
#58330=CARTESIAN_POINT('Ctrl Pts',(-0.899085743350763,-1.40397537655519,
15.982957867819));
#58331=CARTESIAN_POINT('Ctrl Pts',(-0.84494680935439,-1.43583456197496,
15.9871688853832));
#58332=CARTESIAN_POINT('Ctrl Pts',(-0.790807875358018,-1.46769374739474,
15.9913799029474));
#58333=CARTESIAN_POINT('Ctrl Pts',(-0.734953854409687,-1.49643420661138,
15.9955909205116));
#58334=CARTESIAN_POINT('Ctrl Pts',(-0.677785088133018,-1.52189466596888,
15.9998019380759));
#58335=CARTESIAN_POINT('Ctrl Pts',(-0.622427853944392,-1.54654834844266,
16.0038795192562));
#58336=CARTESIAN_POINT('Ctrl Pts',(-0.565609547040969,-1.56822861107888,
16.0079571004366));
#58337=CARTESIAN_POINT('Ctrl Pts',(-0.507681738310143,-1.58676250667401,
16.012034681617));
#58338=CARTESIAN_POINT('Ctrl Pts',(-0.449139249913106,-1.60549306789499,
16.0161555305524));
#58339=CARTESIAN_POINT('Ctrl Pts',(-0.389464019847529,-1.62100979897185,
16.0202763794878));
#58340=CARTESIAN_POINT('Ctrl Pts',(-0.329042167298717,-1.63318316552044,
16.0243972284233));
#58341=CARTESIAN_POINT('Ctrl Pts',(-0.269419352970688,-1.64519554751232,
16.0284635819127));
#58342=CARTESIAN_POINT('Ctrl Pts',(-0.209070060128925,-1.65395235230431,
16.0325299354022));
#58343=CARTESIAN_POINT('Ctrl Pts',(-0.148380494402508,-1.65937916971404,
16.0365962888917));
#58344=CARTESIAN_POINT('Ctrl Pts',(-0.0877280417093517,-1.66480266850298,
16.0406601557146));
#58345=CARTESIAN_POINT('Ctrl Pts',(-0.0267362375120464,-1.66690017194147,
16.0447240225375));
#58346=CARTESIAN_POINT('Ctrl Pts',(0.0342017959122454,-1.66564889372172,
16.0487878893604));
#58347=CARTESIAN_POINT('Ctrl Pts',(0.0951251962315448,-1.66439791597253,
16.0528507803234));
#58348=CARTESIAN_POINT('Ctrl Pts',(0.155994339855136,-1.65979976342375,
16.0569136712863));
#58349=CARTESIAN_POINT('Ctrl Pts',(0.216416401589541,-1.65188375532997,
16.0609765622492));
#58350=CARTESIAN_POINT('Ctrl Pts',(0.278330344666112,-1.64377229305206,
16.0651397700674));
#58351=CARTESIAN_POINT('Ctrl Pts',(0.339774271096009,-1.63217697065474,
16.0693029778856));
#58352=CARTESIAN_POINT('Ctrl Pts',(0.400333934123755,-1.61718543809577,
16.0734661857038));
#58353=CARTESIAN_POINT('Ctrl Pts',(0.459509786011684,-1.60253646770971,
16.0775342626532));
#58354=CARTESIAN_POINT('Ctrl Pts',(0.517840878854687,-1.58464508547898,
16.0816023396027));
#58355=CARTESIAN_POINT('Ctrl Pts',(0.574956209664161,-1.56364361571575,
16.0856704165521));
#58356=CARTESIAN_POINT('Ctrl Pts',(0.634074980099093,-1.54190547549784,
16.0898811898047));
#58357=CARTESIAN_POINT('Ctrl Pts',(0.691890545514775,-1.51683520244987,
16.0940919630573));
#58358=CARTESIAN_POINT('Ctrl Pts',(0.748016887330044,-1.48863250544554,
16.0983027363099));
#58359=CARTESIAN_POINT('Ctrl Pts',(0.804143229145313,-1.46042980844121,
16.1025135095624));
#58360=CARTESIAN_POINT('Ctrl Pts',(0.858579863315902,-1.42909504955832,
16.106724282815));
#58361=CARTESIAN_POINT('Ctrl Pts',(0.910974232784795,-1.39487703658859,
16.1109350560676));
#58362=CARTESIAN_POINT('Ctrl Pts',(0.961698065301025,-1.36175002739831,
16.1150115734375));
#58363=CARTESIAN_POINT('Ctrl Pts',(1.01071755477704,-1.32578403686299,16.1190880908075));
#58364=CARTESIAN_POINT('Ctrl Pts',(1.05769680373141,-1.28718043466189,16.1231646081774));
#58365=CARTESIAN_POINT('Ctrl Pts',(1.10518847802066,-1.24815576434612,16.1272855900892));
#58366=CARTESIAN_POINT('Ctrl Pts',(1.15059464303148,-1.20643580723475,16.1314065720009));
#58367=CARTESIAN_POINT('Ctrl Pts',(1.19359684687473,-1.16227473823133,16.1355275539127));
#58368=CARTESIAN_POINT('Ctrl Pts',(1.23601785510366,-1.11871052746619,16.1395928387577));
#58369=CARTESIAN_POINT('Ctrl Pts',(1.27609911298653,-1.07277115976455,16.1436581236028));
#58370=CARTESIAN_POINT('Ctrl Pts',(1.31356870759362,-1.02474057713688,16.1477234084479));
#58371=CARTESIAN_POINT('Ctrl Pts',(1.35101539321729,-0.976739360501363,
16.1517862077699));
#58372=CARTESIAN_POINT('Ctrl Pts',(1.38585326705964,-0.926649866940003,
16.1558490070918));
#58373=CARTESIAN_POINT('Ctrl Pts',(1.41785003069954,-0.874789855019663,
16.1599118064138));
#58374=CARTESIAN_POINT('Ctrl Pts',(1.44983913147913,-0.82294226298126,16.1639736327416));
#58375=CARTESIAN_POINT('Ctrl Pts',(1.47898820393723,-0.769325430017754,
16.1680354590695));
#58376=CARTESIAN_POINT('Ctrl Pts',(1.50510888446671,-0.714285129272178,
16.1720972853973));
#58377=CARTESIAN_POINT('Ctrl Pts',(1.53188816865151,-0.657857049091822,
16.1762615261191));
#58378=CARTESIAN_POINT('Ctrl Pts',(1.55548398130981,-0.599933228332241,
16.1804257668409));
#58379=CARTESIAN_POINT('Ctrl Pts',(1.57574513398437,-0.540909671502153,
16.1845900075627));
#58380=CARTESIAN_POINT('Ctrl Pts',(1.595533314666,-0.483263947895697,16.1886570391442));
#58381=CARTESIAN_POINT('Ctrl Pts',(1.61214077248512,-0.424569805596175,
16.1927240707257));
#58382=CARTESIAN_POINT('Ctrl Pts',(1.62547754535728,-0.365210555076479,
16.1967911023072));
#58383=CARTESIAN_POINT('Ctrl Pts',(1.63929247638957,-0.303723120303577,
16.2010039475992));
#58384=CARTESIAN_POINT('Ctrl Pts',(1.64959760152643,-0.241522565118642,
16.2052167928912));
#58385=CARTESIAN_POINT('Ctrl Pts',(1.65635136775985,-0.179042303716351,
16.2094296381831));
#58386=CARTESIAN_POINT('Ctrl Pts',(1.66310513399328,-0.116562042314061,
16.2136424834751));
#58387=CARTESIAN_POINT('Ctrl Pts',(1.66630758350186,-0.0538026803141964,
16.2178553287671));
#58388=CARTESIAN_POINT('Ctrl Pts',(1.66597673802543,0.00880388312825253,
16.222068174059));
#58389=CARTESIAN_POINT('Ctrl Pts',(1.66565645885457,0.0694109630445556,
16.2261464725192));
#58390=CARTESIAN_POINT('Ctrl Pts',(1.6620239421295,0.130125458370124,16.2302247709794));
#58391=CARTESIAN_POINT('Ctrl Pts',(1.65506632374988,0.190555671626562,16.2343030694396));
#58392=CARTESIAN_POINT('Ctrl Pts',(1.64803626679041,0.251615048281927,16.2384238287151));
#58393=CARTESIAN_POINT('Ctrl Pts',(1.63761138311908,0.312383661791834,16.2425445879905));
#58394=CARTESIAN_POINT('Ctrl Pts',(1.62383256576161,0.372456438220727,16.246665347266));
#58395=CARTESIAN_POINT('Ctrl Pts',(1.61023333543289,0.431746252574764,16.2507323983824));
#58396=CARTESIAN_POINT('Ctrl Pts',(1.59336719382399,0.490357746760353,16.2547994494988));
#58397=CARTESIAN_POINT('Ctrl Pts',(1.57332532432983,0.547908225729845,16.2588665006152));
#58398=CARTESIAN_POINT('Ctrl Pts',(1.553295754077,0.605423387273993,16.2629310558744));
#58399=CARTESIAN_POINT('Ctrl Pts',(1.53009448798927,0.661878342362491,16.2669956111336));
#58400=CARTESIAN_POINT('Ctrl Pts',(1.50386260427813,0.716905340650921,16.2710601663929));
#58401=CARTESIAN_POINT('Ctrl Pts',(1.47763708461695,0.77191898898055,16.2751237355608));
#58402=CARTESIAN_POINT('Ctrl Pts',(1.44838262701719,0.82550490653593,16.2791873047287));
#58403=CARTESIAN_POINT('Ctrl Pts',(1.41628767545806,0.877317058050051,16.2832508738967));
#58404=CARTESIAN_POINT('Ctrl Pts',(1.38341107148504,0.930391062015504,16.2874134087428));
#58405=CARTESIAN_POINT('Ctrl Pts',(1.34755404742959,0.981603262365005,16.291575943589));
#58406=CARTESIAN_POINT('Ctrl Pts',(1.30896677860741,1.03061242594011,16.2957384784352));
#58407=CARTESIAN_POINT('Ctrl Pts',(1.27124916413082,1.07851705339804,16.2998072008238));
#58408=CARTESIAN_POINT('Ctrl Pts',(1.23092349388916,1.12431656765481,16.3038759232124));
#58409=CARTESIAN_POINT('Ctrl Pts',(1.18826309874579,1.16772719766178,16.3079446456011));
#58410=CARTESIAN_POINT('Ctrl Pts',(1.14412727367919,1.21263920481925,16.312154086676));
#58411=CARTESIAN_POINT('Ctrl Pts',(1.09749267804143,1.25499362159577,16.316363527751));
#58412=CARTESIAN_POINT('Ctrl Pts',(1.04869975885901,1.29452107583038,16.3205729688259));
#58413=CARTESIAN_POINT('Ctrl Pts',(0.999906839676595,1.334048530065,16.3247824099008));
#58414=CARTESIAN_POINT('Ctrl Pts',(0.948956124574717,1.37074873014535,16.3289918509758));
#58415=CARTESIAN_POINT('Ctrl Pts',(0.896218999045746,1.40440290007869,16.3332012920507));
#58416=CARTESIAN_POINT('Ctrl Pts',(0.845122427522264,1.43701015130473,16.3372797852337));
#58417=CARTESIAN_POINT('Ctrl Pts',(0.792139052839318,1.46689216301999,16.3413582784166));
#58418=CARTESIAN_POINT('Ctrl Pts',(0.737591101952586,1.49382574831216,16.3454367715996));
#58419=CARTESIAN_POINT('Ctrl Pts',(0.682478187262265,1.5210382900187,16.3495575065347));
#58420=CARTESIAN_POINT('Ctrl Pts',(0.625768496803139,1.54524062067916,16.3536782414698));
#58421=CARTESIAN_POINT('Ctrl Pts',(0.567824574566224,1.5662475067877,16.3577989764049));
#58422=CARTESIAN_POINT('Ctrl Pts',(0.510632110943244,1.58698196043208,16.3618662706746));
#58423=CARTESIAN_POINT('Ctrl Pts',(0.452237732746338,1.60460317900944,16.3659335649443));
#58424=CARTESIAN_POINT('Ctrl Pts',(0.393012503723287,1.6189802876864,16.3700008592139));
#58425=CARTESIAN_POINT('Ctrl Pts',(0.333823366799519,1.63334863489394,16.3740656748577));
#58426=CARTESIAN_POINT('Ctrl Pts',(0.273804879129351,1.64447667161387,16.3781304905014));
#58427=CARTESIAN_POINT('Ctrl Pts',(0.21334259394841,1.65228355242294,16.3821953061451));
#58428=CARTESIAN_POINT('Ctrl Pts',(0.152894728844761,1.66008857131388,16.3862591523423));
#58429=CARTESIAN_POINT('Ctrl Pts',(0.0920037835339048,1.66457394125964,
16.3903229985394));
#58430=CARTESIAN_POINT('Ctrl Pts',(0.0310627416359322,1.6657103908189,16.3943868447366));
#58431=CARTESIAN_POINT('Ctrl Pts',(-0.0313546605475901,1.66687437205375,
16.3985491418454));
#58432=CARTESIAN_POINT('Ctrl Pts',(-0.0938240599465998,1.66452498517886,
16.4027114389542));
#58433=CARTESIAN_POINT('Ctrl Pts',(-0.15592320112893,1.65868741942227,16.406873736063));
#58434=CARTESIAN_POINT('Ctrl Pts',(-0.21663094967383,1.65298065009635,16.410942772791));
#58435=CARTESIAN_POINT('Ctrl Pts',(-0.276984351890128,1.64394055084883,
16.4150118095191));
#58436=CARTESIAN_POINT('Ctrl Pts',(-0.336596719878015,1.63164292912615,
16.4190808462471));
#58437=CARTESIAN_POINT('Ctrl Pts',(-0.398258518422286,1.61892252396808,
16.4232897735463));
#58438=CARTESIAN_POINT('Ctrl Pts',(-0.459126813983947,1.60271663974591,
16.4274987008455));
#58439=CARTESIAN_POINT('Ctrl Pts',(-0.518790870360076,1.58316519442256,
16.4317076281447));
#58440=CARTESIAN_POINT('Ctrl Pts',(-0.578454926736205,1.56361374909921,
16.4359165554439));
#58441=CARTESIAN_POINT('Ctrl Pts',(-0.63691421349331,1.54071702763948,16.440125482743));
#58442=CARTESIAN_POINT('Ctrl Pts',(-0.693783714101098,1.51466833268808,
16.4443344100422));
#58443=CARTESIAN_POINT('Ctrl Pts',(-0.748781390671607,1.489477014236,16.4484048031323));
#58444=CARTESIAN_POINT('Ctrl Pts',(-0.802520678716739,1.46123344702838,
16.4524751962224));
#58445=CARTESIAN_POINT('Ctrl Pts',(-0.854640355774557,1.4300859632489,16.4565455893124));
#58446=CARTESIAN_POINT('Ctrl Pts',(-0.906685706697143,1.39898289785846,
16.4606101777505));
#58447=CARTESIAN_POINT('Ctrl Pts',(-0.957115587177322,1.36498438372882,
16.4646747661886));
#58448=CARTESIAN_POINT('Ctrl Pts',(-1.00559068253998,1.32828588006829,16.4687393546267));
#58449=CARTESIAN_POINT('Ctrl Pts',(-1.05401479805827,1.291625971154,16.4727996684556));
#58450=CARTESIAN_POINT('Ctrl Pts',(-1.10048779713101,1.25227201095724,16.4768599822845));
#58451=CARTESIAN_POINT('Ctrl Pts',(-1.14469864655802,1.21046313804603,16.4809202961134));
#58452=CARTESIAN_POINT('Ctrl Pts',(-1.1911467321681,1.16653857804753,16.4851860771779));
#58453=CARTESIAN_POINT('Ctrl Pts',(-1.23509713265109,1.11990436848361,16.4894518582424));
#58454=CARTESIAN_POINT('Ctrl Pts',(-1.27622915987716,1.07088520929147,16.4937176393069));
#58455=CARTESIAN_POINT('Ctrl Pts',(-1.31535296308151,1.02425935428716,16.4977751485067));
#58456=CARTESIAN_POINT('Ctrl Pts',(-1.3519268586612,0.975476465052506,16.5018326577066));
#58457=CARTESIAN_POINT('Ctrl Pts',(-1.3857150905121,0.924851170690201,16.5058901669065));
#58458=CARTESIAN_POINT('Ctrl Pts',(-1.41950462859003,0.874223919192992,
16.5099478329665));
#58459=CARTESIAN_POINT('Ctrl Pts',(-1.45050801328961,0.821754554449825,
16.5140054990266));
#58460=CARTESIAN_POINT('Ctrl Pts',(-1.47853337019028,0.76778582510604,16.5180631650867));
#58461=CARTESIAN_POINT('Ctrl Pts',(-1.50658065762251,0.713774863903229,
16.5221240063703));
#58462=CARTESIAN_POINT('Ctrl Pts',(-1.53164504722335,0.658262660893737,
16.5261848476539));
#58463=CARTESIAN_POINT('Ctrl Pts',(-1.55358182078835,0.601614100662496,
16.5302456889375));
#58464=CARTESIAN_POINT('Ctrl Pts',(-1.55693824402091,0.592946620775924,
16.5308670155874));
#58465=CARTESIAN_POINT('Ctrl Pts',(-1.56022154251401,0.584252570950185,
16.5314883422372));
#58466=CARTESIAN_POINT('Ctrl Pts',(-1.56343130033213,0.575533291080358,
16.5321096688871));
#58467=CARTESIAN_POINT('Origin',(0.,0.,18.5459252805377));
#58468=CARTESIAN_POINT('',(-2.0563417111099,-0.00160732539486083,16.0959252805377));
#58469=CARTESIAN_POINT('Ctrl Pts',(1.25371187806425,1.63132526051507,16.5478693678287));
#58470=CARTESIAN_POINT('Ctrl Pts',(1.74340706608286,1.24971892553013,16.514083942288));
#58471=CARTESIAN_POINT('Ctrl Pts',(2.39627136046535,-0.0471270964805914,
16.4432541440835));
#58472=CARTESIAN_POINT('Ctrl Pts',(1.32795615156593,-2.03338265732308,16.335379973215));
#58473=CARTESIAN_POINT('Ctrl Pts',(-0.988023685722461,-2.21849194904435,
16.2242468552235));
#58474=CARTESIAN_POINT('Ctrl Pts',(-2.00194149072845,-0.89317243655016,
16.144428624331));
#58475=CARTESIAN_POINT('Ctrl Pts',(-2.05724731722716,-0.107036611257045,
16.1016547661024));
#58476=CARTESIAN_POINT('Ctrl Pts',(-2.0563417111099,-0.00160732539486083,
16.0959252805377));
#58477=CARTESIAN_POINT('Ctrl Pts',(-2.0563417111099,-0.00160732539486083,
16.0959252805377));
#58478=CARTESIAN_POINT('Ctrl Pts',(-2.05139206022102,0.574623497846713,
16.0646103934386));
#58479=CARTESIAN_POINT('Ctrl Pts',(-1.49844555770996,1.84084369321786,15.9962511336756));
#58480=CARTESIAN_POINT('Ctrl Pts',(0.185193239695499,2.23289701273988,15.9135635423805));
#58481=CARTESIAN_POINT('Ctrl Pts',(1.04119811057559,1.78983372418912,15.8621908381845));
#58482=CARTESIAN_POINT('Ctrl Pts',(1.25042353458576,1.62710269720817,15.8478625066523));
#58483=CARTESIAN_POINT('',(-2.05205730519564,0.00116258004336799,16.1540747194623));
#58484=CARTESIAN_POINT('Ctrl Pts',(-2.05205730519564,0.00116258004336799,
16.1540747194623));
#58485=CARTESIAN_POINT('Ctrl Pts',(-2.05343779045931,0.267183359675191,
16.1396948316641));
#58486=CARTESIAN_POINT('Ctrl Pts',(-1.8817826354213,1.21679945356641,16.0882705712019));
#58487=CARTESIAN_POINT('Ctrl Pts',(-0.543648734454531,2.30953699739386,
16.0056335460702));
#58488=CARTESIAN_POINT('Ctrl Pts',(0.794258702541205,1.97613964882179,15.9373764087368));
#58489=CARTESIAN_POINT('Ctrl Pts',(1.25299305265161,1.63043997671403,15.9061636440672));
#58490=CARTESIAN_POINT('Ctrl Pts',(1.25005477124305,1.62658000731212,16.6061086772888));
#58491=CARTESIAN_POINT('Ctrl Pts',(1.49824451632764,1.43685265743115,16.5892282942038));
#58492=CARTESIAN_POINT('Ctrl Pts',(2.15876687313033,0.660018185534583,16.535303538455));
#58493=CARTESIAN_POINT('Ctrl Pts',(2.08782894295346,-1.24095677525917,16.4443344100422));
#58494=CARTESIAN_POINT('Ctrl Pts',(0.0898693055670313,-2.42680223738284,
16.3332012920507));
#58495=CARTESIAN_POINT('Ctrl Pts',(-1.72097869929178,-1.52582752830307,
16.2364480618573));
#58496=CARTESIAN_POINT('Ctrl Pts',(-2.04988148937533,-0.418119129138231,
16.1767392043279));
#58497=CARTESIAN_POINT('Ctrl Pts',(-2.05205730519564,0.00116258004336799,
16.1540747194623));
#58498=CARTESIAN_POINT('Origin',(-4.61329551933804E-17,0.,6.));
#58499=CARTESIAN_POINT('Ctrl Pts',(-0.769902040670523,-1.47743251885539,
6.));
#58500=CARTESIAN_POINT('Ctrl Pts',(-0.717792690454589,-1.5127546675874,
6.));
#58501=CARTESIAN_POINT('Ctrl Pts',(-0.663680270308176,-1.54477770941651,
6.00000000000001));
#58502=CARTESIAN_POINT('Ctrl Pts',(-0.607902703315375,-1.57356639043324,
6.00000000000001));
#58503=CARTESIAN_POINT('Ctrl Pts',(-0.573141437544782,-1.59150785052124,
6.));
#58504=CARTESIAN_POINT('Ctrl Pts',(-0.53773253874008,-1.60819244673183,
6.00000000000001));
#58505=CARTESIAN_POINT('Ctrl Pts',(-0.501750440668204,-1.62362886153923,
6.00000000000001));
#58506=CARTESIAN_POINT('Ctrl Pts',(-0.479711493700921,-1.63308362781289,
6.00000000000001));
#58507=CARTESIAN_POINT('Ctrl Pts',(-0.457457406962398,-1.64207002758286,
6.00000000000001));
#58508=CARTESIAN_POINT('Ctrl Pts',(-0.435004451876358,-1.65058900058075,
6.00000000000001));
#58509=CARTESIAN_POINT('Ctrl Pts',(-0.418606024085174,-1.65681079913802,
6.00000000000001));
#58510=CARTESIAN_POINT('Ctrl Pts',(-0.402098744685564,-1.66278403922844,
6.00000000000001));
#58511=CARTESIAN_POINT('Ctrl Pts',(-0.385511599491679,-1.66850143620088,
6.00000000000001));
#58512=CARTESIAN_POINT('Ctrl Pts',(-0.323111145475881,-1.69001015049128,
6.00000000000001));
#58513=CARTESIAN_POINT('Ctrl Pts',(-0.259519986062337,-1.70792667113092,
6.00000000000001));
#58514=CARTESIAN_POINT('Ctrl Pts',(-0.195088121265483,-1.72229690513172,
6.00000000000002));
#58515=CARTESIAN_POINT('Ctrl Pts',(-0.148683978642291,-1.7326464176005,
6.00000000000002));
#58516=CARTESIAN_POINT('Ctrl Pts',(-0.101842867286457,-1.74115566058215,
6.00000000000001));
#58517=CARTESIAN_POINT('Ctrl Pts',(-0.054686471152061,-1.74782780182351,
6.00000000000001));
#58518=CARTESIAN_POINT('Ctrl Pts',(-0.0415571896974309,-1.74968545905442,
6.00000000000002));
#58519=CARTESIAN_POINT('Ctrl Pts',(-0.0284034339604797,-1.75140063593638,
6.00000000000001));
#58520=CARTESIAN_POINT('Ctrl Pts',(-0.0152277599227589,-1.75297323080655,
6.00000000000001));
#58521=CARTESIAN_POINT('Ctrl Pts',(-0.0022440902626824,-1.75452290881506,
6.00000000000001));
#58522=CARTESIAN_POINT('Ctrl Pts',(0.0107521937013583,-1.75593306946262,
6.00000000000001));
#58523=CARTESIAN_POINT('Ctrl Pts',(0.0237549906381194,-1.75720382375573,
6.00000000000001));
#58524=CARTESIAN_POINT('Ctrl Pts',(0.0916321708382992,-1.76383741332595,
6.00000000000001));
#58525=CARTESIAN_POINT('Ctrl Pts',(0.159714737884047,-1.76667936393847,
6.00000000000001));
#58526=CARTESIAN_POINT('Ctrl Pts',(0.227642895266991,-1.76577762622816,
6.00000000000002));
#58527=CARTESIAN_POINT('Ctrl Pts',(0.29621450048859,-1.76486734682906,6.00000000000002));
#58528=CARTESIAN_POINT('Ctrl Pts',(0.364629792877382,-1.76014241722597,
6.00000000000003));
#58529=CARTESIAN_POINT('Ctrl Pts',(0.432540137812221,-1.75160369638492,
6.00000000000002));
#58530=CARTESIAN_POINT('Ctrl Pts',(0.499749119582646,-1.74315316158202,
6.00000000000001));
#58531=CARTESIAN_POINT('Ctrl Pts',(0.566464616270658,-1.73096734546305,
6.00000000000001));
#58532=CARTESIAN_POINT('Ctrl Pts',(0.632353683799982,-1.71499680905896,
6.));
#58533=CARTESIAN_POINT('Ctrl Pts',(0.641114946675616,-1.71287320839276,
6.));
#58534=CARTESIAN_POINT('Ctrl Pts',(0.64986159083715,-1.71068261477665,6.));
#58535=CARTESIAN_POINT('Ctrl Pts',(0.658592824186962,-1.70842484195969,
6.));
#58536=CARTESIAN_POINT('Ctrl Pts',(0.673329590642755,-1.70461412365901,
6.));
#58537=CARTESIAN_POINT('Ctrl Pts',(0.688024362203397,-1.70061130221074,
6.));
#58538=CARTESIAN_POINT('Ctrl Pts',(0.702647425019036,-1.69642335099993,
6.));
#58539=CARTESIAN_POINT('Ctrl Pts',(0.7693973145121,-1.67730661163773,6.));
#58540=CARTESIAN_POINT('Ctrl Pts',(0.834774763838756,-1.65430615406101,
5.99999999999999));
#58541=CARTESIAN_POINT('Ctrl Pts',(0.898433301540374,-1.62743891355796,
5.99999999999999));
#58542=CARTESIAN_POINT('Ctrl Pts',(0.90557737680475,-1.62442373923524,5.99999999999999));
#58543=CARTESIAN_POINT('Ctrl Pts',(0.912699810919337,-1.62135981461256,
5.99999999999998));
#58544=CARTESIAN_POINT('Ctrl Pts',(0.919800118172371,-1.61824712514219,
5.99999999999999));
#58545=CARTESIAN_POINT('Ctrl Pts',(0.981482004348972,-1.591206526648,5.99999999999998));
#58546=CARTESIAN_POINT('Ctrl Pts',(1.04149484275984,-1.56049006590522,5.99999999999998));
#58547=CARTESIAN_POINT('Ctrl Pts',(1.09969687621398,-1.52640741779604,5.99999999999998));
#58548=CARTESIAN_POINT('Ctrl Pts',(1.15948995750665,-1.49139306472077,5.99999999999998));
#58549=CARTESIAN_POINT('Ctrl Pts',(1.21737260446499,-1.45282558408269,5.99999999999998));
#58550=CARTESIAN_POINT('Ctrl Pts',(1.27317445221614,-1.410988847483,5.99999999999998));
#58551=CARTESIAN_POINT('Ctrl Pts',(1.28645120926298,-1.40103476513892,5.99999999999998));
#58552=CARTESIAN_POINT('Ctrl Pts',(1.29961007313401,-1.3908954029497,5.99999999999997));
#58553=CARTESIAN_POINT('Ctrl Pts',(1.31264854265785,-1.38057420752588,5.99999999999997));
#58554=CARTESIAN_POINT('Ctrl Pts',(1.32186339391781,-1.37327977158908,5.99999999999997));
#58555=CARTESIAN_POINT('Ctrl Pts',(1.33101119979217,-1.36589995544344,5.99999999999997));
#58556=CARTESIAN_POINT('Ctrl Pts',(1.34008906352326,-1.35843826611053,5.99999999999997));
#58557=CARTESIAN_POINT('Ctrl Pts',(1.3948324733697,-1.31344108071559,5.99999999999997));
#58558=CARTESIAN_POINT('Ctrl Pts',(1.447059982822,-1.26544976553847,5.99999999999997));
#58559=CARTESIAN_POINT('Ctrl Pts',(1.49662261989952,-1.21481178342751,5.99999999999997));
#58560=CARTESIAN_POINT('Ctrl Pts',(1.5476087031021,-1.16271947112618,5.99999999999997));
#58561=CARTESIAN_POINT('Ctrl Pts',(1.59577544363691,-1.10782579891501,5.99999999999997));
#58562=CARTESIAN_POINT('Ctrl Pts',(1.6409401980567,-1.05045698070005,5.99999999999997));
#58563=CARTESIAN_POINT('Ctrl Pts',(1.68610495247649,-0.993088162485092,
5.99999999999997));
#58564=CARTESIAN_POINT('Ctrl Pts',(1.72826847776074,-0.9332434256593,5.99999999999997));
#58565=CARTESIAN_POINT('Ctrl Pts',(1.76721630323826,-0.871207567283829,
5.99999999999997));
#58566=CARTESIAN_POINT('Ctrl Pts',(1.77683707359166,-0.855883663066091,
5.99999999999997));
#58567=CARTESIAN_POINT('Ctrl Pts',(1.78626144751713,-0.840425896263523,
5.99999999999997));
#58568=CARTESIAN_POINT('Ctrl Pts',(1.79548580943118,-0.824838255363802,
5.99999999999997));
#58569=CARTESIAN_POINT('Ctrl Pts',(1.80275062876371,-0.812561916250909,
5.99999999999997));
#58570=CARTESIAN_POINT('Ctrl Pts',(1.8098921539507,-0.800203421397945,5.99999999999997));
#58571=CARTESIAN_POINT('Ctrl Pts',(1.81689809304296,-0.787783901963097,
5.99999999999998));
#58572=CARTESIAN_POINT('Ctrl Pts',(1.85392217059638,-0.722150837690512,
5.99999999999998));
#58573=CARTESIAN_POINT('Ctrl Pts',(1.8872321068448,-0.654701280967435,5.99999999999997));
#58574=CARTESIAN_POINT('Ctrl Pts',(1.91664683208078,-0.585782110438423,
5.99999999999998));
#58575=CARTESIAN_POINT('Ctrl Pts',(1.94609438539803,-0.516786023191269,
5.99999999999998));
#58576=CARTESIAN_POINT('Ctrl Pts',(1.97163879432696,-0.446316209639087,
5.99999999999998));
#58577=CARTESIAN_POINT('Ctrl Pts',(1.99306265208051,-0.37468298955617,5.99999999999999));
#58578=CARTESIAN_POINT('Ctrl Pts',(2.01399848774479,-0.304681529454561,
5.99999999999999));
#58579=CARTESIAN_POINT('Ctrl Pts',(2.03099991890157,-0.233568183954131,
5.99999999999999));
#58580=CARTESIAN_POINT('Ctrl Pts',(2.04382045531739,-0.161609345165651,
5.99999999999999));
#58581=CARTESIAN_POINT('Ctrl Pts',(2.04657337095263,-0.146157837836297,
6.));
#58582=CARTESIAN_POINT('Ctrl Pts',(2.04913333444925,-0.130667287270638,
6.));
#58583=CARTESIAN_POINT('Ctrl Pts',(2.05149759654652,-0.11514024651189,6.));
#58584=CARTESIAN_POINT('Ctrl Pts',(2.05348812665688,-0.102067650968936,
6.));
#58585=CARTESIAN_POINT('Ctrl Pts',(2.05533993402975,-0.0889691892837262,
6.));
#58586=CARTESIAN_POINT('Ctrl Pts',(2.05705381956725,-0.0758464997591838,
6.));
#58587=CARTESIAN_POINT('Ctrl Pts',(1.81742788875951,0.95862058795916,6.));
#58588=CARTESIAN_POINT('Ctrl Pts',(1.77621084984922,1.02166717021418,6.));
#58589=CARTESIAN_POINT('Ctrl Pts',(1.73133475147209,1.08211786795308,6.));
#58590=CARTESIAN_POINT('Ctrl Pts',(1.68313661090665,1.13981832064103,5.99999999999999));
#58591=CARTESIAN_POINT('Ctrl Pts',(1.63705290425077,1.19498747663728,5.99999999999999));
#58592=CARTESIAN_POINT('Ctrl Pts',(1.58793118040593,1.24764248850107,6.));
#58593=CARTESIAN_POINT('Ctrl Pts',(1.53604072926498,1.29761177692827,5.99999999999999));
#58594=CARTESIAN_POINT('Ctrl Pts',(1.5243500726217,1.30886960531223,5.99999999999999));
#58595=CARTESIAN_POINT('Ctrl Pts',(1.51251721040882,1.31999241970392,5.99999999999999));
#58596=CARTESIAN_POINT('Ctrl Pts',(1.50055023090591,1.33097329770719,5.99999999999999));
#58597=CARTESIAN_POINT('Ctrl Pts',(1.44563988718906,1.38135892637195,5.99999999999999));
#58598=CARTESIAN_POINT('Ctrl Pts',(1.38801753538455,1.42866081625881,5.99999999999999));
#58599=CARTESIAN_POINT('Ctrl Pts',(1.32799860875722,1.47270620083035,5.99999999999998));
#58600=CARTESIAN_POINT('Ctrl Pts',(1.28586226841847,1.50362830188993,5.99999999999998));
#58601=CARTESIAN_POINT('Ctrl Pts',(1.24254403319794,1.53294445717117,5.99999999999998));
#58602=CARTESIAN_POINT('Ctrl Pts',(1.19814772472919,1.56058048211627,5.99999999999998));
#58603=CARTESIAN_POINT('Ctrl Pts',(1.18126768766072,1.57108804775828,5.99999999999998));
#58604=CARTESIAN_POINT('Ctrl Pts',(1.1642317740111,1.58135260171141,5.99999999999998));
#58605=CARTESIAN_POINT('Ctrl Pts',(1.14704561463724,1.59136957843244,5.99999999999998));
#58606=CARTESIAN_POINT('Ctrl Pts',(1.12886559876529,1.60196582578565,5.99999999999998));
#58607=CARTESIAN_POINT('Ctrl Pts',(1.11051220777787,1.61228760763449,5.99999999999998));
#58608=CARTESIAN_POINT('Ctrl Pts',(1.09202852306591,1.62231025051435,5.99999999999998));
#58609=CARTESIAN_POINT('Ctrl Pts',(1.02830389374007,1.65686446480318,5.99999999999998));
#58610=CARTESIAN_POINT('Ctrl Pts',(0.96295266441871,1.68791557464673,5.99999999999997));
#58611=CARTESIAN_POINT('Ctrl Pts',(0.896264420566148,1.71530083655865,5.99999999999998));
#58612=CARTESIAN_POINT('Ctrl Pts',(0.83112333229346,1.74205076518954,5.99999999999998));
#58613=CARTESIAN_POINT('Ctrl Pts',(0.764705634417287,1.76530310424274,5.99999999999997));
#58614=CARTESIAN_POINT('Ctrl Pts',(0.697273056338519,1.78485829517618,5.99999999999998));
#58615=CARTESIAN_POINT('Ctrl Pts',(0.632855923422684,1.80353901849189,5.99999999999998));
#58616=CARTESIAN_POINT('Ctrl Pts',(0.567511973039543,1.81884577856428,5.99999999999998));
#58617=CARTESIAN_POINT('Ctrl Pts',(0.501473119004981,1.83056029517611,5.99999999999998));
#58618=CARTESIAN_POINT('Ctrl Pts',(0.479400442364202,1.83447572861231,5.99999999999998));
#58619=CARTESIAN_POINT('Ctrl Pts',(0.457250209367251,1.83798948017187,5.99999999999998));
#58620=CARTESIAN_POINT('Ctrl Pts',(0.43503136941093,1.84109224547236,5.99999999999998));
#58621=CARTESIAN_POINT('Ctrl Pts',(0.422554411239721,1.84283459894111,5.99999999999998));
#58622=CARTESIAN_POINT('Ctrl Pts',(0.410054540378993,1.84444739607236,5.99999999999998));
#58623=CARTESIAN_POINT('Ctrl Pts',(0.397551021819996,1.84592711205622,5.99999999999998));
#58624=CARTESIAN_POINT('Ctrl Pts',(0.329729122828692,1.85395342461138,5.99999999999999));
#58625=CARTESIAN_POINT('Ctrl Pts',(0.261681552305431,1.85808602681896,5.99999999999998));
#58626=CARTESIAN_POINT('Ctrl Pts',(0.193653405621123,1.8581466652395,5.99999999999998));
#58627=CARTESIAN_POINT('Ctrl Pts',(0.183851896072672,1.85815540203576,5.99999999999998));
#58628=CARTESIAN_POINT('Ctrl Pts',(0.174050795898627,1.85807952026247,5.99999999999999));
#58629=CARTESIAN_POINT('Ctrl Pts',(0.16425084754495,1.85791839663518,5.99999999999999));
#58630=CARTESIAN_POINT('Ctrl Pts',(0.094541628531198,1.8567722883275,5.99999999999999));
#58631=CARTESIAN_POINT('Ctrl Pts',(0.0248892021213018,1.85131723329971,
6.));
#58632=CARTESIAN_POINT('Ctrl Pts',(-0.0443759064452823,1.84172919357483,
6.));
#58633=CARTESIAN_POINT('Ctrl Pts',(-0.108331243473457,1.83287616028383,
6.));
#58634=CARTESIAN_POINT('Ctrl Pts',(-0.171956842007351,1.82049853882197,
6.));
#58635=CARTESIAN_POINT('Ctrl Pts',(-0.23497231125761,1.8047009628164,6.));
#58636=CARTESIAN_POINT('Ctrl Pts',(-0.248832415923801,1.80122632302535,
6.));
#58637=CARTESIAN_POINT('Ctrl Pts',(-0.262662907057445,1.79758612674387,
6.00000000000001));
#58638=CARTESIAN_POINT('Ctrl Pts',(-0.276460624295276,1.79378131032826,
6.00000000000001));
#58639=CARTESIAN_POINT('Ctrl Pts',(-0.287524089711141,1.79073048285425,
6.00000000000001));
#58640=CARTESIAN_POINT('Ctrl Pts',(-0.2985659500238,1.78757387230117,6.00000000000001));
#58641=CARTESIAN_POINT('Ctrl Pts',(-0.309571502178386,1.78431609244398,
6.00000000000001));
#58642=CARTESIAN_POINT('Ctrl Pts',(-0.375122573183307,1.7649121628876,6.00000000000001));
#58643=CARTESIAN_POINT('Ctrl Pts',(-0.4395095308677,1.74189006878232,6.00000000000002));
#58644=CARTESIAN_POINT('Ctrl Pts',(-0.502429647359492,1.71543190874701,
6.00000000000002));
#58645=CARTESIAN_POINT('Ctrl Pts',(-0.56468103391033,1.68925495232009,6.00000000000002));
#58646=CARTESIAN_POINT('Ctrl Pts',(-0.625497437618468,1.6597138520638,6.00000000000002));
#58647=CARTESIAN_POINT('Ctrl Pts',(-0.684556584297603,1.62694431289946,
6.00000000000002));
#58648=CARTESIAN_POINT('Ctrl Pts',(-0.743113515046717,1.5944534331048,6.00000000000002));
#58649=CARTESIAN_POINT('Ctrl Pts',(-0.799943720377945,1.55878814071636,
6.00000000000003));
#58650=CARTESIAN_POINT('Ctrl Pts',(-0.854692340605141,1.52005068559395,
6.00000000000003));
#58651=CARTESIAN_POINT('Ctrl Pts',(-0.866175085382049,1.51192605508031,
6.00000000000003));
#58652=CARTESIAN_POINT('Ctrl Pts',(-0.877566096038144,1.50366619624473,
6.00000000000003));
#58653=CARTESIAN_POINT('Ctrl Pts',(-0.888861820035535,1.49527192360063,
6.00000000000004));
#58654=CARTESIAN_POINT('Ctrl Pts',(-0.899513606118717,1.48735618517168,
6.00000000000004));
#58655=CARTESIAN_POINT('Ctrl Pts',(-0.91008193062578,1.47931977959631,6.00000000000003));
#58656=CARTESIAN_POINT('Ctrl Pts',(-0.920547148745782,1.4711767155375,6.00000000000004));
#58657=CARTESIAN_POINT('Ctrl Pts',(-0.972167074707126,1.43101086720119,
6.00000000000004));
#58658=CARTESIAN_POINT('Ctrl Pts',(-1.02137633331925,1.38818383327732,6.00000000000004));
#58659=CARTESIAN_POINT('Ctrl Pts',(-1.06788265822317,1.34282814309811,6.00000000000004));
#58660=CARTESIAN_POINT('Ctrl Pts',(-1.11284005981166,1.29898305359853,6.00000000000005));
#58661=CARTESIAN_POINT('Ctrl Pts',(-1.15527203055497,1.2527742460767,6.00000000000005));
#58662=CARTESIAN_POINT('Ctrl Pts',(-1.19487404980438,1.20429687549393,6.00000000000005));
#58663=CARTESIAN_POINT('Ctrl Pts',(-1.23424035546928,1.15610804511705,6.00000000000005));
#58664=CARTESIAN_POINT('Ctrl Pts',(-1.27081086720789,1.10567706111428,6.00000000000005));
#58665=CARTESIAN_POINT('Ctrl Pts',(-1.30423797357443,1.05308139435648,6.00000000000005));
#58666=CARTESIAN_POINT('Ctrl Pts',(-1.30970780350955,1.04447492542271,6.00000000000005));
#58667=CARTESIAN_POINT('Ctrl Pts',(-1.31509334809115,1.03581046919314,6.00000000000005));
#58668=CARTESIAN_POINT('Ctrl Pts',(-1.32039294356288,1.02708833860433,6.00000000000005));
#58669=CARTESIAN_POINT('Ctrl Pts',(-1.32604932595056,1.0177790043148,6.00000000000004));
#58670=CARTESIAN_POINT('Ctrl Pts',(-1.33160779623118,1.00840396758307,6.00000000000005));
#58671=CARTESIAN_POINT('Ctrl Pts',(-1.33706795287322,0.998964888140392,
6.00000000000005));
#58672=CARTESIAN_POINT('Ctrl Pts',(1.26643921716274,1.07786902174452,16.998323674252));
#58673=CARTESIAN_POINT('Ctrl Pts',(1.62497761725199,0.656628334916694,16.9612665673906));
#58674=CARTESIAN_POINT('Ctrl Pts',(1.8823477456886,-0.564254992005215,16.8871650878655));
#58675=CARTESIAN_POINT('Ctrl Pts',(0.544110383007705,-1.8901268562736,16.7760192356764));
#58676=CARTESIAN_POINT('Ctrl Pts',(-1.29159322672144,-1.4809162453331,16.6648861176848));
#58677=CARTESIAN_POINT('Ctrl Pts',(-1.94534454504545,0.281174607083069,
16.5537529996932));
#58678=CARTESIAN_POINT('Ctrl Pts',(-0.81855718778506,1.78722597471637,16.4426198817017));
#58679=CARTESIAN_POINT('Ctrl Pts',(1.05736298279991,1.65685741880359,16.3314867637101));
#58680=CARTESIAN_POINT('Ctrl Pts',(1.96556536740795,0.0104236887533924,
16.2203536457186));
#58681=CARTESIAN_POINT('Ctrl Pts',(1.07479322704078,-1.64573649927818,16.109220527727));
#58682=CARTESIAN_POINT('Ctrl Pts',(-0.799665835591146,-1.7955563655213,
15.9980874097355));
#58683=CARTESIAN_POINT('Ctrl Pts',(-1.94224246594592,-0.302063406572706,
15.8869542917439));
#58684=CARTESIAN_POINT('Ctrl Pts',(-1.30720066280732,1.46791658208971,15.7758211737524));
#58685=CARTESIAN_POINT('Ctrl Pts',(0.524241757093383,1.89438755754002,15.6646880557608));
#58686=CARTESIAN_POINT('Ctrl Pts',(1.87587794794047,0.587047795516583,15.5535549377692));
#58687=CARTESIAN_POINT('Ctrl Pts',(1.51063656570958,-1.25758504499101,15.4424218197777));
#58688=CARTESIAN_POINT('Ctrl Pts',(-0.23719873324387,-1.95122454958629,
15.3312887017861));
#58689=CARTESIAN_POINT('Ctrl Pts',(-1.76794048158266,-0.859027596207237,
15.2201555837946));
#58690=CARTESIAN_POINT('Ctrl Pts',(-1.68059348111992,1.01938577340468,15.109022465803));
#58691=CARTESIAN_POINT('Ctrl Pts',(-0.055101197330089,1.9648168731157,14.9978893478114));
#58692=CARTESIAN_POINT('Ctrl Pts',(1.62082188049643,1.11197038656462,14.8867562298199));
#58693=CARTESIAN_POINT('Ctrl Pts',(1.81330497340411,-0.758595243245752,
14.7756231118283));
#58694=CARTESIAN_POINT('Ctrl Pts',(0.346179986260669,-1.93486460720292,
14.6644899938368));
#58695=CARTESIAN_POINT('Ctrl Pts',(-1.43778255117909,-1.34026974869229,
14.5533568758452));
#58696=CARTESIAN_POINT('Ctrl Pts',(-1.90582990649864,0.48099274761629,14.4422237578536));
#58697=CARTESIAN_POINT('Ctrl Pts',(-0.629586719028806,1.86203174370634,
14.3310906398621));
#58698=CARTESIAN_POINT('Ctrl Pts',(1.22287901418285,1.53886600219443,14.2199575218705));
#58699=CARTESIAN_POINT('Ctrl Pts',(1.95611774146339,-0.192730475320511,
14.108824403879));
#58700=CARTESIAN_POINT('Ctrl Pts',(0.899040519765985,-1.74793243517711,
13.9976912858874));
#58701=CARTESIAN_POINT('Ctrl Pts',(-0.980873971539237,-1.70335783285293,
13.8865581678959));
#58702=CARTESIAN_POINT('Ctrl Pts',(-1.96305399725381,-0.0998030981586012,
13.7754250499043));
#58703=CARTESIAN_POINT('Ctrl Pts',(-1.14856973963694,1.59509536006063,13.6642919319127));
#58704=CARTESIAN_POINT('Ctrl Pts',(0.71713075096409,1.83009976247439,13.5531588139212));
#58705=CARTESIAN_POINT('Ctrl Pts',(1.92648495228938,0.390124830213576,13.4420256959296));
#58706=CARTESIAN_POINT('Ctrl Pts',(1.3726442995717,-1.40690770180496,13.330892577938));
#58707=CARTESIAN_POINT('Ctrl Pts',(-0.437494442867744,-1.91628292979319,
13.2197594599465));
#58708=CARTESIAN_POINT('Ctrl Pts',(-1.84722105158085,-0.671800596268771,
13.1086263419549));
#58709=CARTESIAN_POINT('Ctrl Pts',(-1.56629824797523,1.18754008477213,12.9974932239634));
#58710=CARTESIAN_POINT('Ctrl Pts',(0.148162361075704,1.95999733910862,12.8863601059718));
#58711=CARTESIAN_POINT('Ctrl Pts',(1.7270189456564,0.938587883948701,12.7752269879802));
#58712=CARTESIAN_POINT('Ctrl Pts',(1.72523981636906,-0.941854145059837,
12.6640938699887));
#58713=CARTESIAN_POINT('Ctrl Pts',(0.144453302363285,-1.9602741894919,12.5529607519971));
#58714=CARTESIAN_POINT('Ctrl Pts',(-1.56854255959194,-1.18457414006062,
12.4418276340056));
#58715=CARTESIAN_POINT('Ctrl Pts',(-1.84594653377508,0.675294786737895,
12.330694516014));
#58716=CARTESIAN_POINT('Ctrl Pts',(-0.433867584499705,1.91710734537012,
12.2195613980225));
#58717=CARTESIAN_POINT('Ctrl Pts',(1.37530405497152,1.40430780490978,12.1084282800309));
#58718=CARTESIAN_POINT('Ctrl Pts',(1.9257432918927,-0.393769511620569,11.9972951620393));
#58719=CARTESIAN_POINT('Ctrl Pts',(0.713666471556317,-1.83145347249883,
11.8861620440478));
#58720=CARTESIAN_POINT('Ctrl Pts',(-1.15158599318701,-1.59291913003992,
11.7750289260562));
#58721=CARTESIAN_POINT('Ctrl Pts',(-1.96286163098258,0.103517496917523,
11.6638958080646));
#58722=CARTESIAN_POINT('Ctrl Pts',(-0.977649046621936,1.70521083628707,
11.5527626900731));
#58723=CARTESIAN_POINT('Ctrl Pts',(0.902346425098597,1.7462281018422,11.4416295720815));
#58724=CARTESIAN_POINT('Ctrl Pts',(1.9564789325597,0.189028677723019,11.33049645409));
#58725=CARTESIAN_POINT('Ctrl Pts',(1.21996491468177,-1.54117723234452,11.2193633360984));
#58726=CARTESIAN_POINT('Ctrl Pts',(-0.633109010464032,-1.86083707922561,
11.1082302181069));
#58727=CARTESIAN_POINT('Ctrl Pts',(-1.90673665030534,-0.477385589365701,
10.9970971001153));
#58728=CARTESIAN_POINT('Ctrl Pts',(-1.43524385936396,1.3429879815954,10.8859639821237));
#58729=CARTESIAN_POINT('Ctrl Pts',(0.349840602315146,1.93420609230853,10.7748308641322));
#58730=CARTESIAN_POINT('Ctrl Pts',(1.8147371751635,0.755162657730938,10.6636977461406));
#58731=CARTESIAN_POINT('Ctrl Pts',(1.61871485794303,-1.11503536411457,10.5525646281491));
#58732=CARTESIAN_POINT('Ctrl Pts',(-0.0588190092628553,-1.96470913335817,
10.4414315101575));
#58733=CARTESIAN_POINT('Ctrl Pts',(-1.68251940409772,-1.01620377355444,
10.330298392166));
#58734=CARTESIAN_POINT('Ctrl Pts',(-1.76631181698397,0.862371277197082,
10.2191652741744));
#58735=CARTESIAN_POINT('Ctrl Pts',(-0.23350613361075,1.9516701924551,10.1080321561828));
#58736=CARTESIAN_POINT('Ctrl Pts',(1.51301355395472,1.25472373058804,9.99689903819129));
#58737=CARTESIAN_POINT('Ctrl Pts',(1.87476368530798,-0.590595274958111,
9.88576592019971));
#58738=CARTESIAN_POINT('Ctrl Pts',(0.520656301887133,-1.89537823925887,
9.77463280220817));
#58739=CARTESIAN_POINT('Ctrl Pts',(-1.30997622185192,-1.4654364376298,9.6634996842166));
#58740=CARTESIAN_POINT('Ctrl Pts',(-1.94166694719282,0.305730470734983,
9.55236656622504));
#58741=CARTESIAN_POINT('Ctrl Pts',(-0.796267659191974,1.79708081884754,
9.44123344823349));
#58742=CARTESIAN_POINT('Ctrl Pts',(1.07790713128235,1.6436720691419,9.33010033024192));
#58743=CARTESIAN_POINT('Ctrl Pts',(1.96553888921238,-0.0140900525500748,
9.21896721225038));
#58744=CARTESIAN_POINT('Ctrl Pts',(1.05423209284676,-1.65895640355874,9.10783409425879));
#58745=CARTESIAN_POINT('Ctrl Pts',(-0.821949409002516,-1.78548055816259,
8.99670097626726));
#58746=CARTESIAN_POINT('Ctrl Pts',(-1.94585046023486,-0.277862630068061,
8.88556785827569));
#58747=CARTESIAN_POINT('Ctrl Pts',(-1.2888325821115,1.48406611355865,8.77443474028413));
#58748=CARTESIAN_POINT('Ctrl Pts',(0.547775602694242,1.88771913792229,8.66330162229257));
#58749=CARTESIAN_POINT('Ctrl Pts',(1.88303799648319,0.563657307092937,8.55216850430101));
#58750=CARTESIAN_POINT('Ctrl Pts',(1.49486989869632,-1.27628587601649,8.44103538630945));
#58751=CARTESIAN_POINT('Ctrl Pts',(-0.261461964938926,-1.94812199224134,
8.32990226831789));
#58752=CARTESIAN_POINT('Ctrl Pts',(-1.77849355284479,-0.836960181982545,
8.21876915032633));
#58753=CARTESIAN_POINT('Ctrl Pts',(-1.66777782961535,1.04022052572397,8.10763603233478));
#58754=CARTESIAN_POINT('Ctrl Pts',(-0.0306462141602966,1.96535047235978,
7.99650291434321));
#58755=CARTESIAN_POINT('Ctrl Pts',(1.63453406194913,1.0917142983495,7.88536979635166));
#58756=CARTESIAN_POINT('Ctrl Pts',(1.80372435497444,-0.781101746316954,
7.77423667836009));
#58757=CARTESIAN_POINT('Ctrl Pts',(0.322075267633636,-1.93902277598313,
7.66310356036854));
#58758=CARTESIAN_POINT('Ctrl Pts',(-1.45435005500721,-1.32227375190043,
7.55197044237697));
#58759=CARTESIAN_POINT('Ctrl Pts',(-1.89969644190983,0.50467208220374,7.44083732438543));
#58760=CARTESIAN_POINT('Ctrl Pts',(-0.60636687257194,1.86972249141181,7.32970420639386));
#58761=CARTESIAN_POINT('Ctrl Pts',(1.24193543302636,1.52352865742128,7.2185710884023));
#58762=CARTESIAN_POINT('Ctrl Pts',(1.95356590264256,-0.217057370469622,
7.10743797041074));
#58763=CARTESIAN_POINT('Ctrl Pts',(0.877222931654791,-1.75898624013855,
6.99630485241919));
#58764=CARTESIAN_POINT('Ctrl Pts',(-1.00200230080329,-1.6910172936132,6.88517173442762));
#58765=CARTESIAN_POINT('Ctrl Pts',(-1.96413016477178,-0.075371123179428,
6.77403861643607));
#58766=CARTESIAN_POINT('Ctrl Pts',(-1.12865736944011,1.6092736399872,6.6629054984445));
#58767=CARTESIAN_POINT('Ctrl Pts',(0.739899879799323,1.82101730763706,6.55177238045295));
#58768=CARTESIAN_POINT('Ctrl Pts',(1.93109432141268,0.366152571270065,6.44063926246139));
#58769=CARTESIAN_POINT('Ctrl Pts',(1.35521404062397,-1.42394081986265,6.32950614446983));
#58770=CARTESIAN_POINT('Ctrl Pts',(-0.461659097576337,-1.91057463508532,
6.21837302647827));
#58771=CARTESIAN_POINT('Ctrl Pts',(-1.85476354891606,-0.648982408557044,
6.10723990848671));
#58772=CARTESIAN_POINT('Ctrl Pts',(-1.55270934033744,1.20736462849148,5.99610679049515));
#58773=CARTESIAN_POINT('Ctrl Pts',(0.175237007265808,1.95716707999619,5.8849736725036));
#58774=CARTESIAN_POINT('Ctrl Pts',(1.21296802187357,1.26497356239067,5.81088492717589));
#58775=CARTESIAN_POINT('Ctrl Pts',(1.47095156957581,0.775868174581949,5.77384055451203));
#58776=CARTESIAN_POINT('Ctrl Pts',(1.36652085687194,1.16304871108613,17.0742005794842));
#58777=CARTESIAN_POINT('Ctrl Pts',(1.753393116568,0.708519053039916,17.0371434726228));
#58778=CARTESIAN_POINT('Ctrl Pts',(2.03110217964673,-0.608845813300611,
16.9630419930976));
#58779=CARTESIAN_POINT('Ctrl Pts',(0.587109256207644,-2.03949604231164,
16.8518961409086));
#58780=CARTESIAN_POINT('Ctrl Pts',(-1.39366268747075,-1.5979471490641,16.740763022917));
#58781=CARTESIAN_POINT('Ctrl Pts',(-2.09907736477262,0.30339471472038,16.6296299049255));
#58782=CARTESIAN_POINT('Ctrl Pts',(-0.883244497242211,1.92846331454007,
16.5184967869339));
#58783=CARTESIAN_POINT('Ctrl Pts',(1.14092216167901,1.7877922516728,16.4073636689423));
#58784=CARTESIAN_POINT('Ctrl Pts',(2.1208961580688,0.0112474312971465,16.2962305509508));
#58785=CARTESIAN_POINT('Ctrl Pts',(1.1597298485958,-1.77579249023686,16.1850974329592));
#58786=CARTESIAN_POINT('Ctrl Pts',(-0.862860236838991,-1.93745202290173,
16.0739643149677));
#58787=CARTESIAN_POINT('Ctrl Pts',(-2.09573014073555,-0.325934272711604,
15.9628311969761));
#58788=CARTESIAN_POINT('Ctrl Pts',(-1.41050351697493,1.58392017428815,15.8516980789846));
#58789=CARTESIAN_POINT('Ctrl Pts',(0.56567049204008,2.0440934498039,15.740564960993));
#58790=CARTESIAN_POINT('Ctrl Pts',(2.02412109958957,0.633439841156638,15.6294318430014));
#58791=CARTESIAN_POINT('Ctrl Pts',(1.63001614781033,-1.35696697479136,15.5182987250099));
#58792=CARTESIAN_POINT('Ctrl Pts',(-0.255943602984384,-2.10542204261793,
15.4071656070183));
#58793=CARTESIAN_POINT('Ctrl Pts',(-1.90765376581075,-0.926913120612018,
15.2960324890267));
#58794=CARTESIAN_POINT('Ctrl Pts',(-1.81340408031464,1.0999437649103,15.1848993710352));
#58795=CARTESIAN_POINT('Ctrl Pts',(-0.0594556251652374,2.12008851325826,
15.0737662530436));
#58796=CARTESIAN_POINT('Ctrl Pts',(1.7489089685132,1.19984497074307,14.9626331350521));
#58797=CARTESIAN_POINT('Ctrl Pts',(1.95660323246916,-0.818543999404555,
14.8515000170605));
#58798=CARTESIAN_POINT('Ctrl Pts',(0.37353720971834,-2.08776923924519,14.7403668990689));
#58799=CARTESIAN_POINT('Ctrl Pts',(-1.55140477111448,-1.44618592081011,
14.6292337810774));
#58800=CARTESIAN_POINT('Ctrl Pts',(-2.05644004195902,0.519003685857384,
14.5181006630858));
#58801=CARTESIAN_POINT('Ctrl Pts',(-0.679340446113083,2.0091806850651,14.4069675450943));
#58802=CARTESIAN_POINT('Ctrl Pts',(1.31951826480522,1.66047644405789,14.2958344271027));
#58803=CARTESIAN_POINT('Ctrl Pts',(2.11070192393092,-0.207961196014097,
14.1847013091112));
#58804=CARTESIAN_POINT('Ctrl Pts',(0.97008810591447,-1.88606456330667,14.0735681911196));
#58805=CARTESIAN_POINT('Ctrl Pts',(-1.05838852896084,-1.83796740796175,
13.962435073128));
#58806=CARTESIAN_POINT('Ctrl Pts',(-2.11818632434884,-0.107690138907505,
13.8513019551365));
#58807=CARTESIAN_POINT('Ctrl Pts',(-1.23933662469974,1.72114938378634,13.7401688371449));
#58808=CARTESIAN_POINT('Ctrl Pts',(0.77380273369309,1.97472524672794,13.6290357191534));
#58809=CARTESIAN_POINT('Ctrl Pts',(2.07872737362893,0.420954839399902,13.5179026011618));
#58810=CARTESIAN_POINT('Ctrl Pts',(1.48111890330862,-1.51809000554917,13.4067694831702));
#58811=CARTESIAN_POINT('Ctrl Pts',(-0.472067883592329,-2.0677191259891,
13.2956363651787));
#58812=CARTESIAN_POINT('Ctrl Pts',(-1.9931995630184,-0.724890317686927,
13.1845032471871));
#58813=CARTESIAN_POINT('Ctrl Pts',(-1.69007655079989,1.2813866407645,13.0733701291956));
#58814=CARTESIAN_POINT('Ctrl Pts',(0.159871041475593,2.11488811070296,12.962237011204));
#58815=CARTESIAN_POINT('Ctrl Pts',(1.86349836412969,1.01276074054045,12.8511038932124));
#58816=CARTESIAN_POINT('Ctrl Pts',(1.86157863735144,-1.0162851212386,12.7399707752209));
#58817=CARTESIAN_POINT('Ctrl Pts',(0.155868870647972,-2.11518683946771,
12.6288376572293));
#58818=CARTESIAN_POINT('Ctrl Pts',(-1.69249822141149,-1.27818630927312,
12.5177045392378));
#58819=CARTESIAN_POINT('Ctrl Pts',(-1.99182432515431,0.728660640091058,
12.4065714212462));
#58820=CARTESIAN_POINT('Ctrl Pts',(-0.468154409074422,2.06860869184061,
12.2954383032546));
#58821=CARTESIAN_POINT('Ctrl Pts',(1.48398884856836,1.51528464917292,12.1843051852631));
#58822=CARTESIAN_POINT('Ctrl Pts',(2.07792710276947,-0.424887545440438,
12.0731720672715));
#58823=CARTESIAN_POINT('Ctrl Pts',(0.770064686102175,-1.97618593505588,
11.96203894928));
#58824=CARTESIAN_POINT('Ctrl Pts',(-1.24259124073652,-1.71880117498774,
11.8509058312884));
#58825=CARTESIAN_POINT('Ctrl Pts',(-2.11797875613851,0.111698071784202,
11.7397727132969));
#58826=CARTESIAN_POINT('Ctrl Pts',(-1.05490875109103,1.83996684686597,11.6286395953053));
#58827=CARTESIAN_POINT('Ctrl Pts',(0.973655263758793,1.88422554330662,11.5175064773137));
#58828=CARTESIAN_POINT('Ctrl Pts',(2.11109165851883,0.203966860118353,11.4063733593222));
#58829=CARTESIAN_POINT('Ctrl Pts',(1.31637387564445,-1.66297032150761,11.2952402413306));
#58830=CARTESIAN_POINT('Ctrl Pts',(-0.683141090190578,-2.00789161101578,
11.1841071233391));
#58831=CARTESIAN_POINT('Ctrl Pts',(-2.05741844211191,-0.515111468278627,
11.0729740053475));
#58832=CARTESIAN_POINT('Ctrl Pts',(-1.54866545661165,1.44911896481696,10.961840887356));
#58833=CARTESIAN_POINT('Ctrl Pts',(0.377487109657989,2.08705868454541,10.8507077693644));
#58834=CARTESIAN_POINT('Ctrl Pts',(1.95814861542077,0.814840150348541,10.7395746513728));
#58835=CARTESIAN_POINT('Ctrl Pts',(1.746635436372,-1.20315216124309,10.6284415333813));
#58836=CARTESIAN_POINT('Ctrl Pts',(-0.0634672409452934,-2.11997225925744,
10.5173084153897));
#58837=CARTESIAN_POINT('Ctrl Pts',(-1.81548220130316,-1.09651030430438,
10.4061752973981));
#58838=CARTESIAN_POINT('Ctrl Pts',(-1.90589639434532,0.930521039373084,
10.2950421794066));
#58839=CARTESIAN_POINT('Ctrl Pts',(-0.251959191931444,2.10590290286506,
10.183909061415));
#58840=CARTESIAN_POINT('Ctrl Pts',(1.63258097995506,1.35387954212443,10.0727759434235));
#58841=CARTESIAN_POINT('Ctrl Pts',(2.02291878122584,-0.637267663748103,
9.96164282543193));
#58842=CARTESIAN_POINT('Ctrl Pts',(0.561801692610688,-2.04516242114731,
9.85050970744037));
#58843=CARTESIAN_POINT('Ctrl Pts',(-1.41349841737958,-1.58124403390446,
9.73937658944881));
#58844=CARTESIAN_POINT('Ctrl Pts',(-2.09510914103105,0.329891130327294,
9.62824347145725));
#58845=CARTESIAN_POINT('Ctrl Pts',(-0.859193516113775,1.93909694769355,
9.5171103534657));
#58846=CARTESIAN_POINT('Ctrl Pts',(1.16308983226872,1.7735649164216,9.40597723547412));
#58847=CARTESIAN_POINT('Ctrl Pts',(2.12086758740706,-0.0152035332001427,
9.29484411748258));
#58848=CARTESIAN_POINT('Ctrl Pts',(1.13754384998149,-1.79005711082064,9.18371099949101));
#58849=CARTESIAN_POINT('Ctrl Pts',(-0.886904792171455,-1.92657996467825,
9.07257788149945));
#58850=CARTESIAN_POINT('Ctrl Pts',(-2.09962326042144,-0.29982100537282,
8.9614447635079));
#58851=CARTESIAN_POINT('Ctrl Pts',(-1.39068388012905,1.6013459388112,8.85031164551634));
#58852=CARTESIAN_POINT('Ctrl Pts',(0.591064123586032,2.03689805158304,8.73917852752478));
#58853=CARTESIAN_POINT('Ctrl Pts',(2.03184697820833,0.608200895733785,8.62804540953321));
#58854=CARTESIAN_POINT('Ctrl Pts',(1.61300350399372,-1.37714565789816,8.51691229154166));
#58855=CARTESIAN_POINT('Ctrl Pts',(-0.282124261098154,-2.1020743025416,
8.40577917355011));
#58856=CARTESIAN_POINT('Ctrl Pts',(-1.91904080420022,-0.90310180666453,
8.29464605555853));
#58857=CARTESIAN_POINT('Ctrl Pts',(-1.79957565899125,1.12242500459889,8.183512937567));
#58858=CARTESIAN_POINT('Ctrl Pts',(-0.0330680622225432,2.12066428072216,
8.07237981957541));
#58859=CARTESIAN_POINT('Ctrl Pts',(1.76370476897043,1.1779881246746,7.96124670158388));
#58860=CARTESIAN_POINT('Ctrl Pts',(1.94626549598055,-0.842829101638638,
7.85011358359229));
#58861=CARTESIAN_POINT('Ctrl Pts',(0.347527591328071,-2.09225601151783,
7.73898046560075));
#58862=CARTESIAN_POINT('Ctrl Pts',(-1.56928153868503,-1.42676777217493,
7.62784734760918));
#58863=CARTESIAN_POINT('Ctrl Pts',(-2.04982187412916,0.544554303804206,
7.51671422961763));
#58864=CARTESIAN_POINT('Ctrl Pts',(-0.65428562781098,2.01747920188457,7.40558111162607));
#58865=CARTESIAN_POINT('Ctrl Pts',(1.34008063641694,1.64392705010552,7.29444799363451));
#58866=CARTESIAN_POINT('Ctrl Pts',(2.10794842346695,-0.234210548650754,
7.18331487564295));
#58867=CARTESIAN_POINT('Ctrl Pts',(0.946546360841719,-1.89799190638236,
7.07218175765139));
#58868=CARTESIAN_POINT('Ctrl Pts',(-1.0811865458091,-1.82465164513035,6.96104863965984));
#58869=CARTESIAN_POINT('Ctrl Pts',(-2.11934753709309,-0.0813274024009634,
6.84991552166827));
#58870=CARTESIAN_POINT('Ctrl Pts',(-1.21785065931351,1.73644811662063,6.73878240367672));
#58871=CARTESIAN_POINT('Ctrl Pts',(0.798371215957767,1.96492504171328,6.62764928568515));
#58872=CARTESIAN_POINT('Ctrl Pts',(2.08370100280802,0.395088148453585,6.5165161676936));
#58873=CARTESIAN_POINT('Ctrl Pts',(1.46231120052276,-1.53646918298456,6.40538304970203));
#58874=CARTESIAN_POINT('Ctrl Pts',(-0.498142174573606,-2.06155972751995,
6.29424993171048));
#58875=CARTESIAN_POINT('Ctrl Pts',(-2.00133811383221,-0.700268899618438,
6.18311681371891));
#58876=CARTESIAN_POINT('Ctrl Pts',(-1.67541376599547,1.30277783909705,6.07198369572737));
#58877=CARTESIAN_POINT('Ctrl Pts',(0.189085288957672,2.11183418750232,5.9608505777358));
#58878=CARTESIAN_POINT('Ctrl Pts',(1.3088240463071,1.3649393772495,5.88676183240809));
#58879=CARTESIAN_POINT('Ctrl Pts',(1.5871950047292,0.837181941605297,5.84971745974424));
#58880=CARTESIAN_POINT('Ctrl Pts',(1.46660249658114,1.24822840042773,17.1500774847164));
#58881=CARTESIAN_POINT('Ctrl Pts',(1.88180861588401,0.760409771163138,17.113020377855));
#58882=CARTESIAN_POINT('Ctrl Pts',(2.17985661360488,-0.653436634596006,
17.0389188983298));
#58883=CARTESIAN_POINT('Ctrl Pts',(0.630108129407586,-2.18886522834968,
16.9277730461408));
#58884=CARTESIAN_POINT('Ctrl Pts',(-1.49573214822006,-1.71497805279509,
16.8166399281492));
#58885=CARTESIAN_POINT('Ctrl Pts',(-2.2528101844998,0.325614822357685,16.7055068101576));
#58886=CARTESIAN_POINT('Ctrl Pts',(-0.947931806699366,2.06970065436379,
16.5943736921661));
#58887=CARTESIAN_POINT('Ctrl Pts',(1.22448134055812,1.91872708454201,16.4832405741745));
#58888=CARTESIAN_POINT('Ctrl Pts',(2.27622694872966,0.0120711738409036,
16.372107456183));
#58889=CARTESIAN_POINT('Ctrl Pts',(1.24466647015081,-1.90584848119554,16.2609743381914));
#58890=CARTESIAN_POINT('Ctrl Pts',(-0.926054638086837,-2.07934768028216,
16.1498412201999));
#58891=CARTESIAN_POINT('Ctrl Pts',(-2.24921781552518,-0.349805138850504,
16.0387081022083));
#58892=CARTESIAN_POINT('Ctrl Pts',(-1.51380637114255,1.6999237664866,15.9275749842167));
#58893=CARTESIAN_POINT('Ctrl Pts',(0.607099226986776,2.19379934206778,15.8164418662252));
#58894=CARTESIAN_POINT('Ctrl Pts',(2.17236425123866,0.679831886796696,15.7053087482336));
#58895=CARTESIAN_POINT('Ctrl Pts',(1.74939572991108,-1.45634890459171,15.5941756302421));
#58896=CARTESIAN_POINT('Ctrl Pts',(-0.274688472724895,-2.25961953564957,
15.4830425122505));
#58897=CARTESIAN_POINT('Ctrl Pts',(-2.04736705003885,-0.994798645016798,
15.3719093942589));
#58898=CARTESIAN_POINT('Ctrl Pts',(-1.94621467950935,1.18050175641591,15.2607762762674));
#58899=CARTESIAN_POINT('Ctrl Pts',(-0.063810053000384,2.27536015340083,
15.1496431582758));
#58900=CARTESIAN_POINT('Ctrl Pts',(1.87699605653,1.28771955492152,15.0385100402842));
#58901=CARTESIAN_POINT('Ctrl Pts',(2.09990149153423,-0.878492755563357,
14.9273769222927));
#58902=CARTESIAN_POINT('Ctrl Pts',(0.400894433176008,-2.24067387128746,
14.8162438043011));
#58903=CARTESIAN_POINT('Ctrl Pts',(-1.66502699104989,-1.55210209292793,
14.7051106863096));
#58904=CARTESIAN_POINT('Ctrl Pts',(-2.2070501774194,0.557014624098477,14.593977568318));
#58905=CARTESIAN_POINT('Ctrl Pts',(-0.729094173197359,2.15632962642386,
14.4828444503265));
#58906=CARTESIAN_POINT('Ctrl Pts',(1.4161575154276,1.78208688592133,14.3717113323349));
#58907=CARTESIAN_POINT('Ctrl Pts',(2.26528610639844,-0.223191916707685,
14.2605782143433));
#58908=CARTESIAN_POINT('Ctrl Pts',(1.04113569206295,-2.02419669143622,14.1494450963518));
#58909=CARTESIAN_POINT('Ctrl Pts',(-1.13590308638243,-1.97257698307058,
14.0383119783602));
#58910=CARTESIAN_POINT('Ctrl Pts',(-2.27331865144387,-0.115577179656406,
13.9271788603687));
#58911=CARTESIAN_POINT('Ctrl Pts',(-1.33010350976255,1.84720340751205,13.8160457423771));
#58912=CARTESIAN_POINT('Ctrl Pts',(0.830474716422089,2.11935073098151,13.7049126243855));
#58913=CARTESIAN_POINT('Ctrl Pts',(2.23096979496849,0.451784848586225,13.593779506394));
#58914=CARTESIAN_POINT('Ctrl Pts',(1.58959350704553,-1.62927230929336,13.4826463884024));
#58915=CARTESIAN_POINT('Ctrl Pts',(-0.506641324316914,-2.21915532218502,
13.3715132704109));
#58916=CARTESIAN_POINT('Ctrl Pts',(-2.13917807445597,-0.777980039105083,
13.2603801524193));
#58917=CARTESIAN_POINT('Ctrl Pts',(-1.81385485362456,1.37523319675687,13.1492470344277));
#58918=CARTESIAN_POINT('Ctrl Pts',(0.17157972187548,2.2697788822973,13.0381139164362));
#58919=CARTESIAN_POINT('Ctrl Pts',(1.99997778260299,1.08693359713219,12.9269807984446));
#58920=CARTESIAN_POINT('Ctrl Pts',(1.99791745833382,-1.09071609741737,12.8158476804531));
#58921=CARTESIAN_POINT('Ctrl Pts',(0.167284438932658,-2.27009948944352,
12.7047145624615));
#58922=CARTESIAN_POINT('Ctrl Pts',(-1.81645388323103,-1.37179847848562,
12.59358144447));
#58923=CARTESIAN_POINT('Ctrl Pts',(-2.13770211653352,0.782026493444224,
12.4824483264784));
#58924=CARTESIAN_POINT('Ctrl Pts',(-0.50244123364914,2.2201100383111,12.3713152084868));
#58925=CARTESIAN_POINT('Ctrl Pts',(1.59267364216519,1.62626149343605,12.2601820904953));
#58926=CARTESIAN_POINT('Ctrl Pts',(2.23011091364624,-0.456005579260306,
12.1490489725037));
#58927=CARTESIAN_POINT('Ctrl Pts',(0.826462900648038,-2.12091839761294,
12.0379158545121));
#58928=CARTESIAN_POINT('Ctrl Pts',(-1.33359648828603,-1.84468321993554,
11.9267827365206));
#58929=CARTESIAN_POINT('Ctrl Pts',(-2.27309588129444,0.119878646650881,
11.815649618529));
#58930=CARTESIAN_POINT('Ctrl Pts',(-1.13216845556012,1.97472285744486,11.7045165005375));
#58931=CARTESIAN_POINT('Ctrl Pts',(1.04496410241899,2.02222298477103,11.5933833825459));
#58932=CARTESIAN_POINT('Ctrl Pts',(2.26570438447796,0.218905042513688,11.4822502645544));
#58933=CARTESIAN_POINT('Ctrl Pts',(1.41278283660713,-1.78476341067069,11.3711171465628));
#58934=CARTESIAN_POINT('Ctrl Pts',(-0.733173169917125,-2.15494614280595,
11.2599840285712));
#58935=CARTESIAN_POINT('Ctrl Pts',(-2.20810023391847,-0.552837347191554,
11.1488509105797));
#58936=CARTESIAN_POINT('Ctrl Pts',(-1.66208705385933,1.55524994803851,11.0377177925881));
#58937=CARTESIAN_POINT('Ctrl Pts',(0.405133617000831,2.23991127678228,10.9265846745966));
#58938=CARTESIAN_POINT('Ctrl Pts',(2.10156005567805,0.874517642966142,10.815451556605));
#58939=CARTESIAN_POINT('Ctrl Pts',(1.87455601480096,-1.29126895837161,10.7043184386134));
#58940=CARTESIAN_POINT('Ctrl Pts',(-0.0681154726277299,-2.27523538515673,
10.5931853206219));
#58941=CARTESIAN_POINT('Ctrl Pts',(-1.94844499850862,-1.17681683505431,
10.4820522026303));
#58942=CARTESIAN_POINT('Ctrl Pts',(-2.04548097170666,0.998670801549088,
10.3709190846388));
#58943=CARTESIAN_POINT('Ctrl Pts',(-0.270412250252138,2.26013561327502,
10.2597859666472));
#58944=CARTESIAN_POINT('Ctrl Pts',(1.75214840595539,1.45303535366084,10.1486528486557));
#58945=CARTESIAN_POINT('Ctrl Pts',(2.17107387714371,-0.683940052538099,
10.0375197306641));
#58946=CARTESIAN_POINT('Ctrl Pts',(0.602947083334242,-2.19494660303576,
9.92638661267257));
#58947=CARTESIAN_POINT('Ctrl Pts',(-1.51702061290722,-1.69705163017914,
9.81525349468102));
#58948=CARTESIAN_POINT('Ctrl Pts',(-2.24855133486928,0.354051789919607,
9.70412037668947));
#58949=CARTESIAN_POINT('Ctrl Pts',(-0.922119373035574,2.08111307653956,
9.5929872586979));
#58950=CARTESIAN_POINT('Ctrl Pts',(1.24827253325508,1.90345776370129,9.48185414070634));
#58951=CARTESIAN_POINT('Ctrl Pts',(2.27619628560175,-0.0163170138502123,
9.37072102271479));
#58952=CARTESIAN_POINT('Ctrl Pts',(1.22085560711622,-1.92115781808254,9.25958790472321));
#58953=CARTESIAN_POINT('Ctrl Pts',(-0.951860175340397,-2.06767937119391,
9.14845478673168));
#58954=CARTESIAN_POINT('Ctrl Pts',(-2.25339606060801,-0.321779380677577,
9.03732166874011));
#58955=CARTESIAN_POINT('Ctrl Pts',(-1.49253517814661,1.71862576406373,8.92618855074854));
#58956=CARTESIAN_POINT('Ctrl Pts',(0.634352644477827,2.18607696524379,8.815055432757));
#58957=CARTESIAN_POINT('Ctrl Pts',(2.18065595993346,0.652744484374632,8.70392231476542));
#58958=CARTESIAN_POINT('Ctrl Pts',(1.73113710929113,-1.47800543977982,8.59278919677388));
#58959=CARTESIAN_POINT('Ctrl Pts',(-0.302786557257382,-2.25602661284187,
8.48165607878231));
#58960=CARTESIAN_POINT('Ctrl Pts',(-2.05958805555566,-0.969243431346512,
8.37052296079076));
#58961=CARTESIAN_POINT('Ctrl Pts',(-1.93137348836714,1.20462948347381,8.25938984279919));
#58962=CARTESIAN_POINT('Ctrl Pts',(-0.0354899102847957,2.27597808908455,
8.14825672480764));
#58963=CARTESIAN_POINT('Ctrl Pts',(1.89287547599173,1.2642619509997,8.03712360681607));
#58964=CARTESIAN_POINT('Ctrl Pts',(2.08880663698666,-0.904556456960322,
7.92599048882451));
#58965=CARTESIAN_POINT('Ctrl Pts',(0.372979915022507,-2.24548924705253,
7.81485737083296));
#58966=CARTESIAN_POINT('Ctrl Pts',(-1.68421302236285,-1.53126179244943,
7.70372425284139));
#58967=CARTESIAN_POINT('Ctrl Pts',(-2.1999473063485,0.584436525404674,7.59259113484984));
#58968=CARTESIAN_POINT('Ctrl Pts',(-0.702204383050016,2.16523591235734,
7.48145801685828));
#58969=CARTESIAN_POINT('Ctrl Pts',(1.43822583980751,1.76432544278975,7.37032489886673));
#58970=CARTESIAN_POINT('Ctrl Pts',(2.26233094429135,-0.251363726831888,
7.25919178087516));
#58971=CARTESIAN_POINT('Ctrl Pts',(1.01586979002864,-2.03699757262616,7.1480586628836));
#58972=CARTESIAN_POINT('Ctrl Pts',(-1.16037079081492,-1.95828599664749,
7.03692554489204));
#58973=CARTESIAN_POINT('Ctrl Pts',(-2.2745649094144,-0.0872836816224959,
6.92579242690049));
#58974=CARTESIAN_POINT('Ctrl Pts',(-1.30704394918692,1.86362259325405,6.81465930890892));
#58975=CARTESIAN_POINT('Ctrl Pts',(0.85684255211621,2.10883277578949,6.70352619091737));
#58976=CARTESIAN_POINT('Ctrl Pts',(2.23630768420334,0.424023725637105,6.59239307292581));
#58977=CARTESIAN_POINT('Ctrl Pts',(1.56940836042156,-1.64899754610648,6.48125995493424));
#58978=CARTESIAN_POINT('Ctrl Pts',(-0.534625251570878,-2.21254481995457,
6.37012683694269));
#58979=CARTESIAN_POINT('Ctrl Pts',(-2.14791267874834,-0.751555390679831,
6.25899371895112));
#58980=CARTESIAN_POINT('Ctrl Pts',(-1.79811819165351,1.39819104970264,6.14786060095958));
#58981=CARTESIAN_POINT('Ctrl Pts',(0.202933570649542,2.26650129500845,6.03672748296801));
#58982=CARTESIAN_POINT('Ctrl Pts',(1.40468007074062,1.46490519210833,5.9626387376403));
#58983=CARTESIAN_POINT('Ctrl Pts',(1.7034384398826,0.898495708628642,5.92559436497645));
#58984=CARTESIAN_POINT('Ctrl Pts',(1.56668413629034,1.33340808976933,17.2259543899486));
#58985=CARTESIAN_POINT('Ctrl Pts',(2.01022411520002,0.81230048928636,17.1888972830873));
#58986=CARTESIAN_POINT('Ctrl Pts',(2.32861104756301,-0.698027455891402,
17.1147958035621));
#58987=CARTESIAN_POINT('Ctrl Pts',(0.673107002607527,-2.33823441438773,
17.003649951373));
#58988=CARTESIAN_POINT('Ctrl Pts',(-1.59780160896937,-1.83200895652609,
16.8925168333815));
#58989=CARTESIAN_POINT('Ctrl Pts',(-2.40654300422696,0.347834929994993,
16.7813837153899));
#58990=CARTESIAN_POINT('Ctrl Pts',(-1.01261911615652,2.2109379941875,16.6702505973984));
#58991=CARTESIAN_POINT('Ctrl Pts',(1.30804051943724,2.04966191741122,16.5591174794068));
#58992=CARTESIAN_POINT('Ctrl Pts',(2.43155773939052,0.0128949163846598,
16.4479843614153));
#58993=CARTESIAN_POINT('Ctrl Pts',(1.32960309170584,-2.03590447215423,16.3368512434237));
#58994=CARTESIAN_POINT('Ctrl Pts',(-0.989249039334683,-2.22124333766259,
16.2257181254322));
#58995=CARTESIAN_POINT('Ctrl Pts',(-2.40270549031482,-0.373676004989402,
16.1145850074406));
#58996=CARTESIAN_POINT('Ctrl Pts',(-1.61710922531016,1.81592735868504,16.003451889449));
#58997=CARTESIAN_POINT('Ctrl Pts',(0.648527961933474,2.34350523433166,15.8923187714575));
#58998=CARTESIAN_POINT('Ctrl Pts',(2.32060740288776,0.726223932436752,15.7811856534659));
#58999=CARTESIAN_POINT('Ctrl Pts',(1.86877531201183,-1.55573083439205,15.6700525354744));
#59000=CARTESIAN_POINT('Ctrl Pts',(-0.293433342465408,-2.4138170286812,
15.5589194174828));
#59001=CARTESIAN_POINT('Ctrl Pts',(-2.18708033426694,-1.06268416942158,
15.4477862994912));
#59002=CARTESIAN_POINT('Ctrl Pts',(-2.07902527870407,1.26105974792152,15.3366531814997));
#59003=CARTESIAN_POINT('Ctrl Pts',(-0.0681644808355317,2.43063179354339,
15.2255200635081));
#59004=CARTESIAN_POINT('Ctrl Pts',(2.00508314454678,1.37559413909997,15.1143869455165));
#59005=CARTESIAN_POINT('Ctrl Pts',(2.24319975059928,-0.938441511722162,
15.003253827525));
#59006=CARTESIAN_POINT('Ctrl Pts',(0.42825165663368,-2.39357850332972,14.8921207095334));
#59007=CARTESIAN_POINT('Ctrl Pts',(-1.77864921098529,-1.65801826504575,
14.7809875915419));
#59008=CARTESIAN_POINT('Ctrl Pts',(-2.35766031287977,0.595025562339573,
14.6698544735503));
#59009=CARTESIAN_POINT('Ctrl Pts',(-0.778847900281635,2.30347856778261,
14.5587213555588));
#59010=CARTESIAN_POINT('Ctrl Pts',(1.51279676604996,1.90369732778478,14.4475882375672));
#59011=CARTESIAN_POINT('Ctrl Pts',(2.41987028886597,-0.238422637401272,
14.3364551195756));
#59012=CARTESIAN_POINT('Ctrl Pts',(1.11218327821145,-2.16232881956578,14.2253220015841));
#59013=CARTESIAN_POINT('Ctrl Pts',(-1.21341764380403,-2.10718655817941,
14.1141888835925));
#59014=CARTESIAN_POINT('Ctrl Pts',(-2.42845097853889,-0.123464220405309,
14.003055765601));
#59015=CARTESIAN_POINT('Ctrl Pts',(-1.42087039482534,1.97325743123777,13.8919226476094));
#59016=CARTESIAN_POINT('Ctrl Pts',(0.887146699151091,2.26397621523506,13.7807895296178));
#59017=CARTESIAN_POINT('Ctrl Pts',(2.38321221630804,0.482614857772549,13.6696564116263));
#59018=CARTESIAN_POINT('Ctrl Pts',(1.69806811078246,-1.74045461303755,13.5585232936347));
#59019=CARTESIAN_POINT('Ctrl Pts',(-0.541214765041502,-2.37059151838093,
13.4473901756432));
#59020=CARTESIAN_POINT('Ctrl Pts',(-2.28515658589353,-0.831069760523239,
13.3362570576516));
#59021=CARTESIAN_POINT('Ctrl Pts',(-1.93763315644923,1.46907975274924,13.22512393966));
#59022=CARTESIAN_POINT('Ctrl Pts',(0.183288402275368,2.42466965389163,13.1139908216685));
#59023=CARTESIAN_POINT('Ctrl Pts',(2.13645720107629,1.16110645372394,13.0028577036769));
#59024=CARTESIAN_POINT('Ctrl Pts',(2.1342562793162,-1.16514707359613,12.8917245856853));
#59025=CARTESIAN_POINT('Ctrl Pts',(0.178700007217345,-2.42501213941933,
12.7805914676938));
#59026=CARTESIAN_POINT('Ctrl Pts',(-1.94040954505056,-1.46541064769812,
12.6694583497022));
#59027=CARTESIAN_POINT('Ctrl Pts',(-2.28357990791274,0.835392346797389,
12.5583252317107));
#59028=CARTESIAN_POINT('Ctrl Pts',(-0.536728058223856,2.3716113847816,12.4471921137191));
#59029=CARTESIAN_POINT('Ctrl Pts',(1.70135843576202,1.7372383376992,12.3360589957276));
#59030=CARTESIAN_POINT('Ctrl Pts',(2.38229472452301,-0.487123613080176,
12.224925877736));
#59031=CARTESIAN_POINT('Ctrl Pts',(0.882861115193896,-2.26565086016999,
12.1137927597444));
#59032=CARTESIAN_POINT('Ctrl Pts',(-1.42460173583554,-1.97056526488335,
12.0026596417529));
#59033=CARTESIAN_POINT('Ctrl Pts',(-2.42821300645037,0.128059221517559,
11.8915265237613));
#59034=CARTESIAN_POINT('Ctrl Pts',(-1.20942816002921,2.10947886802376,11.7803934057698));
#59035=CARTESIAN_POINT('Ctrl Pts',(1.11627294107919,2.16022042623544,11.6692602877782));
#59036=CARTESIAN_POINT('Ctrl Pts',(2.4203171104371,0.233843224909024,11.5581271697867));
#59037=CARTESIAN_POINT('Ctrl Pts',(1.50919179756981,-1.90655649983379,11.4469940517951));
#59038=CARTESIAN_POINT('Ctrl Pts',(-0.783205249643668,-2.30200067459613,
11.3358609338036));
#59039=CARTESIAN_POINT('Ctrl Pts',(-2.35878202572504,-0.590563226104481,
11.224727815812));
#59040=CARTESIAN_POINT('Ctrl Pts',(-1.77550865110702,1.66138093126007,11.1135946978204));
#59041=CARTESIAN_POINT('Ctrl Pts',(0.432780124343675,2.39276386901915,11.0024615798289));
#59042=CARTESIAN_POINT('Ctrl Pts',(2.24497149593532,0.934195135583745,10.8913284618373));
#59043=CARTESIAN_POINT('Ctrl Pts',(2.00247659322994,-1.37938575550013,10.7801953438457));
#59044=CARTESIAN_POINT('Ctrl Pts',(-0.0727637043101689,-2.43049851105601,
10.6690622258542));
#59045=CARTESIAN_POINT('Ctrl Pts',(-2.08140779571408,-1.25712336580426,
10.5579291078626));
#59046=CARTESIAN_POINT('Ctrl Pts',(-2.18506554906801,1.06682056372509,10.4467959898711));
#59047=CARTESIAN_POINT('Ctrl Pts',(-0.288865308572835,2.41436832368498,
10.3356628718795));
#59048=CARTESIAN_POINT('Ctrl Pts',(1.87171583195574,1.55219116519724,10.2245297538879));
#59049=CARTESIAN_POINT('Ctrl Pts',(2.31922897306156,-0.730612441328091,
10.1133966358964));
#59050=CARTESIAN_POINT('Ctrl Pts',(0.644092474057795,-2.3447307849242,10.0022635179048));
#59051=CARTESIAN_POINT('Ctrl Pts',(-1.62054280843487,-1.81285922645382,
9.89113039991323));
#59052=CARTESIAN_POINT('Ctrl Pts',(-2.4019935287075,0.378212449511917,9.77999728192169));
#59053=CARTESIAN_POINT('Ctrl Pts',(-0.985045229957374,2.22312920538556,
9.66886416393011));
#59054=CARTESIAN_POINT('Ctrl Pts',(1.33345523424144,2.03335061098098,9.55773104593856));
#59055=CARTESIAN_POINT('Ctrl Pts',(2.43152498379642,-0.0174304945002811,
9.44659792794699));
#59056=CARTESIAN_POINT('Ctrl Pts',(1.30416736425096,-2.05225852534442,9.33546480995544));
#59057=CARTESIAN_POINT('Ctrl Pts',(-1.01681555850934,-2.20877877770956,
9.22433169196388));
#59058=CARTESIAN_POINT('Ctrl Pts',(-2.40716886079459,-0.343737755982333,
9.11319857397231));
#59059=CARTESIAN_POINT('Ctrl Pts',(-1.59438647616416,1.83590558931627,9.00206545598079));
#59060=CARTESIAN_POINT('Ctrl Pts',(0.67764116536962,2.33525587890453,8.89093233798919));
#59061=CARTESIAN_POINT('Ctrl Pts',(2.32946494165861,0.697288073015479,8.77979921999766));
#59062=CARTESIAN_POINT('Ctrl Pts',(1.84927071458852,-1.57886522166149,8.66866610200607));
#59063=CARTESIAN_POINT('Ctrl Pts',(-0.323448853416607,-2.40997892314214,
8.55753298401454));
#59064=CARTESIAN_POINT('Ctrl Pts',(-2.2001353069111,-1.0353850560285,8.44639986602296));
#59065=CARTESIAN_POINT('Ctrl Pts',(-2.06317131774303,1.28683396234873,8.33526674803142));
#59066=CARTESIAN_POINT('Ctrl Pts',(-0.0379117583470447,2.43129189744692,
8.22413363003985));
#59067=CARTESIAN_POINT('Ctrl Pts',(2.02204618301303,1.3505357773248,8.1130005120483));
#59068=CARTESIAN_POINT('Ctrl Pts',(2.23134777799278,-0.966283812282007,
8.00186739405672));
#59069=CARTESIAN_POINT('Ctrl Pts',(0.398432238716943,-2.39872248258723,
7.89073427606518));
#59070=CARTESIAN_POINT('Ctrl Pts',(-1.79914450604067,-1.63575581272393,
7.7796011580736));
#59071=CARTESIAN_POINT('Ctrl Pts',(-2.35007273856783,0.624318747005141,
7.66846804008207));
#59072=CARTESIAN_POINT('Ctrl Pts',(-0.750123138289054,2.3129926228301,7.55733492209049));
#59073=CARTESIAN_POINT('Ctrl Pts',(1.53637104319808,1.884723835474,7.44620180409894));
#59074=CARTESIAN_POINT('Ctrl Pts',(2.41671346511573,-0.26851690501302,7.33506868610738));
#59075=CARTESIAN_POINT('Ctrl Pts',(1.08519321921556,-2.17600323886998,7.22393556811581));
#59076=CARTESIAN_POINT('Ctrl Pts',(-1.23955503582072,-2.09192034816464,
7.11280245012427));
#59077=CARTESIAN_POINT('Ctrl Pts',(-2.42978228173572,-0.0932399608440297,
7.00166933213269));
#59078=CARTESIAN_POINT('Ctrl Pts',(-1.39623723906031,1.99079706988747,6.89053621414115));
#59079=CARTESIAN_POINT('Ctrl Pts',(0.915313888274649,2.25274050986571,6.77940309614957));
#59080=CARTESIAN_POINT('Ctrl Pts',(2.38891436559868,0.452959302820622,6.66826997815803));
#59081=CARTESIAN_POINT('Ctrl Pts',(1.67650552032034,-1.76152590922838,6.55713686016647));
#59082=CARTESIAN_POINT('Ctrl Pts',(-0.571108328568143,-2.36352991238919,
6.4460037421749));
#59083=CARTESIAN_POINT('Ctrl Pts',(-2.2944872436645,-0.802841881741225,
6.33487062418334));
#59084=CARTESIAN_POINT('Ctrl Pts',(-1.92082261731153,1.49360426030822,6.2237375061918));
#59085=CARTESIAN_POINT('Ctrl Pts',(0.216781852341404,2.42116840251458,6.11260438820022));
#59086=CARTESIAN_POINT('Ctrl Pts',(1.50053609517415,1.56487100696715,6.03851564287252));
#59087=CARTESIAN_POINT('Ctrl Pts',(1.81968187503599,0.95980947565199,6.00147127020867));
#59088=CARTESIAN_POINT('Ctrl Pts',(1.26907087985245,1.07935865304843,17.));
#59089=CARTESIAN_POINT('Ctrl Pts',(1.31463335343697,1.03685370088427,17.));
#59090=CARTESIAN_POINT('Ctrl Pts',(1.35743963235178,0.991755207691644,17.));
#59091=CARTESIAN_POINT('Ctrl Pts',(1.39749071248986,0.944412965608489,17.));
#59092=CARTESIAN_POINT('Ctrl Pts',(1.43900564122184,0.895340386309302,17.));
#59093=CARTESIAN_POINT('Ctrl Pts',(1.47756084223886,0.843856601716214,17.));
#59094=CARTESIAN_POINT('Ctrl Pts',(1.51313081159997,0.790300559584653,17.));
#59095=CARTESIAN_POINT('Ctrl Pts',(1.54562908903941,0.74136942056454,17.));
#59096=CARTESIAN_POINT('Ctrl Pts',(1.5756353908389,0.690707426732232,17.));
#59097=CARTESIAN_POINT('Ctrl Pts',(1.60310603850295,0.638543833142686,17.));
#59098=CARTESIAN_POINT('Ctrl Pts',(1.61661334372111,0.612895017413743,17.));
#59099=CARTESIAN_POINT('Ctrl Pts',(1.62950722716312,0.586882786829157,17.));
#59100=CARTESIAN_POINT('Ctrl Pts',(1.64178012375449,0.560532523386325,17.));
#59101=CARTESIAN_POINT('Ctrl Pts',(1.64738432617045,0.548500138940798,17.));
#59102=CARTESIAN_POINT('Ctrl Pts',(1.65285961119358,0.536395613146207,17.));
#59103=CARTESIAN_POINT('Ctrl Pts',(1.65819677046436,0.524241257566197,17.));
#59104=CARTESIAN_POINT('Ctrl Pts',(1.68515739063045,0.462843621196213,17.));
#59105=CARTESIAN_POINT('Ctrl Pts',(1.70864881961265,0.400067692729951,17.));
#59106=CARTESIAN_POINT('Ctrl Pts',(1.72864695641584,0.336272032400955,17.));
#59107=CARTESIAN_POINT('Ctrl Pts',(1.74902990067328,0.271248805429877,17.));
#59108=CARTESIAN_POINT('Ctrl Pts',(1.76578439667341,0.205165384088333,17.));
#59109=CARTESIAN_POINT('Ctrl Pts',(1.77884521789635,0.138364590989932,17.));
#59110=CARTESIAN_POINT('Ctrl Pts',(1.7896907150818,0.0828942801137585,17.));
#59111=CARTESIAN_POINT('Ctrl Pts',(1.79798870333448,0.0269283684180995,
17.));
#59112=CARTESIAN_POINT('Ctrl Pts',(1.80367735161904,-0.029348946606401,
17.));
#59113=CARTESIAN_POINT('Ctrl Pts',(1.80631029137596,-0.0553963963218251,
17.));
#59114=CARTESIAN_POINT('Ctrl Pts',(1.80838392210809,-0.0815106672623466,
17.));
#59115=CARTESIAN_POINT('Ctrl Pts',(1.80989031432926,-0.107673896123635,
17.));
#59116=CARTESIAN_POINT('Ctrl Pts',(1.81054780481405,-0.119093281981834,
17.));
#59117=CARTESIAN_POINT('Ctrl Pts',(1.81109711555612,-0.130521751152742,
17.));
#59118=CARTESIAN_POINT('Ctrl Pts',(1.81153725496673,-0.141943752396311,
17.));
#59119=CARTESIAN_POINT('Ctrl Pts',(1.81423915749931,-0.212060477559016,
17.));
#59120=CARTESIAN_POINT('Ctrl Pts',(1.8128391711499,-0.28206475899935,17.));
#59121=CARTESIAN_POINT('Ctrl Pts',(1.80728215470532,-0.351596341136129,
17.));
#59122=CARTESIAN_POINT('Ctrl Pts',(1.80231577265823,-0.413737672671453,
17.));
#59123=CARTESIAN_POINT('Ctrl Pts',(1.79402871946725,-0.475502410193276,
17.));
#59124=CARTESIAN_POINT('Ctrl Pts',(1.78234854127328,-0.536645515067971,
17.));
#59125=CARTESIAN_POINT('Ctrl Pts',(1.76958920689471,-0.603437759765362,
17.));
#59126=CARTESIAN_POINT('Ctrl Pts',(1.75278190243293,-0.669489034899465,
17.));
#59127=CARTESIAN_POINT('Ctrl Pts',(1.73217389519949,-0.734583882594501,
17.));
#59128=CARTESIAN_POINT('Ctrl Pts',(1.7242846189666,-0.759503867772431,17.));
#59129=CARTESIAN_POINT('Ctrl Pts',(1.7158377768979,-0.78428363611299,17.));
#59130=CARTESIAN_POINT('Ctrl Pts',(1.70684526783583,-0.808910785136196,
17.));
#59131=CARTESIAN_POINT('Ctrl Pts',(1.7028767076987,-0.819779200305976,17.));
#59132=CARTESIAN_POINT('Ctrl Pts',(1.69880197156565,-0.830617330567754,
17.));
#59133=CARTESIAN_POINT('Ctrl Pts',(1.69462717263472,-0.841411562228869,
17.));
#59134=CARTESIAN_POINT('Ctrl Pts',(1.66964189956069,-0.906012715515375,
17.));
#59135=CARTESIAN_POINT('Ctrl Pts',(1.64103489494096,-0.969158501636665,
17.));
#59136=CARTESIAN_POINT('Ctrl Pts',(1.60911056531399,-1.03063593785474,17.));
#59137=CARTESIAN_POINT('Ctrl Pts',(1.57635918906639,-1.09370603730061,17.));
#59138=CARTESIAN_POINT('Ctrl Pts',(1.54011611570736,-1.15502101490558,17.));
#59139=CARTESIAN_POINT('Ctrl Pts',(1.50065541627137,-1.21434743041401,17.));
#59140=CARTESIAN_POINT('Ctrl Pts',(1.46751534688147,-1.26417121850455,17.));
#59141=CARTESIAN_POINT('Ctrl Pts',(1.43210475062568,-1.31259265519435,17.));
#59142=CARTESIAN_POINT('Ctrl Pts',(1.39455982747634,-1.3594652647581,17.));
#59143=CARTESIAN_POINT('Ctrl Pts',(1.37456954356258,-1.38442194849485,17.));
#59144=CARTESIAN_POINT('Ctrl Pts',(1.35397457645813,-1.40893853932649,17.));
#59145=CARTESIAN_POINT('Ctrl Pts',(1.33279075072117,-1.43299413795622,17.));
#59146=CARTESIAN_POINT('Ctrl Pts',(1.31937221833251,-1.44823174580618,17.));
#59147=CARTESIAN_POINT('Ctrl Pts',(1.3057160205887,-1.46328534776906,17.));
#59148=CARTESIAN_POINT('Ctrl Pts',(1.29185135791409,-1.47812325485253,17.));
#59149=CARTESIAN_POINT('Ctrl Pts',(1.24079790013097,-1.53276046317518,17.));
#59150=CARTESIAN_POINT('Ctrl Pts',(1.1868605733564,-1.58454679540276,17.));
#59151=CARTESIAN_POINT('Ctrl Pts',(1.1303228346641,-1.63321750971738,17.));
#59152=CARTESIAN_POINT('Ctrl Pts',(1.08987767577489,-1.66803486922337,17.));
#59153=CARTESIAN_POINT('Ctrl Pts',(1.04810062967973,-1.70125755846181,17.));
#59154=CARTESIAN_POINT('Ctrl Pts',(1.00508147489063,-1.73278020099862,17.));
#59155=CARTESIAN_POINT('Ctrl Pts',(0.991017431819989,-1.7430857452268,17.));
#59156=CARTESIAN_POINT('Ctrl Pts',(0.976820548550378,-1.75320951848906,
17.));
#59157=CARTESIAN_POINT('Ctrl Pts',(0.962493729450331,-1.76314761869876,
17.));
#59158=CARTESIAN_POINT('Ctrl Pts',(0.948700205378558,-1.77271578756534,
17.));
#59159=CARTESIAN_POINT('Ctrl Pts',(0.934793273211275,-1.78210690615323,
17.));
#59160=CARTESIAN_POINT('Ctrl Pts',(0.920780914430478,-1.79131474048402,
17.));
#59161=CARTESIAN_POINT('Ctrl Pts',(0.857817216437198,-1.83268959457145,
17.));
#59162=CARTESIAN_POINT('Ctrl Pts',(0.792697129221742,-1.87038775038027,
17.));
#59163=CARTESIAN_POINT('Ctrl Pts',(0.725682411188942,-1.90412957333601,
17.));
#59164=CARTESIAN_POINT('Ctrl Pts',(0.674447265301284,-1.92992640233717,
17.));
#59165=CARTESIAN_POINT('Ctrl Pts',(0.622103705214267,-1.95341028870243,
17.));
#59166=CARTESIAN_POINT('Ctrl Pts',(0.56875484042429,-1.97444100905915,17.));
#59167=CARTESIAN_POINT('Ctrl Pts',(0.556450338865399,-1.97929158146463,
17.));
#59168=CARTESIAN_POINT('Ctrl Pts',(0.544092316022985,-1.98401158984533,
17.));
#59169=CARTESIAN_POINT('Ctrl Pts',(0.531682642424069,-1.98860160490479,
17.));
#59170=CARTESIAN_POINT('Ctrl Pts',(-0.530822314817812,-1.98761604614028,
16.9985408643923));
#59171=CARTESIAN_POINT('Ctrl Pts',(-1.19172355532747,-1.81111257755813,
16.9614964917284));
#59172=CARTESIAN_POINT('Ctrl Pts',(-2.31220282305949,-0.750101418116348,
16.8874077464009));
#59173=CARTESIAN_POINT('Ctrl Pts',(-1.88356022517535,1.54029064361322,16.7762746284092));
#59174=CARTESIAN_POINT('Ctrl Pts',(0.272138683002673,2.41558334409046,16.6651415104176));
#59175=CARTESIAN_POINT('Ctrl Pts',(2.17716537292403,1.08271362067439,16.5540083924261));
#59176=CARTESIAN_POINT('Ctrl Pts',(2.09039692632852,-1.24248312461781,16.4428752744345));
#59177=CARTESIAN_POINT('Ctrl Pts',(0.0899798428231618,-2.42978715040514,
16.331742156443));
#59178=CARTESIAN_POINT('Ctrl Pts',(-1.99256263878865,-1.39363276224998,
16.2206090384514));
#59179=CARTESIAN_POINT('Ctrl Pts',(-2.25155255412213,0.918227258501085,
16.1094759204598));
#59180=CARTESIAN_POINT('Ctrl Pts',(-0.449770559963355,2.38958586423339,
15.9983428024683));
#59181=CARTESIAN_POINT('Ctrl Pts',(1.76362649251955,1.67395571200075,15.8872096844767));
#59182=CARTESIAN_POINT('Ctrl Pts',(2.36290026085259,-0.573773007815998,
15.7760765664852));
#59183=CARTESIAN_POINT('Ctrl Pts',(0.799545757360654,-2.29634721328381,
15.6649434484936));
#59184=CARTESIAN_POINT('Ctrl Pts',(-1.4955798077745,-1.91722185216344,15.553810330502));
#59185=CARTESIAN_POINT('Ctrl Pts',(-2.42189432006925,0.216624485203865,
15.4426772125105));
#59186=CARTESIAN_POINT('Ctrl Pts',(-1.13159454186566,2.15220543372035,15.3315440945189));
#59187=CARTESIAN_POINT('Ctrl Pts',(1.19438442805909,2.11800437629149,15.2204109765274));
#59188=CARTESIAN_POINT('Ctrl Pts',(2.42721611075584,0.145321765122002,15.1092778585358));
#59189=CARTESIAN_POINT('Ctrl Pts',(1.43856389040869,-1.96036473920531,14.9981447405443));
#59190=CARTESIAN_POINT('Ctrl Pts',(-0.86671852734562,-2.27184843524121,
14.8870116225527));
#59191=CARTESIAN_POINT('Ctrl Pts',(-2.37874608563758,-0.504046940381654,
14.7758785045611));
#59192=CARTESIAN_POINT('Ctrl Pts',(-1.71365157339857,1.72507810949981,14.6647453865696));
#59193=CARTESIAN_POINT('Ctrl Pts',(0.519844293652045,2.37534379814029,14.553612268578));
#59194=CARTESIAN_POINT('Ctrl Pts',(2.27755820952083,0.851601338069138,14.4424791505865));
#59195=CARTESIAN_POINT('Ctrl Pts',(1.95076120442826,-1.45156017900596,14.3313460325949));
#59196=CARTESIAN_POINT('Ctrl Pts',(-0.161449234185697,-2.4261966907003,
14.2202129146033));
#59197=CARTESIAN_POINT('Ctrl Pts',(-2.12589498013164,-1.18028249516839,
14.1090797966117));
#59198=CARTESIAN_POINT('Ctrl Pts',(-2.14463796530634,1.14587269450434,13.9979466786202));
#59199=CARTESIAN_POINT('Ctrl Pts',(-0.200523872789563,2.42328009352997,
13.8868135606286));
#59200=CARTESIAN_POINT('Ctrl Pts',(1.92711756079595,1.4828061713343,13.7756804426371));
#59201=CARTESIAN_POINT('Ctrl Pts',(2.29098515205495,-0.814790321419068,
13.6645473246455));
#59202=CARTESIAN_POINT('Ctrl Pts',(0.558052959897197,-2.36665864224302,
13.553414206654));
#59203=CARTESIAN_POINT('Ctrl Pts',(-1.68563126593031,-1.7524678228742,13.4422810886624));
#59204=CARTESIAN_POINT('Ctrl Pts',(-2.38655941136709,0.465650524431861,
13.3311479706708));
#59205=CARTESIAN_POINT('Ctrl Pts',(-0.903214449463494,2.25758718396156,
13.2200148526793));
#59206=CARTESIAN_POINT('Ctrl Pts',(1.40678792676647,1.98329119495888,13.1088817346877));
#59207=CARTESIAN_POINT('Ctrl Pts',(2.42924262178492,-0.106190957248261,
12.9977486166962));
#59208=CARTESIAN_POINT('Ctrl Pts',(1.22835885528878,-2.09848296574785,12.8866154987046));
#59209=CARTESIAN_POINT('Ctrl Pts',(-1.09676728330151,-2.17016076850958,
12.7754823807131));
#59210=CARTESIAN_POINT('Ctrl Pts',(-2.41808883587442,-0.255622019236254,
12.6643492627215));
#59211=CARTESIAN_POINT('Ctrl Pts',(-1.52628031080604,1.89287206322695,12.5532161447299));
#59212=CARTESIAN_POINT('Ctrl Pts',(0.762440028519717,2.30893513070632,12.4420830267384));
#59213=CARTESIAN_POINT('Ctrl Pts',(2.35334524439711,0.611769887762175,12.3309499087468));
#59214=CARTESIAN_POINT('Ctrl Pts',(1.79037626583608,-1.64531123549009,12.2198167907553));
#59215=CARTESIAN_POINT('Ctrl Pts',(-0.411215539741278,-2.39653875720262,
12.1086836727637));
#59216=CARTESIAN_POINT('Ctrl Pts',(-2.23644669806148,-0.954359681477023,
11.9975505547722));
#59217=CARTESIAN_POINT('Ctrl Pts',(-2.01479381263157,1.36128693796739,11.8864174367806));
#59218=CARTESIAN_POINT('Ctrl Pts',(0.0508776716304708,2.43103017205227,
11.775284318789));
#59219=CARTESIAN_POINT('Ctrl Pts',(2.06998390829065,1.27579890825976,11.6641512007974));
#59220=CARTESIAN_POINT('Ctrl Pts',(2.19455939831053,-1.0470937313278,11.5530180828059));
#59221=CARTESIAN_POINT('Ctrl Pts',(0.310587749980402,-2.41164497479648,
11.4418849648143));
#59222=CARTESIAN_POINT('Ctrl Pts',(-1.8576460317465,-1.5689638159102,11.3307518468228));
#59223=CARTESIAN_POINT('Ctrl Pts',(-2.3256890489837,0.709694781111127,11.2196187288312));
#59224=CARTESIAN_POINT('Ctrl Pts',(-0.665169910362038,2.33881278114516,
11.1084856108397));
#59225=CARTESIAN_POINT('Ctrl Pts',(1.6041389110555,1.82735726910112,10.9973524928481));
#59226=CARTESIAN_POINT('Ctrl Pts',(2.40527666278277,-0.3565675397055,10.8862193748566));
#59227=CARTESIAN_POINT('Ctrl Pts',(1.00501054196433,-2.21414770181206,10.775086256865));
#59228=CARTESIAN_POINT('Ctrl Pts',(-1.31508078368933,-2.04525273921589,
10.6639531388734));
#59229=CARTESIAN_POINT('Ctrl Pts',(-2.43155841503526,-0.00446196932597716,
10.5528200208819));
#59230=CARTESIAN_POINT('Ctrl Pts',(-1.32257807973431,2.04041257051249,10.4416869028903));
#59231=CARTESIAN_POINT('Ctrl Pts',(0.996877770305409,2.21782121596171,10.3305537848988));
#59232=CARTESIAN_POINT('Ctrl Pts',(2.40395184823498,0.365392591970382,10.2194206669072));
#59233=CARTESIAN_POINT('Ctrl Pts',(1.61083457603706,-1.82145771390455,10.1082875489157));
#59234=CARTESIAN_POINT('Ctrl Pts',(-0.656581901980842,-2.34123822813698,
9.99715443092411));
#59235=CARTESIAN_POINT('Ctrl Pts',(-2.32306878049448,-0.718225365739856,
9.88602131293258));
#59236=CARTESIAN_POINT('Ctrl Pts',(-1.86339167600253,1.56213562045755,9.77488819494099));
#59237=CARTESIAN_POINT('Ctrl Pts',(0.301734832747034,2.41276860175285,9.66375507694945));
#59238=CARTESIAN_POINT('Ctrl Pts',(2.19070174640221,1.05514079307809,9.55262195895788));
#59239=CARTESIAN_POINT('Ctrl Pts',(2.07465219656388,-1.26819339936035,9.44148884096632));
#59240=CARTESIAN_POINT('Ctrl Pts',(0.059799298926456,-2.43082707709519,
9.33035572297477));
#59241=CARTESIAN_POINT('Ctrl Pts',(-2.00978427078675,-1.36867213745724,
9.21922260498321));
#59242=CARTESIAN_POINT('Ctrl Pts',(-2.23993417149811,0.946145412803733,
9.10808948699165));
#59243=CARTESIAN_POINT('Ctrl Pts',(-0.420008155580443,2.39501344132368,
8.99695636900008));
#59244=CARTESIAN_POINT('Ctrl Pts',(1.78432585582941,1.65187090157668,8.88582325100852));
#59245=CARTESIAN_POINT('Ctrl Pts',(2.35557461332577,-0.603128904380432,
8.77469013301699));
#59246=CARTESIAN_POINT('Ctrl Pts',(0.770908770722433,-2.30612139796956,
8.6635570150254));
#59247=CARTESIAN_POINT('Ctrl Pts',(-1.51932312253082,-1.8984608203825,8.55242389703386));
#59248=CARTESIAN_POINT('Ctrl Pts',(-2.41901069213679,0.246745823280066,
8.44129077904229));
#59249=CARTESIAN_POINT('Ctrl Pts',(-1.10472446865624,2.16612097656366,8.33015766105073));
#59250=CARTESIAN_POINT('Ctrl Pts',(1.22064907711907,2.10297695649155,8.21902454305917));
#59251=CARTESIAN_POINT('Ctrl Pts',(2.42883652976957,0.115105649486712,8.10789142506762));
#59252=CARTESIAN_POINT('Ctrl Pts',(1.41405721802439,-1.97811487082963,7.99675830707606));
#59253=CARTESIAN_POINT('Ctrl Pts',(-0.89492296554583,-2.26088681806294,
7.88562518908451));
#59254=CARTESIAN_POINT('Ctrl Pts',(-2.38483433335392,-0.474406133986129,
7.77449207109293));
#59255=CARTESIAN_POINT('Ctrl Pts',(-1.69205163242953,1.74626966328898,7.66335895310138));
#59256=CARTESIAN_POINT('Ctrl Pts',(0.549363663544479,2.368690833595,7.55222583510981));
#59257=CARTESIAN_POINT('Ctrl Pts',(2.28797905753948,0.823192728573481,7.44109271711826));
#59258=CARTESIAN_POINT('Ctrl Pts',(1.93254721410632,-1.47572339224646,7.32995959912669));
#59259=CARTESIAN_POINT('Ctrl Pts',(-0.191630291862095,-2.4240000872683,
7.21882648113514));
#59260=CARTESIAN_POINT('Ctrl Pts',(-2.14041565072953,-1.15373514472855,
7.10769336314358));
#59261=CARTESIAN_POINT('Ctrl Pts',(-2.13021707383623,1.17247103400131,6.99656024515202));
#59262=CARTESIAN_POINT('Ctrl Pts',(-0.170343340793051,2.42559050070374,
6.88542712716047));
#59263=CARTESIAN_POINT('Ctrl Pts',(1.94540352455545,1.45870466023832,6.77429400916891));
#59264=CARTESIAN_POINT('Ctrl Pts',(2.28070125668873,-0.843227122409361,
6.66316089117734));
#59265=CARTESIAN_POINT('Ctrl Pts',(0.528495394995496,-2.37343859473579,
6.55202777318578));
#59266=CARTESIAN_POINT('Ctrl Pts',(-1.70718858770076,-1.73132004390081,
6.44089465519424));
#59267=CARTESIAN_POINT('Ctrl Pts',(-2.38080986332144,0.495245413179216,
6.32976153720266));
#59268=CARTESIAN_POINT('Ctrl Pts',(-0.874610928483785,2.26878239794609,
6.21862841921112));
#59269=CARTESIAN_POINT('Ctrl Pts',(1.43051727062736,1.96538105553873,6.10749530121955));
#59270=CARTESIAN_POINT('Ctrl Pts',(2.42936606799034,-0.135922390952342,
5.99636218322799));
#59271=CARTESIAN_POINT('Ctrl Pts',(1.19867795027514,-2.1148820515815,5.88521633177802));
#59272=CARTESIAN_POINT('Ctrl Pts',(-0.344613920714289,-2.14055559361498,
5.81111485299191));
#59273=CARTESIAN_POINT('Ctrl Pts',(-0.951346992282116,-1.82409669095297,
5.77405774686964));
#59274=CARTESIAN_POINT('Ctrl Pts',(-0.496914232204698,-1.8606503040938,
17.0744136915879));
#59275=CARTESIAN_POINT('Ctrl Pts',(-1.11559815585193,-1.69542159549652,
17.037369318924));
#59276=CARTESIAN_POINT('Ctrl Pts',(-2.16450299553907,-0.702186136215599,
16.9632805735963));
#59277=CARTESIAN_POINT('Ctrl Pts',(-1.76324140296468,1.44189933463109,16.8521474556048));
#59278=CARTESIAN_POINT('Ctrl Pts',(0.25475489809407,2.26127973381666,16.7410143376132));
#59279=CARTESIAN_POINT('Ctrl Pts',(2.03809152228371,1.01355160191342,16.6298812196215));
#59280=CARTESIAN_POINT('Ctrl Pts',(1.95686570562903,-1.16311528483624,16.51874810163));
#59281=CARTESIAN_POINT('Ctrl Pts',(0.0842320740146667,-2.27457622364427,
16.4076149836385));
#59282=CARTESIAN_POINT('Ctrl Pts',(-1.86528091629542,-1.30460972475591,
16.296481865647));
#59283=CARTESIAN_POINT('Ctrl Pts',(-2.10772696902188,0.859572366139308,
16.1853487476554));
#59284=CARTESIAN_POINT('Ctrl Pts',(-0.421039934142888,2.23694293149729,
16.0742156296637));
#59285=CARTESIAN_POINT('Ctrl Pts',(1.65096884581237,1.56702609169514,15.9630825116722));
#59286=CARTESIAN_POINT('Ctrl Pts',(2.21196196188707,-0.537121303456362,
15.8519493936807));
#59287=CARTESIAN_POINT('Ctrl Pts',(0.748472049950942,-2.14966021682032,
15.7408162756892));
#59288=CARTESIAN_POINT('Ctrl Pts',(-1.40004455565548,-1.79475277892349,
15.6296831576976));
#59289=CARTESIAN_POINT('Ctrl Pts',(-2.26718757471825,0.202786858685022,
15.518550039706));
#59290=CARTESIAN_POINT('Ctrl Pts',(-1.0593100878421,2.01472598417605,15.4074169217145));
#59291=CARTESIAN_POINT('Ctrl Pts',(1.11808905627853,1.98270963573244,15.296283803723));
#59292=CARTESIAN_POINT('Ctrl Pts',(2.272169417906,0.136038842607842,15.1851506857314));
#59293=CARTESIAN_POINT('Ctrl Pts',(1.34667072412956,-1.83513976716994,15.0740175677399));
#59294=CARTESIAN_POINT('Ctrl Pts',(-0.811353930554621,-2.12672638163449,
14.9628844497482));
#59295=CARTESIAN_POINT('Ctrl Pts',(-2.22679558066473,-0.471849225970919,
14.8517513317567));
#59296=CARTESIAN_POINT('Ctrl Pts',(-1.60418624479641,1.61488287200104,14.740618213765));
#59297=CARTESIAN_POINT('Ctrl Pts',(0.486637469517006,2.22361062586486,14.6294850957736));
#59298=CARTESIAN_POINT('Ctrl Pts',(2.13207142464232,0.79720240321163,14.518351977782));
#59299=CARTESIAN_POINT('Ctrl Pts',(1.82614969087327,-1.35883683054512,14.4072188597905));
#59300=CARTESIAN_POINT('Ctrl Pts',(-0.151136114677013,-2.27121511677727,
14.2960857417988));
#59301=CARTESIAN_POINT('Ctrl Pts',(-1.99009620038771,-1.10488793236309,
14.1849526238074));
#59302=CARTESIAN_POINT('Ctrl Pts',(-2.00764191357142,1.07267617486913,14.0738195058158));
#59303=CARTESIAN_POINT('Ctrl Pts',(-0.187714727705331,2.26848482718112,
13.9626863878241));
#59304=CARTESIAN_POINT('Ctrl Pts',(1.80401636547585,1.38808687873242,13.8515532698327));
#59305=CARTESIAN_POINT('Ctrl Pts',(2.14464067550829,-0.76274281557801,13.7404201518411));
#59306=CARTESIAN_POINT('Ctrl Pts',(0.522405427119336,-2.21548026387029,
13.6292870338496));
#59307=CARTESIAN_POINT('Ctrl Pts',(-1.57795582986649,-1.64052297418177,
13.518153915858));
#59308=CARTESIAN_POINT('Ctrl Pts',(-2.23410980361178,0.435905511815549,
13.4070207978665));
#59309=CARTESIAN_POINT('Ctrl Pts',(-0.845518551392067,2.11337611633463,
13.2958876798749));
#59310=CARTESIAN_POINT('Ctrl Pts',(1.31692455835042,1.85660171750613,13.1847545618833));
#59311=CARTESIAN_POINT('Ctrl Pts',(2.27406647864359,-0.0994076483130035,
13.0736214438918));
#59312=CARTESIAN_POINT('Ctrl Pts',(1.14989325129853,-1.96443522175046,12.9624883259002));
#59313=CARTESIAN_POINT('Ctrl Pts',(-1.02670753899269,-2.03153436082434,
12.8513552079086));
#59314=CARTESIAN_POINT('Ctrl Pts',(-2.26362517878265,-0.239293292458876,
12.7402220899171));
#59315=CARTESIAN_POINT('Ctrl Pts',(-1.42878395953199,1.77195841565734,12.6290889719255));
#59316=CARTESIAN_POINT('Ctrl Pts',(0.713736575871035,2.16144403816025,12.517955853934));
#59317=CARTESIAN_POINT('Ctrl Pts',(2.20301730463899,0.572691003330619,12.4068227359424));
#59318=CARTESIAN_POINT('Ctrl Pts',(1.6760098862852,-1.54021137864547,12.2956896179507));
#59319=CARTESIAN_POINT('Ctrl Pts',(-0.384947747103115,-2.24345168475608,
12.1845564999592));
#59320=CARTESIAN_POINT('Ctrl Pts',(-2.09358605094697,-0.893396707580089,
12.0734233819677));
#59321=CARTESIAN_POINT('Ctrl Pts',(-1.88609199822018,1.27433010012496,11.9622902639762));
#59322=CARTESIAN_POINT('Ctrl Pts',(0.0476276871353746,2.27573984305167,
11.8511571459845));
#59323=CARTESIAN_POINT('Ctrl Pts',(1.93775663861714,1.19430290937011,11.740024027993));
#59324=CARTESIAN_POINT('Ctrl Pts',(2.05437444507841,-0.980207054271423,
11.6288909100015));
#59325=CARTESIAN_POINT('Ctrl Pts',(0.29074790001371,-2.25759294127003,11.5177577920098));
#59326=CARTESIAN_POINT('Ctrl Pts',(-1.73898256686937,-1.46874091042604,
11.4066246740184));
#59327=CARTESIAN_POINT('Ctrl Pts',(-2.17712774286675,0.664360610718776,
11.2954915560267));
#59328=CARTESIAN_POINT('Ctrl Pts',(-0.622679917679542,2.18941315195494,
11.1843584380353));
#59329=CARTESIAN_POINT('Ctrl Pts',(1.5016690766107,1.71062860206002,11.0732253200437));
#59330=CARTESIAN_POINT('Ctrl Pts',(2.25163142686794,-0.333790574125898,
10.962092202052));
#59331=CARTESIAN_POINT('Ctrl Pts',(0.940812071906275,-2.07271147900283,
10.8509590840606));
#59332=CARTESIAN_POINT('Ctrl Pts',(-1.23107552126632,-1.91460525716752,
10.7398259660689));
#59333=CARTESIAN_POINT('Ctrl Pts',(-2.27623434271564,-0.00417694584392041,
10.6286928480775));
#59334=CARTESIAN_POINT('Ctrl Pts',(-1.2380939020009,1.91007427071903,10.5175597300858));
#59335=CARTESIAN_POINT('Ctrl Pts',(0.933198808726156,2.07615033492922,10.4064266120944));
#59336=CARTESIAN_POINT('Ctrl Pts',(2.2503912393599,0.342051896131316,10.2952934941028));
#59337=CARTESIAN_POINT('Ctrl Pts',(1.50793703319531,-1.70510590103744,10.1841603761111));
#59338=CARTESIAN_POINT('Ctrl Pts',(-0.614640497572694,-2.19168366526239,
10.0730272581197));
#59339=CARTESIAN_POINT('Ctrl Pts',(-2.17467485294833,-0.672346275210854,
9.96189414012807));
#59340=CARTESIAN_POINT('Ctrl Pts',(-1.74436118853674,1.46234888920541,9.85076102213649));
#59341=CARTESIAN_POINT('Ctrl Pts',(0.28246049300954,2.25864479272903,9.73962790414495));
#59342=CARTESIAN_POINT('Ctrl Pts',(2.05076321381961,0.987740082555135,9.62849478615337));
#59343=CARTESIAN_POINT('Ctrl Pts',(1.94212672408311,-1.18718322824561,9.51736166816183));
#59344=CARTESIAN_POINT('Ctrl Pts',(0.0559794151129784,-2.27554972147643,
9.40622855017026));
#59345=CARTESIAN_POINT('Ctrl Pts',(-1.88140245791634,-1.28124354485353,
9.29509543217871));
#59346=CARTESIAN_POINT('Ctrl Pts',(-2.09685075014427,0.885707153284858,
9.18396231418714));
#59347=CARTESIAN_POINT('Ctrl Pts',(-0.393178704669941,2.24202380362205,
9.07282919619558));
#59348=CARTESIAN_POINT('Ctrl Pts',(1.67034596681712,1.54635202372753,8.96169607820403));
#59349=CARTESIAN_POINT('Ctrl Pts',(2.20510426503715,-0.564601992181745,
8.85056296021247));
#59350=CARTESIAN_POINT('Ctrl Pts',(0.721664348332612,-2.15881004218177,
8.73942984222091));
#59351=CARTESIAN_POINT('Ctrl Pts',(-1.42227118534451,-1.77719017192194,
8.62829672422935));
#59352=CARTESIAN_POINT('Ctrl Pts',(-2.26448814833767,0.230984093739564,
8.5171636062378));
#59353=CARTESIAN_POINT('Ctrl Pts',(-1.0341564320416,2.02775262434295,8.40603048824622));
#59354=CARTESIAN_POINT('Ctrl Pts',(1.14267596145836,1.96864214353504,8.29489737025468));
#59355=CARTESIAN_POINT('Ctrl Pts',(2.27368632713831,0.107752884233482,8.1837642522631));
#59356=CARTESIAN_POINT('Ctrl Pts',(1.32372949887998,-1.85175604870411,8.07263113427156));
#59357=CARTESIAN_POINT('Ctrl Pts',(-0.837756714239087,-2.11646497507375,
7.96149801627999));
#59358=CARTESIAN_POINT('Ctrl Pts',(-2.23249492082995,-0.44410182699992,
7.85036489828844));
#59359=CARTESIAN_POINT('Ctrl Pts',(-1.5839660735966,1.6347207431425,7.73923178029686));
#59360=CARTESIAN_POINT('Ctrl Pts',(0.514271189154998,2.21738264208079,7.62809866230533));
#59361=CARTESIAN_POINT('Ctrl Pts',(2.14182660551464,0.770608490368339,7.51696554431375));
#59362=CARTESIAN_POINT('Ctrl Pts',(1.80909918119506,-1.38145653627306,7.4058324263222));
#59363=CARTESIAN_POINT('Ctrl Pts',(-0.179389254538965,-2.26915882886811,
7.29469930833064));
#59364=CARTESIAN_POINT('Ctrl Pts',(-2.00368931371364,-1.08003638431653,
7.18356619033908));
#59365=CARTESIAN_POINT('Ctrl Pts',(-1.99414220564178,1.09757545487321,7.07243307234752));
#59366=CARTESIAN_POINT('Ctrl Pts',(-0.159462079943669,2.27064764923059,
6.96129995435596));
#59367=CARTESIAN_POINT('Ctrl Pts',(1.82113425104325,1.36552493371444,6.85016683636441));
#59368=CARTESIAN_POINT('Ctrl Pts',(2.13501369897146,-0.789363119088234,
6.73903371837284));
#59369=CARTESIAN_POINT('Ctrl Pts',(0.494735952308336,-2.22182712381435,
6.62790060038128));
#59370=CARTESIAN_POINT('Ctrl Pts',(-1.59813610431413,-1.62072608159068,
6.51676748238972));
#59371=CARTESIAN_POINT('Ctrl Pts',(-2.22872752752264,0.463609926284491,
6.40563436439817));
#59372=CARTESIAN_POINT('Ctrl Pts',(-0.818742177699371,2.12385619791032,
6.29450124640661));
#59373=CARTESIAN_POINT('Ctrl Pts',(1.33913810958254,1.83983564921886,6.18336812841505));
#59374=CARTESIAN_POINT('Ctrl Pts',(2.27418203930235,-0.127239885464669,
6.07223501042349));
#59375=CARTESIAN_POINT('Ctrl Pts',(1.12210831514517,-1.97978676014366,5.96108915897352));
#59376=CARTESIAN_POINT('Ctrl Pts',(-0.322600533245414,-2.00382031727082,
5.8869876801874));
#59377=CARTESIAN_POINT('Ctrl Pts',(-0.890576464164601,-1.70757630444214,
5.84993057406514));
#59378=CARTESIAN_POINT('Ctrl Pts',(-0.463006149591583,-1.73368456204731,
17.1502865187834));
#59379=CARTESIAN_POINT('Ctrl Pts',(-1.03947275637638,-1.5797306134349,17.1132421461195));
#59380=CARTESIAN_POINT('Ctrl Pts',(-2.01680316801866,-0.65427085431485,
17.0391534007918));
#59381=CARTESIAN_POINT('Ctrl Pts',(-1.64292258075401,1.34350802564897,16.9280202828002));
#59382=CARTESIAN_POINT('Ctrl Pts',(0.237371113185469,2.10697612354286,16.8168871648087));
#59383=CARTESIAN_POINT('Ctrl Pts',(1.89901767164339,0.944389583152448,16.7057540468171));
#59384=CARTESIAN_POINT('Ctrl Pts',(1.82333448492954,-1.08374744505468,16.5946209288256));
#59385=CARTESIAN_POINT('Ctrl Pts',(0.0784843052061702,-2.11936529688341,
16.483487810834));
#59386=CARTESIAN_POINT('Ctrl Pts',(-1.7379991938022,-1.21558668726184,16.3723546928424));
#59387=CARTESIAN_POINT('Ctrl Pts',(-1.96390138392162,0.80091747377753,16.2612215748509));
#59388=CARTESIAN_POINT('Ctrl Pts',(-0.39230930832242,2.08429999876119,16.1500884568593));
#59389=CARTESIAN_POINT('Ctrl Pts',(1.5383111991052,1.46009647138952,16.0389553388678));
#59390=CARTESIAN_POINT('Ctrl Pts',(2.06102366292156,-0.500469599096727,
15.9278222208762));
#59391=CARTESIAN_POINT('Ctrl Pts',(0.697398342541232,-2.00297322035683,
15.8166891028847));
#59392=CARTESIAN_POINT('Ctrl Pts',(-1.30450930353645,-1.67228370568353,
15.7055559848931));
#59393=CARTESIAN_POINT('Ctrl Pts',(-2.11248082936726,0.188949232166182,
15.5944228669016));
#59394=CARTESIAN_POINT('Ctrl Pts',(-0.987025633818535,1.87724653463175,
15.48328974891));
#59395=CARTESIAN_POINT('Ctrl Pts',(1.04179368449796,1.84741489517339,15.3721566309185));
#59396=CARTESIAN_POINT('Ctrl Pts',(2.11712272505618,0.126755920093683,15.2610235129269));
#59397=CARTESIAN_POINT('Ctrl Pts',(1.25477755785045,-1.70991479513458,15.1498903949353));
#59398=CARTESIAN_POINT('Ctrl Pts',(-0.755989333763624,-1.98160432802777,
15.0387572769437));
#59399=CARTESIAN_POINT('Ctrl Pts',(-2.07484507569188,-0.439651511560185,
14.9276241589522));
#59400=CARTESIAN_POINT('Ctrl Pts',(-1.49472091619425,1.50468763450227,14.8164910409607));
#59401=CARTESIAN_POINT('Ctrl Pts',(0.453430645381966,2.07187745358944,14.705357922969));
#59402=CARTESIAN_POINT('Ctrl Pts',(1.98658463976382,0.742803468354118,14.5942248049775));
#59403=CARTESIAN_POINT('Ctrl Pts',(1.70153817731828,-1.26611348208428,14.4830916869859));
#59404=CARTESIAN_POINT('Ctrl Pts',(-0.140822995168328,-2.11623354285424,
14.3719585689944));
#59405=CARTESIAN_POINT('Ctrl Pts',(-1.85429742064377,-1.02949336955781,
14.2608254510028));
#59406=CARTESIAN_POINT('Ctrl Pts',(-1.87064586183651,0.999479655233932,
14.1496923330113));
#59407=CARTESIAN_POINT('Ctrl Pts',(-0.174905582621096,2.11368956083228,
14.0385592150197));
#59408=CARTESIAN_POINT('Ctrl Pts',(1.68091517015576,1.29336758613053,13.9274260970282));
#59409=CARTESIAN_POINT('Ctrl Pts',(1.99829619896164,-0.710695309736953,
13.8162929790366));
#59410=CARTESIAN_POINT('Ctrl Pts',(0.486757894341478,-2.06430188549755,
13.7051598610451));
#59411=CARTESIAN_POINT('Ctrl Pts',(-1.47028039380267,-1.52857812548934,
13.5940267430535));
#59412=CARTESIAN_POINT('Ctrl Pts',(-2.08166019585647,0.406160499199236,
13.4828936250619));
#59413=CARTESIAN_POINT('Ctrl Pts',(-0.787822653320641,1.96916504870769,
13.3717605070704));
#59414=CARTESIAN_POINT('Ctrl Pts',(1.22706118993438,1.72991224005338,13.2606273890788));
#59415=CARTESIAN_POINT('Ctrl Pts',(2.11889033550226,-0.0926243393777398,
13.1494942710872));
#59416=CARTESIAN_POINT('Ctrl Pts',(1.07142764730828,-1.83038747775309,13.0383611530957));
#59417=CARTESIAN_POINT('Ctrl Pts',(-0.956647794683878,-1.89290795313909,
12.9272280351041));
#59418=CARTESIAN_POINT('Ctrl Pts',(-2.10916152169086,-0.222964565681501,
12.8160949171126));
#59419=CARTESIAN_POINT('Ctrl Pts',(-1.33128760825794,1.65104476808775,12.704961799121));
#59420=CARTESIAN_POINT('Ctrl Pts',(0.665033123222356,2.01395294561419,12.5938286811294));
#59421=CARTESIAN_POINT('Ctrl Pts',(2.05268936488087,0.533612118899064,12.4826955631379));
#59422=CARTESIAN_POINT('Ctrl Pts',(1.56164350673432,-1.43511152180085,12.3715624451463));
#59423=CARTESIAN_POINT('Ctrl Pts',(-0.358679954464953,-2.09036461230954,
12.2604293271548));
#59424=CARTESIAN_POINT('Ctrl Pts',(-1.95072540383246,-0.832433733683153,
12.1492962091632));
#59425=CARTESIAN_POINT('Ctrl Pts',(-1.7573901838088,1.18737326228254,12.0381630911717));
#59426=CARTESIAN_POINT('Ctrl Pts',(0.0443777026402783,2.12044951405105,
11.9270299731801));
#59427=CARTESIAN_POINT('Ctrl Pts',(1.80552936894361,1.11280691048046,11.8158968551885));
#59428=CARTESIAN_POINT('Ctrl Pts',(1.91418949184629,-0.913320377215045,
11.704763737197));
#59429=CARTESIAN_POINT('Ctrl Pts',(0.270908050047019,-2.10354090774357,
11.5936306192054));
#59430=CARTESIAN_POINT('Ctrl Pts',(-1.62031910199222,-1.36851800494188,
11.4824975012139));
#59431=CARTESIAN_POINT('Ctrl Pts',(-2.0285664367498,0.619026440326427,11.3713643832223));
#59432=CARTESIAN_POINT('Ctrl Pts',(-0.580189924997046,2.04001352276471,
11.2602312652308));
#59433=CARTESIAN_POINT('Ctrl Pts',(1.39919924216592,1.59389993501891,11.1490981472392));
#59434=CARTESIAN_POINT('Ctrl Pts',(2.09798619095311,-0.311013608546298,
11.0379650292476));
#59435=CARTESIAN_POINT('Ctrl Pts',(0.876613601848224,-1.93127525619361,
10.9268319112561));
#59436=CARTESIAN_POINT('Ctrl Pts',(-1.14707025884331,-1.78395777511916,
10.8156987932645));
#59437=CARTESIAN_POINT('Ctrl Pts',(-2.12091027039602,-0.00389192236186189,
10.704565675273));
#59438=CARTESIAN_POINT('Ctrl Pts',(-1.15360972426749,1.77973597092559,10.5934325572814));
#59439=CARTESIAN_POINT('Ctrl Pts',(0.869519847146903,1.93447945389672,10.4822994392899));
#59440=CARTESIAN_POINT('Ctrl Pts',(2.09683063048482,0.318711200292248,10.3711663212983));
#59441=CARTESIAN_POINT('Ctrl Pts',(1.40503949035355,-1.58875408817032,10.2600332033067));
#59442=CARTESIAN_POINT('Ctrl Pts',(-0.572699093164549,-2.04212910238781,
10.1489000853151));
#59443=CARTESIAN_POINT('Ctrl Pts',(-2.02628092540217,-0.62646718468185,
10.0377669673236));
#59444=CARTESIAN_POINT('Ctrl Pts',(-1.62533070107094,1.36256215795326,9.926633849332));
#59445=CARTESIAN_POINT('Ctrl Pts',(0.263186153272049,2.1045209837052,9.81550073134043));
#59446=CARTESIAN_POINT('Ctrl Pts',(1.91082468123702,0.92033937203218,9.70436761334888));
#59447=CARTESIAN_POINT('Ctrl Pts',(1.80960125160234,-1.10617305713086,9.59323449535732));
#59448=CARTESIAN_POINT('Ctrl Pts',(0.0521595312995029,-2.12027236585766,
9.48210137736577));
#59449=CARTESIAN_POINT('Ctrl Pts',(-1.75302064504595,-1.19381495224981,
9.3709682593742));
#59450=CARTESIAN_POINT('Ctrl Pts',(-1.95376732879043,0.825268893765985,
9.25983514138264));
#59451=CARTESIAN_POINT('Ctrl Pts',(-0.36634925375944,2.0890341659204,9.14870202339108));
#59452=CARTESIAN_POINT('Ctrl Pts',(1.55636607780483,1.44083314587839,9.03756890539953));
#59453=CARTESIAN_POINT('Ctrl Pts',(2.05463391674853,-0.52607507998306,8.92643578740797));
#59454=CARTESIAN_POINT('Ctrl Pts',(0.672419925942791,-2.01149868639398,
8.8153026694164));
#59455=CARTESIAN_POINT('Ctrl Pts',(-1.32521924815821,-1.65591952346139,
8.70416955142485));
#59456=CARTESIAN_POINT('Ctrl Pts',(-2.10996560453856,0.215222364199064,
8.59303643343329));
#59457=CARTESIAN_POINT('Ctrl Pts',(-0.963588395426978,1.88938427212225,
8.48190331544173));
#59458=CARTESIAN_POINT('Ctrl Pts',(1.06470284579765,1.83430733057853,8.37077019745017));
#59459=CARTESIAN_POINT('Ctrl Pts',(2.11853612450705,0.100400118980249,8.2596370794586));
#59460=CARTESIAN_POINT('Ctrl Pts',(1.23340177973559,-1.72539722657859,8.14850396146706));
#59461=CARTESIAN_POINT('Ctrl Pts',(-0.780590462932345,-1.97204313208455,
8.03737084347548));
#59462=CARTESIAN_POINT('Ctrl Pts',(-2.08015550830599,-0.413797520013708,
7.92623772548394));
#59463=CARTESIAN_POINT('Ctrl Pts',(-1.47588051476366,1.52317182299603,7.81510460749237));
#59464=CARTESIAN_POINT('Ctrl Pts',(0.479178714765514,2.06607445056659,7.70397148950082));
#59465=CARTESIAN_POINT('Ctrl Pts',(1.9956741534898,0.718024252163197,7.59283837150925));
#59466=CARTESIAN_POINT('Ctrl Pts',(1.6856511482838,-1.28718968029966,7.4817052535177));
#59467=CARTESIAN_POINT('Ctrl Pts',(-0.167148217215834,-2.11431757046793,
7.37057213552614));
#59468=CARTESIAN_POINT('Ctrl Pts',(-1.86696297669774,-1.00633762390452,
7.25943901753458));
#59469=CARTESIAN_POINT('Ctrl Pts',(-1.85806733744734,1.0226798757451,7.14830589954301));
#59470=CARTESIAN_POINT('Ctrl Pts',(-0.14858081909429,2.11570479775745,7.03717278155147));
#59471=CARTESIAN_POINT('Ctrl Pts',(1.69686497753106,1.27234520719057,6.9260396635599));
#59472=CARTESIAN_POINT('Ctrl Pts',(1.98932614125418,-0.735499115767105,
6.81490654556834));
#59473=CARTESIAN_POINT('Ctrl Pts',(0.460976509621175,-2.0702156528929,6.70377342757679));
#59474=CARTESIAN_POINT('Ctrl Pts',(-1.48908362092749,-1.51013211928057,
6.59264030958522));
#59475=CARTESIAN_POINT('Ctrl Pts',(-2.07664519172384,0.431974439389764,
6.48150719159367));
#59476=CARTESIAN_POINT('Ctrl Pts',(-0.762873426914959,1.97892999787455,
6.3703740736021));
#59477=CARTESIAN_POINT('Ctrl Pts',(1.24775894853773,1.71429024289899,6.25924095561055));
#59478=CARTESIAN_POINT('Ctrl Pts',(2.11899801061436,-0.118557379976997,
6.14810783761898));
#59479=CARTESIAN_POINT('Ctrl Pts',(1.04553868001519,-1.84469146870582,6.03696198616902));
#59480=CARTESIAN_POINT('Ctrl Pts',(-0.300587145776539,-1.86708504092665,
5.9628605073829));
#59481=CARTESIAN_POINT('Ctrl Pts',(-0.829805936047086,-1.59105591793132,
5.92580340126064));
#59482=CARTESIAN_POINT('Ctrl Pts',(-0.429098066978468,-1.60671882000083,
17.2261593459789));
#59483=CARTESIAN_POINT('Ctrl Pts',(-0.963347356900843,-1.46403963137329,
17.189114973315));
#59484=CARTESIAN_POINT('Ctrl Pts',(-1.86910334049824,-0.606355572414101,
17.1150262279873));
#59485=CARTESIAN_POINT('Ctrl Pts',(-1.52260375854332,1.24511671666685,17.0038931099958));
#59486=CARTESIAN_POINT('Ctrl Pts',(0.219987328276866,1.95267251326906,16.8927599920042));
#59487=CARTESIAN_POINT('Ctrl Pts',(1.75994382100308,0.875227564391478,16.7816268740126));
#59488=CARTESIAN_POINT('Ctrl Pts',(1.68980326423006,-1.00437960527311,16.6704937560211));
#59489=CARTESIAN_POINT('Ctrl Pts',(0.0727365363976771,-1.96415437012253,
16.5593606380295));
#59490=CARTESIAN_POINT('Ctrl Pts',(-1.61071747130897,-1.12656364976777,
16.448227520038));
#59491=CARTESIAN_POINT('Ctrl Pts',(-1.82007579882138,0.742262581415753,
16.3370944020464));
#59492=CARTESIAN_POINT('Ctrl Pts',(-0.363578682501955,1.93165706602509,
16.2259612840548));
#59493=CARTESIAN_POINT('Ctrl Pts',(1.42565355239802,1.3531668510839,16.1148281660633));
#59494=CARTESIAN_POINT('Ctrl Pts',(1.91008536395604,-0.46381789473709,16.0036950480717));
#59495=CARTESIAN_POINT('Ctrl Pts',(0.646324635131519,-1.85628622389334,
15.8925619300802));
#59496=CARTESIAN_POINT('Ctrl Pts',(-1.20897405141744,-1.54981463244357,
15.7814288120886));
#59497=CARTESIAN_POINT('Ctrl Pts',(-1.95777408401628,0.17511160564734,15.6702956940971));
#59498=CARTESIAN_POINT('Ctrl Pts',(-0.914741179794969,1.73976708508744,
15.5591625761055));
#59499=CARTESIAN_POINT('Ctrl Pts',(0.965498312717399,1.71212015461434,15.4480294581139));
#59500=CARTESIAN_POINT('Ctrl Pts',(1.96207603220635,0.117472997579524,15.3368963401224));
#59501=CARTESIAN_POINT('Ctrl Pts',(1.16288439157133,-1.5846898230992,15.2257632221308));
#59502=CARTESIAN_POINT('Ctrl Pts',(-0.700624736972627,-1.83648227442104,
15.1146301041392));
#59503=CARTESIAN_POINT('Ctrl Pts',(-1.92289457071904,-0.407453797149452,
15.0034969861477));
#59504=CARTESIAN_POINT('Ctrl Pts',(-1.38525558759209,1.3944923970035,14.8923638681561));
#59505=CARTESIAN_POINT('Ctrl Pts',(0.420223821246926,1.92014428131401,14.7812307501646));
#59506=CARTESIAN_POINT('Ctrl Pts',(1.84109785488531,0.688404533496607,14.670097632173));
#59507=CARTESIAN_POINT('Ctrl Pts',(1.57692666376329,-1.17339013362344,14.5589645141814));
#59508=CARTESIAN_POINT('Ctrl Pts',(-0.130509875659643,-1.9612519689312,
14.4478313961899));
#59509=CARTESIAN_POINT('Ctrl Pts',(-1.71849864089984,-0.954098806752508,
14.3366982781983));
#59510=CARTESIAN_POINT('Ctrl Pts',(-1.73364981010159,0.926283135598728,
14.2255651602068));
#59511=CARTESIAN_POINT('Ctrl Pts',(-0.162096437536863,1.95889429448345,
14.1144320422152));
#59512=CARTESIAN_POINT('Ctrl Pts',(1.55781397483566,1.19864829352863,14.0032989242236));
#59513=CARTESIAN_POINT('Ctrl Pts',(1.85195172241498,-0.658647803895892,
13.8921658062321));
#59514=CARTESIAN_POINT('Ctrl Pts',(0.451110361563619,-1.91312350712482,
13.7810326882405));
#59515=CARTESIAN_POINT('Ctrl Pts',(-1.36260495773885,-1.41663327679692,
13.669899570249));
#59516=CARTESIAN_POINT('Ctrl Pts',(-1.92921058810115,0.376415486582924,
13.5587664522574));
#59517=CARTESIAN_POINT('Ctrl Pts',(-0.730126755249216,1.82495398108075,
13.4476333342658));
#59518=CARTESIAN_POINT('Ctrl Pts',(1.13719782151834,1.60322276260062,13.3365002162743));
#59519=CARTESIAN_POINT('Ctrl Pts',(1.96371419236092,-0.0858410304424767,
13.2253670982827));
#59520=CARTESIAN_POINT('Ctrl Pts',(0.992962043318029,-1.69633973375572,
13.1142339802912));
#59521=CARTESIAN_POINT('Ctrl Pts',(-0.886588050375063,-1.75428154545383,
13.0031008622996));
#59522=CARTESIAN_POINT('Ctrl Pts',(-1.95469786459909,-0.206635838904127,
12.8919677443081));
#59523=CARTESIAN_POINT('Ctrl Pts',(-1.23379125698389,1.53013112051816,12.7808346263165));
#59524=CARTESIAN_POINT('Ctrl Pts',(0.616329670573675,1.86646185306811,12.6697015083249));
#59525=CARTESIAN_POINT('Ctrl Pts',(1.90236142512275,0.49453323446751,12.5585683903334));
#59526=CARTESIAN_POINT('Ctrl Pts',(1.44727712718345,-1.33001166495622,12.4474352723418));
#59527=CARTESIAN_POINT('Ctrl Pts',(-0.332412161826789,-1.93727753986298,
12.3363021543503));
#59528=CARTESIAN_POINT('Ctrl Pts',(-1.80786475671794,-0.77147075978622,
12.2251690363587));
#59529=CARTESIAN_POINT('Ctrl Pts',(-1.62868836939741,1.10041642444011,12.1140359183672));
#59530=CARTESIAN_POINT('Ctrl Pts',(0.0411277181451806,1.96515918505044,
12.0029028003756));
#59531=CARTESIAN_POINT('Ctrl Pts',(1.67330209927009,1.03131091159081,11.891769682384));
#59532=CARTESIAN_POINT('Ctrl Pts',(1.77400453861417,-0.846433700158669,
11.7806365643925));
#59533=CARTESIAN_POINT('Ctrl Pts',(0.25106820008033,-1.94948887421713,11.6695034464009));
#59534=CARTESIAN_POINT('Ctrl Pts',(-1.50165563711509,-1.26829509945771,
11.5583703284093));
#59535=CARTESIAN_POINT('Ctrl Pts',(-1.88000513063285,0.573692269934076,
11.4472372104178));
#59536=CARTESIAN_POINT('Ctrl Pts',(-0.537699932314552,1.89061389357449,
11.3361040924262));
#59537=CARTESIAN_POINT('Ctrl Pts',(1.29672940772112,1.47717126797781,11.2249709744347));
#59538=CARTESIAN_POINT('Ctrl Pts',(1.94434095503829,-0.288236642966698,
11.1138378564431));
#59539=CARTESIAN_POINT('Ctrl Pts',(0.81241513179017,-1.78983903338438,11.0027047384516));
#59540=CARTESIAN_POINT('Ctrl Pts',(-1.0630649964203,-1.65331029307079,10.89157162046));
#59541=CARTESIAN_POINT('Ctrl Pts',(-1.9655861980764,-0.00360689887980824,
10.7804385024684));
#59542=CARTESIAN_POINT('Ctrl Pts',(-1.0691255465341,1.64939767113214,10.6693053844769));
#59543=CARTESIAN_POINT('Ctrl Pts',(0.80584088556765,1.79280857286422,10.5581722664853));
#59544=CARTESIAN_POINT('Ctrl Pts',(1.94327002160974,0.295370504453181,10.4470391484938));
#59545=CARTESIAN_POINT('Ctrl Pts',(1.30214194751179,-1.47240227530321,10.3359060305022));
#59546=CARTESIAN_POINT('Ctrl Pts',(-0.530757688756401,-1.89257453951323,
10.2247729125106));
#59547=CARTESIAN_POINT('Ctrl Pts',(-1.87788699785602,-0.580588094152845,
10.1136397945191));
#59548=CARTESIAN_POINT('Ctrl Pts',(-1.50630021360515,1.26277542670112,10.0025066765275));
#59549=CARTESIAN_POINT('Ctrl Pts',(0.243911813534555,1.95039717468138,9.89137355853593));
#59550=CARTESIAN_POINT('Ctrl Pts',(1.77088614865442,0.852938661509229,9.78024044054438));
#59551=CARTESIAN_POINT('Ctrl Pts',(1.67707577912157,-1.02516288601611,9.66910732255282));
#59552=CARTESIAN_POINT('Ctrl Pts',(0.0483396474860255,-1.9649950102389,
9.55797420456127));
#59553=CARTESIAN_POINT('Ctrl Pts',(-1.62463883217554,-1.10638635964609,
9.44684108656969));
#59554=CARTESIAN_POINT('Ctrl Pts',(-1.8106839074366,0.76483063424711,9.33570796857815));
#59555=CARTESIAN_POINT('Ctrl Pts',(-0.339519802848938,1.93604452821876,
9.22457485058658));
#59556=CARTESIAN_POINT('Ctrl Pts',(1.44238618879254,1.33531426802924,9.11344173259502));
#59557=CARTESIAN_POINT('Ctrl Pts',(1.90416356845991,-0.487548167784373,
9.00230861460347));
#59558=CARTESIAN_POINT('Ctrl Pts',(0.62317550355297,-1.8641873306062,8.8911754966119));
#59559=CARTESIAN_POINT('Ctrl Pts',(-1.22816731097189,-1.53464887500082,
8.78004237862035));
#59560=CARTESIAN_POINT('Ctrl Pts',(-1.95544306073944,0.19946063465856,8.66890926062879));
#59561=CARTESIAN_POINT('Ctrl Pts',(-0.893020358812349,1.75101591990155,
8.55777614263723));
#59562=CARTESIAN_POINT('Ctrl Pts',(0.986729730136937,1.69997251762203,8.44664302464568));
#59563=CARTESIAN_POINT('Ctrl Pts',(1.96338592187579,0.0930473537270221,
8.33550990665409));
#59564=CARTESIAN_POINT('Ctrl Pts',(1.1430740605912,-1.59903840445307,8.22437678866256));
#59565=CARTESIAN_POINT('Ctrl Pts',(-0.723424211625604,-1.82762128909535,
8.11324367067098));
#59566=CARTESIAN_POINT('Ctrl Pts',(-1.92781609578202,-0.383493213027498,
8.00211055267944));
#59567=CARTESIAN_POINT('Ctrl Pts',(-1.36779495593073,1.41162290284956,7.89097743468786));
#59568=CARTESIAN_POINT('Ctrl Pts',(0.444086240376034,1.91476625905239,7.77984431669632));
#59569=CARTESIAN_POINT('Ctrl Pts',(1.84952170146496,0.665440013958054,7.66871119870474));
#59570=CARTESIAN_POINT('Ctrl Pts',(1.56220311537253,-1.19292282432625,7.5575780807132));
#59571=CARTESIAN_POINT('Ctrl Pts',(-0.154907179892704,-1.95947631206774,
7.44644496272163));
#59572=CARTESIAN_POINT('Ctrl Pts',(-1.73023663968183,-0.932638863492504,
7.33531184473009));
#59573=CARTESIAN_POINT('Ctrl Pts',(-1.72199246925288,0.947784296617001,
7.22417872673851));
#59574=CARTESIAN_POINT('Ctrl Pts',(-0.13769955824491,1.9607619462843,7.11304560874695));
#59575=CARTESIAN_POINT('Ctrl Pts',(1.57259570401887,1.17916548066668,7.00191249075541));
#59576=CARTESIAN_POINT('Ctrl Pts',(1.84363858353691,-0.681635112445974,
6.89077937276383));
#59577=CARTESIAN_POINT('Ctrl Pts',(0.427217066934015,-1.91860418197146,
6.77964625477228));
#59578=CARTESIAN_POINT('Ctrl Pts',(-1.38003113754085,-1.39953815697045,
6.66851313678072));
#59579=CARTESIAN_POINT('Ctrl Pts',(-1.92456285592503,0.400338952495038,
6.55738001878916));
#59580=CARTESIAN_POINT('Ctrl Pts',(-0.707004676130548,1.83400379783878,
6.44624690079761));
#59581=CARTESIAN_POINT('Ctrl Pts',(1.15637978749291,1.58874483657911,6.33511378280605));
#59582=CARTESIAN_POINT('Ctrl Pts',(1.96381398192635,-0.109874874489327,
6.22398066481448));
#59583=CARTESIAN_POINT('Ctrl Pts',(0.968969044885222,-1.70959617726799,
6.11283481336452));
#59584=CARTESIAN_POINT('Ctrl Pts',(-0.278573758307664,-1.7303497645825,
6.0387333345784));
#59585=CARTESIAN_POINT('Ctrl Pts',(-0.769035407929571,-1.47453553142049,
6.00167622845614));
#59586=CARTESIAN_POINT('Ctrl Pts',(-0.530170217188721,-1.98517432567169,
17.));
#59587=CARTESIAN_POINT('Ctrl Pts',(-0.59958638778647,-1.95947209126774,
17.));
#59588=CARTESIAN_POINT('Ctrl Pts',(-0.667262296603072,-1.92979787875034,
17.));
#59589=CARTESIAN_POINT('Ctrl Pts',(-0.733002470738773,-1.89645448736446,
17.));
#59590=CARTESIAN_POINT('Ctrl Pts',(-0.799702571694335,-1.86262422145966,
17.));
#59591=CARTESIAN_POINT('Ctrl Pts',(-0.864410706066083,-1.82501605153519,
17.));
#59592=CARTESIAN_POINT('Ctrl Pts',(-0.926891494234642,-1.78390179589663,
17.));
#59593=CARTESIAN_POINT('Ctrl Pts',(-0.977240315226614,-1.75077074300754,
17.));
#59594=CARTESIAN_POINT('Ctrl Pts',(-1.0261423231337,-1.71536194678685,17.));
#59595=CARTESIAN_POINT('Ctrl Pts',(-1.0734552151732,-1.6778024578881,17.));
#59596=CARTESIAN_POINT('Ctrl Pts',(-1.09711166119295,-1.65902271343873,
17.));
#59597=CARTESIAN_POINT('Ctrl Pts',(-1.12037053740919,-1.63970511721008,
17.));
#59598=CARTESIAN_POINT('Ctrl Pts',(-1.14321217455345,-1.61986466499212,
17.));
#59599=CARTESIAN_POINT('Ctrl Pts',(-1.15783918687559,-1.60715951004916,
17.));
#59600=CARTESIAN_POINT('Ctrl Pts',(-1.17229538706437,-1.59423965238433,
17.));
#59601=CARTESIAN_POINT('Ctrl Pts',(-1.18657442194043,-1.58110975612116,
17.));
#59602=CARTESIAN_POINT('Ctrl Pts',(-1.19459362037587,-1.57373592137077,
17.));
#59603=CARTESIAN_POINT('Ctrl Pts',(-1.20255571179842,-1.56629689983921,
17.));
#59604=CARTESIAN_POINT('Ctrl Pts',(-1.21045281961469,-1.55880022777578,
17.));
#59605=CARTESIAN_POINT('Ctrl Pts',(-1.26354014875506,-1.50840477838492,
17.));
#59606=CARTESIAN_POINT('Ctrl Pts',(-1.31378747767688,-1.45532141233497,
17.));
#59607=CARTESIAN_POINT('Ctrl Pts',(-1.36097600959484,-1.3998088981192,17.));
#59608=CARTESIAN_POINT('Ctrl Pts',(-1.40742908231333,-1.34516157694095,
17.));
#59609=CARTESIAN_POINT('Ctrl Pts',(-1.45091839778076,-1.28815934728008,
17.));
#59610=CARTESIAN_POINT('Ctrl Pts',(-1.49119167764656,-1.22902545012624,
17.));
#59611=CARTESIAN_POINT('Ctrl Pts',(-1.52524153022102,-1.17902951021394,
17.));
#59612=CARTESIAN_POINT('Ctrl Pts',(-1.55699193038151,-1.12750916897208,
17.));
#59613=CARTESIAN_POINT('Ctrl Pts',(-1.58626203451582,-1.07459264749954,
17.));
#59614=CARTESIAN_POINT('Ctrl Pts',(-1.59836979258552,-1.05270340388976,
17.));
#59615=CARTESIAN_POINT('Ctrl Pts',(-1.61005281462832,-1.03057521758956,
17.));
#59616=CARTESIAN_POINT('Ctrl Pts',(-1.62129684910972,-1.00821707885185,
17.));
#59617=CARTESIAN_POINT('Ctrl Pts',(-1.62649913652706,-0.997872618949778,
17.));
#59618=CARTESIAN_POINT('Ctrl Pts',(-1.63160743994957,-0.987478934463243,
17.));
#59619=CARTESIAN_POINT('Ctrl Pts',(-1.63662028259746,-0.977036917721011,
17.));
#59620=CARTESIAN_POINT('Ctrl Pts',(-1.64185147465901,-0.966140067585173,
17.));
#59621=CARTESIAN_POINT('Ctrl Pts',(-1.64697509598823,-0.955198041348551,
17.));
#59622=CARTESIAN_POINT('Ctrl Pts',(-1.65198809526169,-0.94421612686998,
17.));
#59623=CARTESIAN_POINT('Ctrl Pts',(-1.68052781084573,-0.881694530777598,
17.));
#59624=CARTESIAN_POINT('Ctrl Pts',(-1.70550660071472,-0.817838180873781,
17.));
#59625=CARTESIAN_POINT('Ctrl Pts',(-1.72670093437665,-0.752850869832327,
17.));
#59626=CARTESIAN_POINT('Ctrl Pts',(-1.74590469391102,-0.693967174127041,
17.));
#59627=CARTESIAN_POINT('Ctrl Pts',(-1.76200116624391,-0.634154383630976,
17.));
#59628=CARTESIAN_POINT('Ctrl Pts',(-1.77478736554882,-0.573559243480358,
17.));
#59629=CARTESIAN_POINT('Ctrl Pts',(-1.78927486034487,-0.504901485481765,
17.));
#59630=CARTESIAN_POINT('Ctrl Pts',(-1.799512747065,-0.435238075154566,17.));
#59631=CARTESIAN_POINT('Ctrl Pts',(-1.80556817728997,-0.364940578178376,
17.));
#59632=CARTESIAN_POINT('Ctrl Pts',(-1.80722934559513,-0.345656073267864,
17.));
#59633=CARTESIAN_POINT('Ctrl Pts',(-1.80857547625591,-0.326323949543816,
17.));
#59634=CARTESIAN_POINT('Ctrl Pts',(-1.80960732651783,-0.30695215324635,
17.));
#59635=CARTESIAN_POINT('Ctrl Pts',(-1.81050226718635,-0.290150676356872,
17.));
#59636=CARTESIAN_POINT('Ctrl Pts',(-1.81116079923754,-0.273313162210314,
17.));
#59637=CARTESIAN_POINT('Ctrl Pts',(-1.81158284306408,-0.256479086675087,
17.));
#59638=CARTESIAN_POINT('Ctrl Pts',(-1.81330048651302,-0.187967387785159,
17.));
#59639=CARTESIAN_POINT('Ctrl Pts',(-1.81111278941556,-0.11942609791947,
17.));
#59640=CARTESIAN_POINT('Ctrl Pts',(-1.80514016974053,-0.05119331079533,
17.));
#59641=CARTESIAN_POINT('Ctrl Pts',(-1.79915254414877,0.0172109078911375,
17.));
#59642=CARTESIAN_POINT('Ctrl Pts',(-1.78936051943155,0.085306157363821,
17.));
#59643=CARTESIAN_POINT('Ctrl Pts',(-1.77583551231836,0.152736676162679,
17.));
#59644=CARTESIAN_POINT('Ctrl Pts',(-1.76259194094567,0.218764063870252,
17.));
#59645=CARTESIAN_POINT('Ctrl Pts',(-1.74576857726395,0.284154971652147,
17.));
#59646=CARTESIAN_POINT('Ctrl Pts',(-1.72539221768325,0.348546576029075,
17.));
#59647=CARTESIAN_POINT('Ctrl Pts',(-1.71949214477078,0.367191474754506,
17.));
#59648=CARTESIAN_POINT('Ctrl Pts',(-1.71329394772695,0.385752356812901,
17.));
#59649=CARTESIAN_POINT('Ctrl Pts',(-1.70679772648935,0.404219792736258,
17.));
#59650=CARTESIAN_POINT('Ctrl Pts',(-1.70266287321327,0.415974339746853,
17.));
#59651=CARTESIAN_POINT('Ctrl Pts',(-1.698410480872,0.427681900514319,17.));
#59652=CARTESIAN_POINT('Ctrl Pts',(-1.69404123115752,0.439339805259342,
17.));
#59653=CARTESIAN_POINT('Ctrl Pts',(-1.67085891425587,0.501194187560434,
17.));
#59654=CARTESIAN_POINT('Ctrl Pts',(-1.64438824791585,0.561658220290148,
17.));
#59655=CARTESIAN_POINT('Ctrl Pts',(-1.6146796577165,0.62039476474356,17.));
#59656=CARTESIAN_POINT('Ctrl Pts',(-1.59391160861621,0.661455058450027,
17.));
#59657=CARTESIAN_POINT('Ctrl Pts',(-1.5715603802492,0.70167061883402,17.));
#59658=CARTESIAN_POINT('Ctrl Pts',(-1.54763291644676,0.740915041686162,
17.));
#59659=CARTESIAN_POINT('Ctrl Pts',(-1.53991882725148,0.753567238375207,
17.));
#59660=CARTESIAN_POINT('Ctrl Pts',(-1.53203975915063,0.766120089974338,
17.));
#59661=CARTESIAN_POINT('Ctrl Pts',(-1.52399923812354,0.778563773820041,
17.));
#59662=CARTESIAN_POINT('Ctrl Pts',(-1.48975784779894,0.83155648837186,17.));
#59663=CARTESIAN_POINT('Ctrl Pts',(-1.45266161665523,0.88246473729788,17.));
#59664=CARTESIAN_POINT('Ctrl Pts',(-1.41274488079971,0.930972884647871,
17.));
#59665=CARTESIAN_POINT('Ctrl Pts',(-1.37594347516523,0.975695178917259,
17.));
#59666=CARTESIAN_POINT('Ctrl Pts',(-1.33674405604559,1.01837748510076,17.));
#59667=CARTESIAN_POINT('Ctrl Pts',(-1.29515206733999,1.05873948677329,17.));
#59668=CARTESIAN_POINT('Ctrl Pts',(-1.28733353636727,1.06632680274491,17.));
#59669=CARTESIAN_POINT('Ctrl Pts',(-1.2794304058483,1.07383202241508,17.));
#59670=CARTESIAN_POINT('Ctrl Pts',(-1.27144426759649,1.08125448192165,17.));
#59671=CARTESIAN_POINT('Origin',(0.,0.,5.));
#59672=CARTESIAN_POINT('Origin',(0.,0.,0.));
#59673=CARTESIAN_POINT('',(-5.,-6.12323399573677E-16,17.));
#59674=CARTESIAN_POINT('Origin',(0.,0.,17.));
#59675=CARTESIAN_POINT('',(-5.,-6.12323399573677E-16,0.));
#59676=CARTESIAN_POINT('',(-5.,-6.12323399573677E-16,0.));
#59677=CARTESIAN_POINT('Origin',(0.,0.,0.));
#59678=CARTESIAN_POINT('Origin',(0.,0.,17.));
#59679=CARTESIAN_POINT('Origin',(0.,0.,0.));
#94385=UNCERTAINTY_MEASURE_WITH_UNIT(LENGTH_MEASURE(0.01),#94413,
'DISTANCE_ACCURACY_VALUE',
'Maximum model space distance between geometric entities at asserted c
onnectivities');
#94394=UNCERTAINTY_MEASURE_WITH_UNIT(LENGTH_MEASURE(0.01),#94413,
'DISTANCE_ACCURACY_VALUE',
'Maximum model space distance between geometric entities at asserted c
onnectivities');
#94403=(
GEOMETRIC_REPRESENTATION_CONTEXT(3)
GLOBAL_UNCERTAINTY_ASSIGNED_CONTEXT((#94385))
GLOBAL_UNIT_ASSIGNED_CONTEXT((#94413,#94415,#94416))
REPRESENTATION_CONTEXT('','3D')
);
#94412=(
GEOMETRIC_REPRESENTATION_CONTEXT(3)
GLOBAL_UNCERTAINTY_ASSIGNED_CONTEXT((#94394))
GLOBAL_UNIT_ASSIGNED_CONTEXT((#94413,#94415,#94416))
REPRESENTATION_CONTEXT('','3D')
);
#94413=(
LENGTH_UNIT()
NAMED_UNIT(*)
SI_UNIT(.MILLI.,.METRE.)
);
#94415=(
NAMED_UNIT(*)
PLANE_ANGLE_UNIT()
SI_UNIT($,.RADIAN.)
);
#94416=(
NAMED_UNIT(*)
SI_UNIT($,.STERADIAN.)
SOLID_ANGLE_UNIT()
);
#94425=SHAPE_DEFINITION_REPRESENTATION(#94442,#94494);
#94442=PRODUCT_DEFINITION_SHAPE('',$,#94512);
#94494=SHAPE_REPRESENTATION('',(#8647),#94403);
#94503=PRODUCT_DEFINITION_CONTEXT('part definition',#94556,'design');
#94512=PRODUCT_DEFINITION('Tray pillar','Tray pillar',#94529,#94503);
#94529=PRODUCT_DEFINITION_FORMATION('',$,#94566);
#94556=APPLICATION_CONTEXT(
'Core Data for Automotive Mechanical Design Process');
#94557=PRODUCT_CONTEXT('part definition',#94556,'mechanical');
#94566=PRODUCT('Tray pillar','Tray pillar',
'Steel tray boss welded to the base panel.',(#94557));
#94577=PRESENTATION_STYLE_ASSIGNMENT((#94584));
#94584=SURFACE_STYLE_USAGE(.BOTH.,#94591);
#94591=SURFACE_SIDE_STYLE('',(#94598));
#94598=SURFACE_STYLE_FILL_AREA(#94605);
#94605=FILL_AREA_STYLE('Opaque(104,114,127)',(#94612));
#94612=FILL_AREA_STYLE_COLOUR('Opaque(104,114,127)',#94619);
#94619=COLOUR_RGB('Opaque(104,114,127)',0.407843137254902,0.447058823529412,
0.498039215686275);
ENDSEC;
END-ISO-10303-21;
